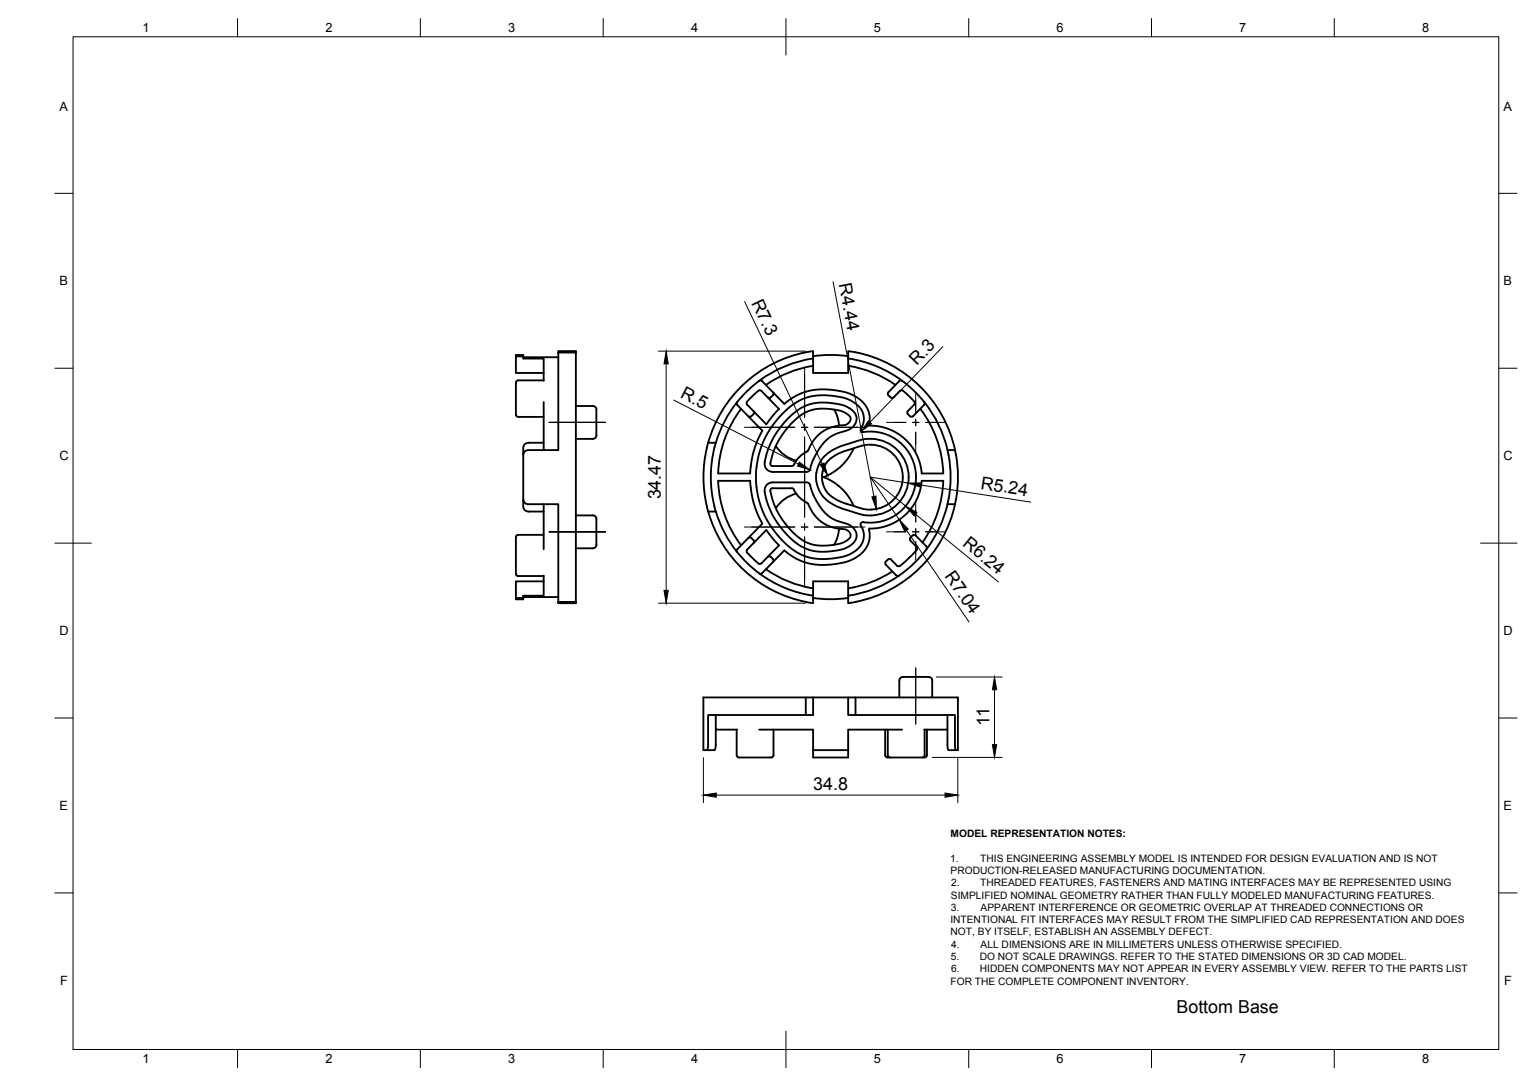
ISO-10303-21;
HEADER;
/* Generated by software containing ST-Developer
 * from STEP Tools, Inc. (www.steptools.com) 
 */

FILE_DESCRIPTION(
/* description */ ('STEP AP214'),
/* implementation_level */ '2;1');

FILE_NAME(
/* name */ 'Bottom Base.step',
/* time_stamp */ '2026-10-06T00:19:40-07:00',
/* author */ (''),
/* organization */ (''),
/* preprocessor_version */ 'ST-DEVELOPER v20.2',
/* originating_system */ 'Autodesk Translation Framework v15.15.0.0',
/* authorisation */ '');

FILE_SCHEMA (('AUTOMOTIVE_DESIGN { 1 0 10303 214 3 1 1 }'));
ENDSEC;

DATA;
#10=MECHANICAL_DESIGN_GEOMETRIC_PRESENTATION_REPRESENTATION('',(#2067),#98302);
#63=ORIENTED_CLOSED_SHELL('',*,#34171,.F.);
#64=ORIENTED_CLOSED_SHELL('',*,#34172,.F.);
#65=BREP_WITH_VOIDS('Body1',#34173,(#63,#64));
#120=TOROIDAL_SURFACE('',#35179,1.75,0.5);
#121=TOROIDAL_SURFACE('',#35197,1.75,0.5);
#122=TOROIDAL_SURFACE('',#35509,16.1,0.3);
#123=TOROIDAL_SURFACE('',#35537,0.6,0.3);
#124=TOROIDAL_SURFACE('',#35540,15.7,0.3);
#125=TOROIDAL_SURFACE('',#35542,0.6,0.3);
#126=TOROIDAL_SURFACE('',#35565,16.1,0.3);
#127=TOROIDAL_SURFACE('',#35593,0.6,0.3);
#128=TOROIDAL_SURFACE('',#35596,15.7,0.3);
#129=TOROIDAL_SURFACE('',#35598,0.6,0.3);
#130=TOROIDAL_SURFACE('',#35623,16.1,0.3);
#131=TOROIDAL_SURFACE('',#35651,0.6,0.3);
#132=TOROIDAL_SURFACE('',#35654,15.7,0.3);
#133=TOROIDAL_SURFACE('',#35656,0.6,0.3);
#134=TOROIDAL_SURFACE('',#35689,16.1,0.3);
#135=TOROIDAL_SURFACE('',#35706,0.6,0.3);
#136=TOROIDAL_SURFACE('',#35709,15.7,0.3);
#137=TOROIDAL_SURFACE('',#35711,0.6,0.3);
#587=ELLIPSE('',#35016,13.361638124116,11.5578357668316);
#588=ELLIPSE('',#35018,0.952789221356583,0.825051280209737);
#589=ELLIPSE('',#35164,8.5034308409691,7.3551645679647);
#590=ELLIPSE('',#35170,0.95278921998829,0.825051277838727);
#591=ELLIPSE('',#35172,13.3616381240247,11.5578357666725);
#592=ELLIPSE('',#35175,13.3641581201969,11.5586227277888);
#593=ELLIPSE('',#35177,13.3735436793885,11.5615411739172);
#594=ELLIPSE('',#35193,13.3735436794947,11.5615411741025);
#595=ELLIPSE('',#35195,13.3641581202021,11.5586227277978);
#596=ELLIPSE('',#35373,5.47251735374185,5.45746583056251);
#597=ELLIPSE('',#35374,5.47484463449433,5.45859738058976);
#598=ELLIPSE('',#35383,1586.78234781094,77.5099567232996);
#599=ELLIPSE('',#35385,1.14101622851481,0.979516364167449);
#600=ELLIPSE('',#35388,3.21318791213204,0.733552647206039);
#601=ELLIPSE('',#35393,9.5906032530047,5.82945480771065);
#602=ELLIPSE('',#35396,9.59060325044611,5.82945480684165);
#603=ELLIPSE('',#35401,1586.78234781094,77.5099567232996);
#604=ELLIPSE('',#35402,1.14101622838842,0.979516363971379);
#605=ELLIPSE('',#35405,3.21319255571472,0.733554698090194);
#712=SPHERICAL_SURFACE('',#35503,0.3);
#713=SPHERICAL_SURFACE('',#35507,0.3);
#714=SPHERICAL_SURFACE('',#35514,0.3);
#715=SPHERICAL_SURFACE('',#35522,0.3);
#716=SPHERICAL_SURFACE('',#35527,0.3);
#717=SPHERICAL_SURFACE('',#35532,0.3);
#718=SPHERICAL_SURFACE('',#35559,0.3);
#719=SPHERICAL_SURFACE('',#35563,0.3);
#720=SPHERICAL_SURFACE('',#35570,0.3);
#721=SPHERICAL_SURFACE('',#35578,0.3);
#722=SPHERICAL_SURFACE('',#35583,0.3);
#723=SPHERICAL_SURFACE('',#35588,0.3);
#724=SPHERICAL_SURFACE('',#35617,0.3);
#725=SPHERICAL_SURFACE('',#35621,0.3);
#726=SPHERICAL_SURFACE('',#35628,0.3);
#727=SPHERICAL_SURFACE('',#35636,0.3);
#728=SPHERICAL_SURFACE('',#35641,0.3);
#729=SPHERICAL_SURFACE('',#35646,0.3);
#730=SPHERICAL_SURFACE('',#35673,0.3);
#731=SPHERICAL_SURFACE('',#35677,0.3);
#732=SPHERICAL_SURFACE('',#35686,0.3);
#733=SPHERICAL_SURFACE('',#35691,0.3);
#734=SPHERICAL_SURFACE('',#35697,0.3);
#735=SPHERICAL_SURFACE('',#35700,0.3);
#1106=B_SPLINE_SURFACE_WITH_KNOTS('',3,1,((#74322,#74323),(#74324,#74325),
(#74326,#74327),(#74328,#74329)),.UNSPECIFIED.,.F.,.F.,.F.,(4,4),(2,2),
(1.93787056397,2.72108189072),(0.,0.18),.UNSPECIFIED.);
#1107=B_SPLINE_SURFACE_WITH_KNOTS('',3,1,((#74355,#74356),(#74357,#74358),
(#74359,#74360),(#74361,#74362)),.UNSPECIFIED.,.F.,.F.,.F.,(4,4),(2,2),
(1.93787056397,2.72108189072),(0.,0.18),.UNSPECIFIED.);
#1108=B_SPLINE_SURFACE_WITH_KNOTS('',4,1,((#74601,#74602),(#74603,#74604),
(#74605,#74606),(#74607,#74608),(#74609,#74610)),.UNSPECIFIED.,.F.,.F.,
 .F.,(5,5),(2,2),(13.4220086236,14.3963748612),(0.,0.288),.UNSPECIFIED.);
#1109=B_SPLINE_SURFACE_WITH_KNOTS('',4,1,((#74660,#74661),(#74662,#74663),
(#74664,#74665),(#74666,#74667),(#74668,#74669)),.UNSPECIFIED.,.F.,.F.,
 .F.,(5,5),(2,2),(13.4220086236,14.3963748612),(0.,0.288),.UNSPECIFIED.);
#1110=B_SPLINE_SURFACE_WITH_KNOTS('',4,1,((#74721,#74722),(#74723,#74724),
(#74725,#74726),(#74727,#74728),(#74729,#74730)),.UNSPECIFIED.,.F.,.F.,
 .F.,(5,5),(2,2),(7.90893025972,8.88329649724),(0.,0.288),.UNSPECIFIED.);
#1111=B_SPLINE_SURFACE_WITH_KNOTS('',4,1,((#74780,#74781),(#74782,#74783),
(#74784,#74785),(#74786,#74787),(#74788,#74789)),.UNSPECIFIED.,.F.,.F.,
 .F.,(5,5),(2,2),(7.90893025972,8.88329649724),(0.,0.288),.UNSPECIFIED.);
#1112=B_SPLINE_SURFACE_WITH_KNOTS('',5,1,((#75672,#75673),(#75674,#75675),
(#75676,#75677),(#75678,#75679),(#75680,#75681),(#75682,#75683),(#75684,
#75685),(#75686,#75687),(#75688,#75689),(#75690,#75691),(#75692,#75693),
(#75694,#75695)),.UNSPECIFIED.,.F.,.F.,.F.,(6,3,3,6),(2,2),(0.,3.06410506181,
5.01303018899,6.53082821197),(0.,0.180000000000001),.UNSPECIFIED.);
#1113=B_SPLINE_SURFACE_WITH_KNOTS('',5,1,((#75710,#75711),(#75712,#75713),
(#75714,#75715),(#75716,#75717),(#75718,#75719),(#75720,#75721),(#75722,
#75723),(#75724,#75725),(#75726,#75727),(#75728,#75729),(#75730,#75731),
(#75732,#75733)),.UNSPECIFIED.,.F.,.F.,.F.,(6,3,3,6),(2,2),(0.,1.23981126536,
4.14117682427,4.7101423031),(0.,0.180000000000001),.UNSPECIFIED.);
#1114=B_SPLINE_SURFACE_WITH_KNOTS('',5,1,((#75748,#75749),(#75750,#75751),
(#75752,#75753),(#75754,#75755),(#75756,#75757),(#75758,#75759),(#75760,
#75761),(#75762,#75763),(#75764,#75765),(#75766,#75767),(#75768,#75769),
(#75770,#75771)),.UNSPECIFIED.,.F.,.F.,.F.,(6,3,3,6),(2,2),(17.5092154859,
21.7374875265,29.3008927769,31.9433833551),(0.,0.180000000000001),
 .UNSPECIFIED.);
#1115=B_SPLINE_SURFACE_WITH_KNOTS('',5,1,((#75786,#75787),(#75788,#75789),
(#75790,#75791),(#75792,#75793),(#75794,#75795),(#75796,#75797),(#75798,
#75799),(#75800,#75801),(#75802,#75803)),.UNSPECIFIED.,.F.,.F.,.F.,(6,3,
6),(2,2),(10.4583103224,10.8525207074,15.6953714763),(0.,0.180000000000001),
 .UNSPECIFIED.);
#1116=B_SPLINE_SURFACE_WITH_KNOTS('',5,1,((#75836,#75837),(#75838,#75839),
(#75840,#75841),(#75842,#75843),(#75844,#75845),(#75846,#75847),(#75848,
#75849),(#75850,#75851),(#75852,#75853)),.UNSPECIFIED.,.F.,.F.,.F.,(6,3,
6),(2,2),(-1.52206773895,0.,8.40229743882),(0.,0.180000000000003),
 .UNSPECIFIED.);
#1117=B_SPLINE_SURFACE_WITH_KNOTS('',5,1,((#75877,#75878),(#75879,#75880),
(#75881,#75882),(#75883,#75884),(#75885,#75886),(#75887,#75888),(#75889,
#75890),(#75891,#75892),(#75893,#75894)),.UNSPECIFIED.,.F.,.F.,.F.,(6,3,
6),(2,2),(-1.52206773895,0.,8.40229791516),(0.,0.180000000000001),
 .UNSPECIFIED.);
#1118=B_SPLINE_SURFACE_WITH_KNOTS('',5,1,((#75906,#75907),(#75908,#75909),
(#75910,#75911),(#75912,#75913),(#75914,#75915),(#75916,#75917),(#75918,
#75919),(#75920,#75921),(#75922,#75923)),.UNSPECIFIED.,.F.,.F.,.F.,(6,3,
6),(2,2),(10.4583103224,10.8525207074,15.6953714763),(0.,0.180000000000001),
 .UNSPECIFIED.);
#1119=B_SPLINE_SURFACE_WITH_KNOTS('',5,1,((#75956,#75957),(#75958,#75959),
(#75960,#75961),(#75962,#75963),(#75964,#75965),(#75966,#75967),(#75968,
#75969),(#75970,#75971),(#75972,#75973),(#75974,#75975),(#75976,#75977),
(#75978,#75979)),.UNSPECIFIED.,.F.,.F.,.F.,(6,3,3,6),(2,2),(17.5092154859,
21.7374875265,29.3008927769,31.9433833551),(0.,0.180000000000001),
 .UNSPECIFIED.);
#1120=B_SPLINE_SURFACE_WITH_KNOTS('',5,1,((#75996,#75997),(#75998,#75999),
(#76000,#76001),(#76002,#76003),(#76004,#76005),(#76006,#76007),(#76008,
#76009),(#76010,#76011),(#76012,#76013),(#76014,#76015),(#76016,#76017),
(#76018,#76019)),.UNSPECIFIED.,.F.,.F.,.F.,(6,3,3,6),(2,2),(0.,1.23981126536,
4.14117682427,4.7101423031),(0.,0.180000000000001),.UNSPECIFIED.);
#1121=B_SPLINE_SURFACE_WITH_KNOTS('',5,1,((#76034,#76035),(#76036,#76037),
(#76038,#76039),(#76040,#76041),(#76042,#76043),(#76044,#76045),(#76046,
#76047),(#76048,#76049),(#76050,#76051),(#76052,#76053),(#76054,#76055),
(#76056,#76057)),.UNSPECIFIED.,.F.,.F.,.F.,(6,3,3,6),(2,2),(0.,3.06410506181,
5.01303018899,6.53082821197),(0.,0.180000000000001),.UNSPECIFIED.);
#1122=B_SPLINE_SURFACE_WITH_KNOTS('',5,1,((#76190,#76191),(#76192,#76193),
(#76194,#76195),(#76196,#76197),(#76198,#76199),(#76200,#76201),(#76202,
#76203),(#76204,#76205),(#76206,#76207),(#76208,#76209),(#76210,#76211),
(#76212,#76213),(#76214,#76215),(#76216,#76217),(#76218,#76219)),
 .UNSPECIFIED.,.F.,.F.,.F.,(6,3,3,3,6),(2,2),(0.,2.13949651284,3.65547289001,
4.94562974894,5.62440522293),(0.,0.120000000000001),.UNSPECIFIED.);
#1123=B_SPLINE_SURFACE_WITH_KNOTS('',5,1,((#76253,#76254),(#76255,#76256),
(#76257,#76258),(#76259,#76260),(#76261,#76262),(#76263,#76264),(#76265,
#76266),(#76267,#76268),(#76269,#76270)),.UNSPECIFIED.,.F.,.F.,.F.,(6,3,
6),(2,2),(0.,1.07297825382,3.85154891337),(0.,0.120000000000002),
 .UNSPECIFIED.);
#1124=B_SPLINE_SURFACE_WITH_KNOTS('',5,1,((#76292,#76293),(#76294,#76295),
(#76296,#76297),(#76298,#76299),(#76300,#76301),(#76302,#76303),(#76304,
#76305),(#76306,#76307),(#76308,#76309),(#76310,#76311),(#76312,#76313),
(#76314,#76315),(#76316,#76317),(#76318,#76319),(#76320,#76321),(#76322,
#76323),(#76324,#76325),(#76326,#76327)),.UNSPECIFIED.,.F.,.F.,.F.,(6,3,
3,3,3,6),(2,2),(-1.28529178055,0.,8.34825709363,17.7305069581,25.102843518,
27.4630296434),(0.,0.120000000000001),.UNSPECIFIED.);
#1125=B_SPLINE_SURFACE_WITH_KNOTS('',5,1,((#76373,#76374),(#76375,#76376),
(#76377,#76378),(#76379,#76380),(#76381,#76382),(#76383,#76384),(#76385,
#76386),(#76387,#76388),(#76389,#76390),(#76391,#76392),(#76393,#76394),
(#76395,#76396),(#76397,#76398),(#76399,#76400),(#76401,#76402),(#76403,
#76404),(#76405,#76406),(#76407,#76408)),.UNSPECIFIED.,.F.,.F.,.F.,(6,3,
3,3,3,6),(2,2),(-1.28529178055,0.,8.34825709363,17.7305069581,25.102843518,
27.4630296434),(0.,0.120000000000001),.UNSPECIFIED.);
#1126=B_SPLINE_SURFACE_WITH_KNOTS('',5,1,((#76448,#76449),(#76450,#76451),
(#76452,#76453),(#76454,#76455),(#76456,#76457),(#76458,#76459),(#76460,
#76461),(#76462,#76463),(#76464,#76465)),.UNSPECIFIED.,.F.,.F.,.F.,(6,3,
6),(2,2),(0.,1.07297825382,3.85154891337),(0.,0.120000000000001),
 .UNSPECIFIED.);
#1127=B_SPLINE_SURFACE_WITH_KNOTS('',5,1,((#76487,#76488),(#76489,#76490),
(#76491,#76492),(#76493,#76494),(#76495,#76496),(#76497,#76498),(#76499,
#76500),(#76501,#76502),(#76503,#76504),(#76505,#76506),(#76507,#76508),
(#76509,#76510),(#76511,#76512),(#76513,#76514),(#76515,#76516)),
 .UNSPECIFIED.,.F.,.F.,.F.,(6,3,3,3,6),(2,2),(0.,2.13949651284,3.65547289001,
4.94562974894,5.62440522293),(0.,0.120000000000001),.UNSPECIFIED.);
#1128=B_SPLINE_SURFACE_WITH_KNOTS('',5,1,((#76588,#76589),(#76590,#76591),
(#76592,#76593),(#76594,#76595),(#76596,#76597),(#76598,#76599)),
 .UNSPECIFIED.,.F.,.F.,.F.,(6,6),(2,2),(0.,3.5713550833),(0.,0.300000000000001),
 .UNSPECIFIED.);
#1129=B_SPLINE_SURFACE_WITH_KNOTS('',5,1,((#76666,#76667),(#76668,#76669),
(#76670,#76671),(#76672,#76673),(#76674,#76675),(#76676,#76677)),
 .UNSPECIFIED.,.F.,.F.,.F.,(6,6),(2,2),(0.,3.5713550833),(0.,0.300000000000001),
 .UNSPECIFIED.);
#1130=B_SPLINE_SURFACE_WITH_KNOTS('',5,1,((#77077,#77078),(#77079,#77080),
(#77081,#77082),(#77083,#77084),(#77085,#77086),(#77087,#77088),(#77089,
#77090),(#77091,#77092),(#77093,#77094),(#77095,#77096),(#77097,#77098),
(#77099,#77100),(#77101,#77102),(#77103,#77104),(#77105,#77106),(#77107,
#77108),(#77109,#77110),(#77111,#77112)),.UNSPECIFIED.,.F.,.F.,.F.,(6,3,
3,3,3,6),(2,2),(2.04066423734,2.62011481805,3.50908168923,4.52495007124,
5.25002578886,6.51367347233),(0.,0.300000000000002),.UNSPECIFIED.);
#1131=B_SPLINE_SURFACE_WITH_KNOTS('',5,1,((#77218,#77219),(#77220,#77221),
(#77222,#77223),(#77224,#77225),(#77226,#77227),(#77228,#77229),(#77230,
#77231),(#77232,#77233),(#77234,#77235),(#77236,#77237),(#77238,#77239),
(#77240,#77241),(#77242,#77243),(#77244,#77245),(#77246,#77247),(#77248,
#77249),(#77250,#77251),(#77252,#77253)),.UNSPECIFIED.,.F.,.F.,.F.,(6,3,
3,3,3,6),(2,2),(2.04066423734,2.62011481805,3.50908168923,4.52495007124,
5.25002578886,6.51367347233),(0.,0.300000000000002),.UNSPECIFIED.);
#1132=B_SPLINE_SURFACE_WITH_KNOTS('',5,1,((#77254,#77255),(#77256,#77257),
(#77258,#77259),(#77260,#77261),(#77262,#77263),(#77264,#77265),(#77266,
#77267),(#77268,#77269),(#77270,#77271),(#77272,#77273),(#77274,#77275),
(#77276,#77277)),.UNSPECIFIED.,.F.,.F.,.F.,(6,3,3,6),(2,2),(0.,3.39713474113,
6.68643994484,8.37826425912),(0.,0.300000000000001),.UNSPECIFIED.);
#1133=B_SPLINE_SURFACE_WITH_KNOTS('',5,1,((#77298,#77299),(#77300,#77301),
(#77302,#77303),(#77304,#77305),(#77306,#77307),(#77308,#77309),(#77310,
#77311),(#77312,#77313),(#77314,#77315)),.UNSPECIFIED.,.F.,.F.,.F.,(6,3,
6),(2,2),(0.,2.6134611976,3.73613338933),(0.,0.300000000000001),
 .UNSPECIFIED.);
#1134=B_SPLINE_SURFACE_WITH_KNOTS('',5,1,((#77327,#77328),(#77329,#77330),
(#77331,#77332),(#77333,#77334),(#77335,#77336),(#77337,#77338)),
 .UNSPECIFIED.,.F.,.F.,.F.,(6,6),(2,2),(0.,1.1155886229),(0.,0.300000000000001),
 .UNSPECIFIED.);
#1135=B_SPLINE_SURFACE_WITH_KNOTS('',5,1,((#77347,#77348),(#77349,#77350),
(#77351,#77352),(#77353,#77354),(#77355,#77356),(#77357,#77358),(#77359,
#77360),(#77361,#77362),(#77363,#77364),(#77365,#77366),(#77367,#77368),
(#77369,#77370),(#77371,#77372),(#77373,#77374),(#77375,#77376)),
 .UNSPECIFIED.,.F.,.F.,.F.,(6,3,3,3,6),(2,2),(0.,1.14196741734,1.69664449439,
2.26600465298,2.82383165251),(0.,0.300000000000001),.UNSPECIFIED.);
#1136=B_SPLINE_SURFACE_WITH_KNOTS('',5,1,((#77394,#77395),(#77396,#77397),
(#77398,#77399),(#77400,#77401),(#77402,#77403),(#77404,#77405)),
 .UNSPECIFIED.,.F.,.F.,.F.,(6,6),(2,2),(0.,2.29845936737),(0.,0.300000000000001),
 .UNSPECIFIED.);
#1137=B_SPLINE_SURFACE_WITH_KNOTS('',5,1,((#77414,#77415),(#77416,#77417),
(#77418,#77419),(#77420,#77421),(#77422,#77423),(#77424,#77425),(#77426,
#77427),(#77428,#77429),(#77430,#77431),(#77432,#77433),(#77434,#77435),
(#77436,#77437),(#77438,#77439),(#77440,#77441),(#77442,#77443)),
 .UNSPECIFIED.,.F.,.F.,.F.,(6,3,3,3,6),(2,2),(0.,6.696077534,12.6191089245,
16.7682744334,17.9215041098),(0.,0.300000000000001),.UNSPECIFIED.);
#1138=B_SPLINE_SURFACE_WITH_KNOTS('',5,1,((#77471,#77472),(#77473,#77474),
(#77475,#77476),(#77477,#77478),(#77479,#77480),(#77481,#77482),(#77483,
#77484),(#77485,#77486),(#77487,#77488),(#77489,#77490),(#77491,#77492),
(#77493,#77494),(#77495,#77496),(#77497,#77498),(#77499,#77500)),
 .UNSPECIFIED.,.F.,.F.,.F.,(6,3,3,3,6),(2,2),(0.,6.696077534,12.6191089245,
16.7682744334,17.9215041098),(0.,0.300000000000001),.UNSPECIFIED.);
#1139=B_SPLINE_SURFACE_WITH_KNOTS('',5,1,((#77520,#77521),(#77522,#77523),
(#77524,#77525),(#77526,#77527),(#77528,#77529),(#77530,#77531),(#77532,
#77533),(#77534,#77535),(#77536,#77537)),.UNSPECIFIED.,.F.,.F.,.F.,(6,3,
6),(2,2),(0.,2.6134611976,3.73613338933),(0.,0.300000000000001),
 .UNSPECIFIED.);
#1140=B_SPLINE_SURFACE_WITH_KNOTS('',5,1,((#77565,#77566),(#77567,#77568),
(#77569,#77570),(#77571,#77572),(#77573,#77574),(#77575,#77576),(#77577,
#77578),(#77579,#77580),(#77581,#77582),(#77583,#77584),(#77585,#77586),
(#77587,#77588)),.UNSPECIFIED.,.F.,.F.,.F.,(6,3,3,6),(2,2),(0.,3.39713474113,
6.68643994484,8.37826425912),(0.,0.300000000000001),.UNSPECIFIED.);
#1141=B_SPLINE_SURFACE_WITH_KNOTS('',5,1,((#77603,#77604),(#77605,#77606),
(#77607,#77608),(#77609,#77610),(#77611,#77612),(#77613,#77614)),
 .UNSPECIFIED.,.F.,.F.,.F.,(6,6),(2,2),(0.,2.29845936737),(0.,0.300000000000001),
 .UNSPECIFIED.);
#1142=B_SPLINE_SURFACE_WITH_KNOTS('',5,1,((#77623,#77624),(#77625,#77626),
(#77627,#77628),(#77629,#77630),(#77631,#77632),(#77633,#77634),(#77635,
#77636),(#77637,#77638),(#77639,#77640),(#77641,#77642),(#77643,#77644),
(#77645,#77646),(#77647,#77648),(#77649,#77650),(#77651,#77652)),
 .UNSPECIFIED.,.F.,.F.,.F.,(6,3,3,3,6),(2,2),(0.,1.14196741734,1.69664449439,
2.26600465298,2.82383165251),(0.,0.300000000000001),.UNSPECIFIED.);
#1143=B_SPLINE_SURFACE_WITH_KNOTS('',5,1,((#77670,#77671),(#77672,#77673),
(#77674,#77675),(#77676,#77677),(#77678,#77679),(#77680,#77681)),
 .UNSPECIFIED.,.F.,.F.,.F.,(6,6),(2,2),(0.,1.1155886229),(0.,0.300000000000001),
 .UNSPECIFIED.);
#1144=B_SPLINE_SURFACE_WITH_KNOTS('',5,1,((#77688,#77689),(#77690,#77691),
(#77692,#77693),(#77694,#77695),(#77696,#77697),(#77698,#77699),(#77700,
#77701),(#77702,#77703),(#77704,#77705),(#77706,#77707),(#77708,#77709),
(#77710,#77711),(#77712,#77713),(#77714,#77715),(#77716,#77717)),
 .UNSPECIFIED.,.F.,.F.,.F.,(6,3,3,3,6),(2,2),(0.,1.06902836413,2.19771269917,
3.2241260379,4.7004853448),(0.,0.120000000000001),.UNSPECIFIED.);
#1145=B_SPLINE_SURFACE_WITH_KNOTS('',5,1,((#77737,#77738),(#77739,#77740),
(#77741,#77742),(#77743,#77744),(#77745,#77746),(#77747,#77748)),
 .UNSPECIFIED.,.F.,.F.,.F.,(6,6),(2,2),(0.,6.43612007405),(0.,0.120000000000001),
 .UNSPECIFIED.);
#1146=B_SPLINE_SURFACE_WITH_KNOTS('',5,1,((#77777,#77778),(#77779,#77780),
(#77781,#77782),(#77783,#77784),(#77785,#77786),(#77787,#77788),(#77789,
#77790),(#77791,#77792),(#77793,#77794),(#77795,#77796),(#77797,#77798),
(#77799,#77800),(#77801,#77802),(#77803,#77804),(#77805,#77806)),
 .UNSPECIFIED.,.F.,.F.,.F.,(6,3,3,3,6),(2,2),(0.039515807079,7.53253625942,
14.2747183071,18.8083875826,22.71906151),(0.,0.120000000000001),
 .UNSPECIFIED.);
#1147=B_SPLINE_SURFACE_WITH_KNOTS('',5,1,((#77824,#77825),(#77826,#77827),
(#77828,#77829),(#77830,#77831),(#77832,#77833),(#77834,#77835),(#77836,
#77837),(#77838,#77839),(#77840,#77841)),.UNSPECIFIED.,.F.,.F.,.F.,(6,3,
6),(2,2),(1.18944404077E-12,1.10170421198,3.01229896543),(0.,0.120000000000001),
 .UNSPECIFIED.);
#1148=B_SPLINE_SURFACE_WITH_KNOTS('',5,1,((#77851,#77852),(#77853,#77854),
(#77855,#77856),(#77857,#77858),(#77859,#77860),(#77861,#77862),(#77863,
#77864),(#77865,#77866),(#77867,#77868)),.UNSPECIFIED.,.F.,.F.,.F.,(6,3,
6),(2,2),(0.,2.92723336323,3.88093368919),(0.,0.120000000000002),
 .UNSPECIFIED.);
#1149=B_SPLINE_SURFACE_WITH_KNOTS('',5,1,((#77871,#77872),(#77873,#77874),
(#77875,#77876),(#77877,#77878),(#77879,#77880),(#77881,#77882),(#77883,
#77884),(#77885,#77886),(#77887,#77888),(#77889,#77890),(#77891,#77892),
(#77893,#77894),(#77895,#77896),(#77897,#77898),(#77899,#77900),(#77901,
#77902),(#77903,#77904)),.UNSPECIFIED.,.F.,.F.,.F.,(6,3,3,5,6),(2,2),(3.11522256756,
4.13897763214,6.99130562041,9.89933117719,9.89969814681689),(0.,0.120000000000001),
 .UNSPECIFIED.);
#1150=B_SPLINE_SURFACE_WITH_KNOTS('',5,1,((#77908,#77909),(#77910,#77911),
(#77912,#77913),(#77914,#77915),(#77916,#77917),(#77918,#77919),(#77920,
#77921),(#77922,#77923),(#77924,#77925),(#77926,#77927),(#77928,#77929),
(#77930,#77931)),.UNSPECIFIED.,.F.,.F.,.F.,(6,3,3,6),(2,2),(3.11522256756,
4.13897763214,6.99130562041,9.89912618426),(0.,0.120000000000001),
 .UNSPECIFIED.);
#1151=B_SPLINE_SURFACE_WITH_KNOTS('',5,1,((#77933,#77934),(#77935,#77936),
(#77937,#77938),(#77939,#77940),(#77941,#77942),(#77943,#77944),(#77945,
#77946),(#77947,#77948),(#77949,#77950),(#77951,#77952),(#77953,#77954),
(#77955,#77956),(#77957,#77958),(#77959,#77960)),.UNSPECIFIED.,.F.,.F.,
 .F.,(6,3,5,6),(2,2),(0.,2.92723336323,3.88093368919,3.88140412218319),
(0.,0.120000000000005),.UNSPECIFIED.);
#1152=B_SPLINE_SURFACE_WITH_KNOTS('',5,1,((#77987,#77988),(#77989,#77990),
(#77991,#77992),(#77993,#77994),(#77995,#77996),(#77997,#77998)),
 .UNSPECIFIED.,.F.,.F.,.F.,(6,6),(2,2),(0.,6.43612007405),(0.,0.120000000000003),
 .UNSPECIFIED.);
#1153=B_SPLINE_SURFACE_WITH_KNOTS('',5,1,((#78007,#78008),(#78009,#78010),
(#78011,#78012),(#78013,#78014),(#78015,#78016),(#78017,#78018),(#78019,
#78020),(#78021,#78022),(#78023,#78024),(#78025,#78026),(#78027,#78028),
(#78029,#78030),(#78031,#78032),(#78033,#78034),(#78035,#78036)),
 .UNSPECIFIED.,.F.,.F.,.F.,(6,3,3,3,6),(2,2),(0.,1.06902836413,2.19771269917,
3.2241260379,4.7004853448),(0.,0.120000000000001),.UNSPECIFIED.);
#1154=B_SPLINE_SURFACE_WITH_KNOTS('',5,1,((#78054,#78055),(#78056,#78057),
(#78058,#78059),(#78060,#78061),(#78062,#78063),(#78064,#78065),(#78066,
#78067),(#78068,#78069),(#78070,#78071)),.UNSPECIFIED.,.F.,.F.,.F.,(6,3,
6),(2,2),(1.18944404077E-12,1.10170421198,3.01229896543),(0.,0.120000000000001),
 .UNSPECIFIED.);
#1155=B_SPLINE_SURFACE_WITH_KNOTS('',5,1,((#78083,#78084),(#78085,#78086),
(#78087,#78088),(#78089,#78090),(#78091,#78092),(#78093,#78094),(#78095,
#78096),(#78097,#78098),(#78099,#78100),(#78101,#78102),(#78103,#78104),
(#78105,#78106),(#78107,#78108),(#78109,#78110),(#78111,#78112)),
 .UNSPECIFIED.,.F.,.F.,.F.,(6,3,3,3,6),(2,2),(0.0395158070789,7.53253625942,
14.2747183071,18.8083875826,22.71906151),(0.,0.120000000000001),
 .UNSPECIFIED.);
#1274=FACE_BOUND('',#5903,.T.);
#1275=FACE_BOUND('',#5904,.T.);
#1276=FACE_BOUND('',#5905,.T.);
#1277=FACE_BOUND('',#5906,.T.);
#1278=FACE_BOUND('',#5907,.T.);
#1279=FACE_BOUND('',#5908,.T.);
#1280=FACE_BOUND('',#6001,.T.);
#1281=FACE_BOUND('',#6002,.T.);
#1282=FACE_BOUND('',#6003,.T.);
#1283=FACE_BOUND('',#6038,.T.);
#1284=FACE_BOUND('',#6051,.T.);
#1285=FACE_BOUND('',#6070,.T.);
#1286=FACE_BOUND('',#6072,.T.);
#1287=FACE_BOUND('',#6074,.T.);
#1288=FACE_BOUND('',#6114,.T.);
#1289=FACE_BOUND('',#6115,.T.);
#1290=FACE_BOUND('',#6116,.T.);
#1291=FACE_BOUND('',#6121,.T.);
#1292=FACE_BOUND('',#6170,.T.);
#1293=FACE_BOUND('',#6172,.T.);
#1294=FACE_BOUND('',#6188,.T.);
#1636=B_SPLINE_CURVE_WITH_KNOTS('',3,(#74305,#74306,#74307,#74308),
 .UNSPECIFIED.,.F.,.F.,(4,4),(1.93787056397,2.72108189072),
 .UNSPECIFIED.);
#1637=B_SPLINE_CURVE_WITH_KNOTS('',3,(#74330,#74331,#74332,#74333),
 .UNSPECIFIED.,.F.,.F.,(4,4),(1.93787056397,2.72108189072),
 .UNSPECIFIED.);
#1638=B_SPLINE_CURVE_WITH_KNOTS('',3,(#74338,#74339,#74340,#74341),
 .UNSPECIFIED.,.F.,.F.,(4,4),(1.93787056397,2.72108189072),
 .UNSPECIFIED.);
#1639=B_SPLINE_CURVE_WITH_KNOTS('',3,(#74363,#74364,#74365,#74366),
 .UNSPECIFIED.,.F.,.F.,(4,4),(1.93787056397,2.72108189072),
 .UNSPECIFIED.);
#1640=B_SPLINE_CURVE_WITH_KNOTS('',4,(#74404,#74405,#74406,#74407,#74408),
 .UNSPECIFIED.,.F.,.F.,(5,5),(0.,1.),.UNSPECIFIED.);
#1641=B_SPLINE_CURVE_WITH_KNOTS('',4,(#74416,#74417,#74418,#74419,#74420),
 .UNSPECIFIED.,.F.,.F.,(5,5),(7.90893025972,8.88329649724),
 .UNSPECIFIED.);
#1642=B_SPLINE_CURVE_WITH_KNOTS('',4,(#74428,#74429,#74430,#74431,#74432),
 .UNSPECIFIED.,.F.,.F.,(5,5),(13.4220086236,14.3963748612),
 .UNSPECIFIED.);
#1643=B_SPLINE_CURVE_WITH_KNOTS('',4,(#74440,#74441,#74442,#74443,#74444),
 .UNSPECIFIED.,.F.,.F.,(5,5),(13.4220086236,14.3963748612),
 .UNSPECIFIED.);
#1644=B_SPLINE_CURVE_WITH_KNOTS('',5,(#74544,#74545,#74546,#74547,#74548,
#74549),.UNSPECIFIED.,.F.,.F.,(6,6),(1.465995819,7.32028714189),
 .UNSPECIFIED.);
#1645=B_SPLINE_CURVE_WITH_KNOTS('',4,(#74613,#74614,#74615,#74616,#74617),
 .UNSPECIFIED.,.F.,.F.,(5,5),(13.4220086236,14.3963748612),
 .UNSPECIFIED.);
#1646=B_SPLINE_CURVE_WITH_KNOTS('',3,(#74630,#74631,#74632,#74633,#74634,
#74635,#74636,#74637,#74638,#74639),.UNSPECIFIED.,.F.,.F.,(4,2,2,2,4),(-0.319033797120111,
-0.292165211589356,-0.265296626058601,-0.238938061557758,-0.212579497056914),
 .UNSPECIFIED.);
#1647=B_SPLINE_CURVE_WITH_KNOTS('',3,(#74643,#74644,#74645,#74646,#74647,
#74648,#74649,#74650,#74651,#74652),.UNSPECIFIED.,.F.,.F.,(4,2,2,2,4),(-0.425158994113829,
-0.398800429612985,-0.372441865112142,-0.345573279581387,-0.318704694050632),
 .UNSPECIFIED.);
#1648=B_SPLINE_CURVE_WITH_KNOTS('',4,(#74672,#74673,#74674,#74675,#74676),
 .UNSPECIFIED.,.F.,.F.,(5,5),(13.4220086236,14.3963748612),
 .UNSPECIFIED.);
#1649=B_SPLINE_CURVE_WITH_KNOTS('',4,(#74733,#74734,#74735,#74736,#74737),
 .UNSPECIFIED.,.F.,.F.,(5,5),(7.90893025972,8.88329649724),
 .UNSPECIFIED.);
#1650=B_SPLINE_CURVE_WITH_KNOTS('',3,(#74750,#74751,#74752,#74753,#74754,
#74755,#74756,#74757,#74758,#74759),.UNSPECIFIED.,.F.,.F.,(4,2,2,2,4),(-0.107173137775093,
-0.0799325798318727,-0.0526920218886528,-0.0263460109443264,0.),
 .UNSPECIFIED.);
#1651=B_SPLINE_CURVE_WITH_KNOTS('',3,(#74763,#74764,#74765,#74766,#74767,
#74768,#74769,#74770,#74771,#74772),.UNSPECIFIED.,.F.,.F.,(4,2,2,2,4),(-0.213889101174212,
-0.187543090229885,-0.161197079285559,-0.133956521342339,-0.106715963399119),
 .UNSPECIFIED.);
#1652=B_SPLINE_CURVE_WITH_KNOTS('',4,(#74791,#74792,#74793,#74794,#74795),
 .UNSPECIFIED.,.F.,.F.,(5,5),(7.90893025972,8.88329649724),
 .UNSPECIFIED.);
#1653=B_SPLINE_CURVE_WITH_KNOTS('',3,(#75099,#75100,#75101,#75102,#75103,
#75104,#75105,#75106,#75107,#75108),.UNSPECIFIED.,.F.,.F.,(4,2,2,2,4),(-0.321679119149099,
-0.294322680562913,-0.266966241976726,-0.24062267379048,-0.214279105604234),
 .UNSPECIFIED.);
#1654=B_SPLINE_CURVE_WITH_KNOTS('',3,(#75110,#75111,#75112,#75113,#75114,
#75115,#75116,#75117,#75118,#75119),.UNSPECIFIED.,.F.,.F.,(4,2,2,2,4),(0.321158197663602,
0.348514636249788,0.375871074835975,0.402214643022221,0.428558211208467),
 .UNSPECIFIED.);
#1655=B_SPLINE_CURVE_WITH_KNOTS('',5,(#75123,#75124,#75125,#75126,#75127,
#75128),.UNSPECIFIED.,.F.,.F.,(6,6),(148.878135266,165.903598687),
 .UNSPECIFIED.);
#1656=B_SPLINE_CURVE_WITH_KNOTS('',5,(#75131,#75132,#75133,#75134,#75135,
#75136),.UNSPECIFIED.,.F.,.F.,(6,6),(0.,2.27905325485),.UNSPECIFIED.);
#1657=B_SPLINE_CURVE_WITH_KNOTS('',5,(#75139,#75140,#75141,#75142,#75143,
#75144),.UNSPECIFIED.,.F.,.F.,(6,6),(0.,2.27905325485),.UNSPECIFIED.);
#1658=B_SPLINE_CURVE_WITH_KNOTS('',5,(#75147,#75148,#75149,#75150,#75151,
#75152),.UNSPECIFIED.,.F.,.F.,(6,6),(124.379562504,141.405025925),
 .UNSPECIFIED.);
#1659=B_SPLINE_CURVE_WITH_KNOTS('',4,(#75156,#75157,#75158,#75159,#75160),
 .UNSPECIFIED.,.F.,.F.,(5,5),(4.11843680488,6.1261056745),.UNSPECIFIED.);
#1660=B_SPLINE_CURVE_WITH_KNOTS('',4,(#75164,#75165,#75166,#75167,#75168),
 .UNSPECIFIED.,.F.,.F.,(5,5),(2.04203522484,4.04970409445),
 .UNSPECIFIED.);
#1661=B_SPLINE_CURVE_WITH_KNOTS('',5,(#75173,#75174,#75175,#75176,#75177,
#75178),.UNSPECIFIED.,.F.,.F.,(6,6),(1.465995819,7.32028714189),
 .UNSPECIFIED.);
#1662=B_SPLINE_CURVE_WITH_KNOTS('',3,(#75231,#75232,#75233,#75234,#75235,
#75236,#75237,#75238,#75239,#75240),.UNSPECIFIED.,.F.,.F.,(4,2,2,2,4),(-0.106582101769708,
-0.0796485655513957,-0.0527150293330838,-0.0263575146665419,0.),
 .UNSPECIFIED.);
#1663=B_SPLINE_CURVE_WITH_KNOTS('',3,(#75244,#75245,#75246,#75247,#75248,
#75249,#75250,#75251,#75252,#75253),.UNSPECIFIED.,.F.,.F.,(4,2,2,2,4),(0.212791235802262,
0.239148750468804,0.265506265135346,0.292439801353658,0.31937333757197),
 .UNSPECIFIED.);
#1664=B_SPLINE_CURVE_WITH_KNOTS('',5,(#75314,#75315,#75316,#75317,#75318,
#75319,#75320,#75321,#75322),.UNSPECIFIED.,.F.,.F.,(6,3,6),(-1.52206773895,
0.,8.40229708781167),.UNSPECIFIED.);
#1665=B_SPLINE_CURVE_WITH_KNOTS('',3,(#75337,#75338,#75339,#75340,#75341,
#75342,#75343,#75344,#75345,#75346,#75347,#75348,#75349,#75350,#75351,#75352,
#75353,#75354,#75355,#75356,#75357,#75358,#75359,#75360,#75361,#75362,#75363,
#75364),.UNSPECIFIED.,.F.,.F.,(4,3,3,3,3,3,3,3,3,4),(-0.271480002345994,
-0.251044878779879,-0.221887843336835,-0.191803254069106,-0.161041040318657,
-0.129499206095465,-0.096441307247811,-0.0623399505509545,-0.0260590387577341,
-3.17944058136899E-7),.UNSPECIFIED.);
#1666=B_SPLINE_CURVE_WITH_KNOTS('',5,(#75402,#75403,#75404,#75405,#75406,
#75407,#75408,#75409,#75410,#75411,#75412,#75413),.UNSPECIFIED.,.F.,.F.,
(6,3,3,6),(0.,0.469175571973241,0.767594863359273,1.),.UNSPECIFIED.);
#1667=B_SPLINE_CURVE_WITH_KNOTS('',5,(#75415,#75416,#75417,#75418,#75419,
#75420,#75421,#75422,#75423,#75424,#75425,#75426),.UNSPECIFIED.,.F.,.F.,
(6,3,3,6),(0.,1.23981126536,4.14117682427,4.7101423031),.UNSPECIFIED.);
#1668=B_SPLINE_CURVE_WITH_KNOTS('',5,(#75427,#75428,#75429,#75430,#75431,
#75432,#75433,#75434,#75435,#75436,#75437,#75438),.UNSPECIFIED.,.F.,.F.,
(6,3,3,6),(0.,0.292934935973857,0.816928097127191,1.),.UNSPECIFIED.);
#1669=B_SPLINE_CURVE_WITH_KNOTS('',5,(#75496,#75497,#75498,#75499,#75500,
#75501,#75502,#75503,#75504),.UNSPECIFIED.,.F.,.F.,(6,3,6),(-1.52206773895,
0.,8.40229708780905),.UNSPECIFIED.);
#1670=B_SPLINE_CURVE_WITH_KNOTS('',3,(#75515,#75516,#75517,#75518,#75519,
#75520,#75521,#75522,#75523,#75524,#75525,#75526,#75527,#75528,#75529,#75530,
#75531,#75532,#75533,#75534,#75535,#75536,#75537,#75538,#75539,#75540,#75541,
#75542),.UNSPECIFIED.,.F.,.F.,(4,3,3,3,3,3,3,3,3,4),(-0.271480014742483,
-0.251044890243242,-0.221887853468803,-0.191803262827329,-0.161041047672182,
-0.129499212008716,-0.0964413116515472,-0.0623399533975151,-0.0260590399476091,
-3.17944058081387E-7),.UNSPECIFIED.);
#1671=B_SPLINE_CURVE_WITH_KNOTS('',5,(#75558,#75559,#75560,#75561,#75562,
#75563,#75564,#75565,#75566,#75567,#75568,#75569),.UNSPECIFIED.,.F.,.F.,
(6,3,3,6),(17.5092154859,21.7374875265,29.3008927769,31.9433833551),
 .UNSPECIFIED.);
#1672=B_SPLINE_CURVE_WITH_KNOTS('',5,(#75571,#75572,#75573,#75574,#75575,
#75576,#75577,#75578,#75579,#75580,#75581,#75582),.UNSPECIFIED.,.F.,.F.,
(6,3,3,6),(0.,0.263221615309587,0.879204184880883,1.),.UNSPECIFIED.);
#1673=B_SPLINE_CURVE_WITH_KNOTS('',5,(#75584,#75585,#75586,#75587,#75588,
#75589,#75590,#75591,#75592,#75593,#75594,#75595),.UNSPECIFIED.,.F.,.F.,
(6,3,3,6),(0.,3.06410506181,5.01303018899,6.53082821197),.UNSPECIFIED.);
#1674=B_SPLINE_CURVE_WITH_KNOTS('',5,(#75698,#75699,#75700,#75701,#75702,
#75703,#75704,#75705,#75706,#75707,#75708,#75709),.UNSPECIFIED.,.F.,.F.,
(6,3,3,6),(0.,3.06410506181,5.01303018899,6.53082821197),.UNSPECIFIED.);
#1675=B_SPLINE_CURVE_WITH_KNOTS('',5,(#75735,#75736,#75737,#75738,#75739,
#75740,#75741,#75742,#75743,#75744,#75745,#75746),.UNSPECIFIED.,.F.,.F.,
(6,3,3,6),(0.,0.263221615309587,0.879204184880883,1.),.UNSPECIFIED.);
#1676=B_SPLINE_CURVE_WITH_KNOTS('',5,(#75773,#75774,#75775,#75776,#75777,
#75778,#75779,#75780,#75781,#75782,#75783,#75784),.UNSPECIFIED.,.F.,.F.,
(6,3,3,6),(17.5092154859,21.7374875265,29.3008927769,31.9433833551),
 .UNSPECIFIED.);
#1677=B_SPLINE_CURVE_WITH_KNOTS('',3,(#75807,#75808,#75809,#75810,#75811,
#75812,#75813,#75814,#75815,#75816,#75817,#75818,#75819,#75820,#75821,#75822,
#75823,#75824,#75825,#75826,#75827,#75828,#75829,#75830,#75831,#75832,#75833,
#75834),.UNSPECIFIED.,.F.,.F.,(4,3,3,3,3,3,3,3,3,4),(-0.271480015020472,
-0.251044890500306,-0.221887853696004,-0.191803263023729,-0.161041047837091,
-0.129499212141309,-0.0964413117502902,-0.0623399534613448,-0.0260590399743052,
-3.17944058358943E-7),.UNSPECIFIED.);
#1678=B_SPLINE_CURVE_WITH_KNOTS('',5,(#75856,#75857,#75858,#75859,#75860,
#75861,#75862,#75863,#75864),.UNSPECIFIED.,.F.,.F.,(6,3,6),(-1.52206773895,
0.,8.40229708781167),.UNSPECIFIED.);
#1679=B_SPLINE_CURVE_WITH_KNOTS('',5,(#75897,#75898,#75899,#75900,#75901,
#75902,#75903,#75904,#75905),.UNSPECIFIED.,.F.,.F.,(6,3,6),(-1.52206773895,
0.,8.40229708780905),.UNSPECIFIED.);
#1680=B_SPLINE_CURVE_WITH_KNOTS('',3,(#75928,#75929,#75930,#75931,#75932,
#75933,#75934,#75935,#75936,#75937,#75938,#75939,#75940,#75941,#75942,#75943,
#75944,#75945,#75946,#75947,#75948,#75949,#75950,#75951,#75952,#75953,#75954,
#75955),.UNSPECIFIED.,.F.,.F.,(4,3,3,3,3,3,3,3,3,4),(-0.271480002344046,
-0.251044878778074,-0.221887843335248,-0.191803254067733,-0.161041040317497,
-0.129499206094535,-0.0964413072471161,-0.0623399505504905,-0.0260590387575272,
-3.17944058136899E-7),.UNSPECIFIED.);
#1681=B_SPLINE_CURVE_WITH_KNOTS('',5,(#75983,#75984,#75985,#75986,#75987,
#75988,#75989,#75990,#75991,#75992,#75993,#75994),.UNSPECIFIED.,.F.,.F.,
(6,3,3,6),(0.,0.292934935973857,0.816928097127191,1.),.UNSPECIFIED.);
#1682=B_SPLINE_CURVE_WITH_KNOTS('',5,(#76022,#76023,#76024,#76025,#76026,
#76027,#76028,#76029,#76030,#76031,#76032,#76033),.UNSPECIFIED.,.F.,.F.,
(6,3,3,6),(0.,1.23981126536,4.14117682427,4.7101423031),.UNSPECIFIED.);
#1683=B_SPLINE_CURVE_WITH_KNOTS('',5,(#76059,#76060,#76061,#76062,#76063,
#76064,#76065,#76066,#76067,#76068,#76069,#76070),.UNSPECIFIED.,.F.,.F.,
(6,3,3,6),(0.,3.06410506181,5.01303018899,6.53082821197),.UNSPECIFIED.);
#1684=B_SPLINE_CURVE_WITH_KNOTS('',5,(#76115,#76116,#76117,#76118,#76119,
#76120),.UNSPECIFIED.,.F.,.F.,(6,6),(0.,1.),.UNSPECIFIED.);
#1685=B_SPLINE_CURVE_WITH_KNOTS('',5,(#76221,#76222,#76223,#76224,#76225,
#76226,#76227,#76228,#76229,#76230,#76231,#76232,#76233,#76234,#76235),
 .UNSPECIFIED.,.F.,.F.,(6,3,3,3,6),(0.,2.13949651284,3.65547289001,4.94562974894,
5.62440522293),.UNSPECIFIED.);
#1686=B_SPLINE_CURVE_WITH_KNOTS('',5,(#76238,#76239,#76240,#76241,#76242,
#76243,#76244,#76245,#76246,#76247,#76248,#76249,#76250,#76251,#76252),
 .UNSPECIFIED.,.F.,.F.,(6,3,3,3,6),(0.,2.13949651284,3.65547289001,4.94562974894,
5.62440522293),.UNSPECIFIED.);
#1687=B_SPLINE_CURVE_WITH_KNOTS('',5,(#76274,#76275,#76276,#76277,#76278,
#76279,#76280,#76281,#76282),.UNSPECIFIED.,.F.,.F.,(6,3,6),(0.,1.07297825382,
3.85154891337),.UNSPECIFIED.);
#1688=B_SPLINE_CURVE_WITH_KNOTS('',5,(#76283,#76284,#76285,#76286,#76287,
#76288,#76289,#76290,#76291),.UNSPECIFIED.,.F.,.F.,(6,3,6),(0.,0.278583571948246,
1.),.UNSPECIFIED.);
#1689=B_SPLINE_CURVE_WITH_KNOTS('',5,(#76329,#76330,#76331,#76332,#76333,
#76334,#76335,#76336,#76337,#76338,#76339,#76340,#76341,#76342,#76343,#76344,
#76345,#76346),.UNSPECIFIED.,.F.,.F.,(6,3,3,3,3,6),(-1.28529177837993,0.,
8.34825709363,17.7305069581,25.102843518,27.4630296434),.UNSPECIFIED.);
#1690=B_SPLINE_CURVE_WITH_KNOTS('',5,(#76348,#76349,#76350,#76351,#76352,
#76353,#76354,#76355,#76356,#76357,#76358,#76359,#76360,#76361,#76362,#76363,
#76364,#76365),.UNSPECIFIED.,.F.,.F.,(6,3,3,3,3,6),(-1.28529178055,0.,8.34825709363,
17.7305069581,25.102843518,27.4630296434),.UNSPECIFIED.);
#1691=B_SPLINE_CURVE_WITH_KNOTS('',5,(#76412,#76413,#76414,#76415,#76416,
#76417,#76418,#76419,#76420,#76421,#76422,#76423,#76424,#76425,#76426,#76427,
#76428,#76429),.UNSPECIFIED.,.F.,.F.,(6,3,3,3,3,6),(-1.28529177837993,0.,
8.34825709363,17.7305069581,25.102843518,27.4630296434),.UNSPECIFIED.);
#1692=B_SPLINE_CURVE_WITH_KNOTS('',5,(#76430,#76431,#76432,#76433,#76434,
#76435,#76436,#76437,#76438,#76439,#76440,#76441,#76442,#76443,#76444,#76445,
#76446,#76447),.UNSPECIFIED.,.F.,.F.,(6,3,3,3,3,6),(0.,0.0447084113745589,
0.335099525711938,0.661457705937853,0.917901776225663,1.),.UNSPECIFIED.);
#1693=B_SPLINE_CURVE_WITH_KNOTS('',5,(#76467,#76468,#76469,#76470,#76471,
#76472,#76473,#76474,#76475),.UNSPECIFIED.,.F.,.F.,(6,3,6),(0.,0.278583571948246,
1.),.UNSPECIFIED.);
#1694=B_SPLINE_CURVE_WITH_KNOTS('',5,(#76477,#76478,#76479,#76480,#76481,
#76482,#76483,#76484,#76485),.UNSPECIFIED.,.F.,.F.,(6,3,6),(0.,1.07297825382,
3.85154891337),.UNSPECIFIED.);
#1695=B_SPLINE_CURVE_WITH_KNOTS('',5,(#76520,#76521,#76522,#76523,#76524,
#76525,#76526,#76527,#76528,#76529,#76530,#76531,#76532,#76533,#76534),
 .UNSPECIFIED.,.F.,.F.,(6,3,3,3,6),(0.,2.13949651284,3.65547289001,4.94562974894,
5.62440522293),.UNSPECIFIED.);
#1696=B_SPLINE_CURVE_WITH_KNOTS('',5,(#76535,#76536,#76537,#76538,#76539,
#76540,#76541,#76542,#76543,#76544,#76545,#76546,#76547,#76548,#76549),
 .UNSPECIFIED.,.F.,.F.,(6,3,3,3,6),(0.,0.380395157894659,0.649930569566199,
0.879316043726239,1.),.UNSPECIFIED.);
#1697=B_SPLINE_CURVE_WITH_KNOTS('',5,(#76565,#76566,#76567,#76568,#76569,
#76570),.UNSPECIFIED.,.F.,.F.,(6,6),(0.,0.144177579366703),
 .UNSPECIFIED.);
#1698=B_SPLINE_CURVE_WITH_KNOTS('',5,(#76575,#76576,#76577,#76578,#76579,
#76580),.UNSPECIFIED.,.F.,.F.,(6,6),(0.,0.144177579366703),
 .UNSPECIFIED.);
#1699=B_SPLINE_CURVE_WITH_KNOTS('',5,(#76582,#76583,#76584,#76585,#76586,
#76587),.UNSPECIFIED.,.F.,.F.,(6,6),(0.266540302038896,2.4758008952433),
 .UNSPECIFIED.);
#1700=B_SPLINE_CURVE_WITH_KNOTS('',5,(#76602,#76603,#76604,#76605,#76606,
#76607),.UNSPECIFIED.,.F.,.F.,(6,6),(0.,3.5713550833),.UNSPECIFIED.);
#1701=B_SPLINE_CURVE_WITH_KNOTS('',5,(#76610,#76611,#76612,#76613,#76614,
#76615),.UNSPECIFIED.,.F.,.F.,(6,6),(2.4758008952433,3.5713550833),
 .UNSPECIFIED.);
#1702=B_SPLINE_CURVE_WITH_KNOTS('',5,(#76619,#76620,#76621,#76622,#76623,
#76624,#76625,#76626,#76627,#76628,#76629,#76630,#76631),.UNSPECIFIED.,
 .F.,.F.,(6,2,2,1,2,6),(0.,0.129543792616671,0.328284019716155,0.555394747336254,
0.717494953154769,1.),.UNSPECIFIED.);
#1703=B_SPLINE_CURVE_WITH_KNOTS('',5,(#76635,#76636,#76637,#76638,#76639,
#76640,#76641,#76642,#76643,#76644,#76645,#76646,#76647,#76648,#76649,#76650,
#76651,#76652),.UNSPECIFIED.,.F.,.F.,(6,3,3,3,3,6),(2.04066423734,2.62011481805,
3.50908168923,4.52495007124,5.25002578886,6.51367347233),.UNSPECIFIED.);
#1704=B_SPLINE_CURVE_WITH_KNOTS('',5,(#76653,#76654,#76655,#76656,#76657,
#76658),.UNSPECIFIED.,.F.,.F.,(6,6),(2.47580089524329,3.5713550833),
 .UNSPECIFIED.);
#1705=B_SPLINE_CURVE_WITH_KNOTS('',5,(#76660,#76661,#76662,#76663,#76664,
#76665),.UNSPECIFIED.,.F.,.F.,(6,6),(0.266540302038896,2.47580089524329),
 .UNSPECIFIED.);
#1706=B_SPLINE_CURVE_WITH_KNOTS('',5,(#76682,#76683,#76684,#76685,#76686,
#76687),.UNSPECIFIED.,.F.,.F.,(6,6),(0.,3.5713550833),.UNSPECIFIED.);
#1707=B_SPLINE_CURVE_WITH_KNOTS('',5,(#76693,#76694,#76695,#76696,#76697,
#76698,#76699,#76700,#76701,#76702,#76703,#76704),.UNSPECIFIED.,.F.,.F.,
(6,3,3,6),(0.380642553355298,3.39713474113,6.68643994484,8.37826425912),
 .UNSPECIFIED.);
#1708=B_SPLINE_CURVE_WITH_KNOTS('',5,(#76706,#76707,#76708,#76709,#76710,
#76711),.UNSPECIFIED.,.F.,.F.,(6,6),(0.836079546685,9.68451754643),
 .UNSPECIFIED.);
#1709=B_SPLINE_CURVE_WITH_KNOTS('',3,(#76714,#76715,#76716,#76717),
 .UNSPECIFIED.,.F.,.F.,(4,4),(0.,1.89584162936),.UNSPECIFIED.);
#1710=B_SPLINE_CURVE_WITH_KNOTS('',3,(#76721,#76722,#76723,#76724,#76725,
#76726),.UNSPECIFIED.,.F.,.F.,(4,2,4),(-0.0280207886793255,-0.0140109256855064,
-1.00277206334723E-6),.UNSPECIFIED.);
#1711=B_SPLINE_CURVE_WITH_KNOTS('',5,(#76728,#76729,#76730,#76731,#76732,
#76733),.UNSPECIFIED.,.F.,.F.,(6,6),(0.,1.1155886229),.UNSPECIFIED.);
#1712=B_SPLINE_CURVE_WITH_KNOTS('',5,(#76735,#76736,#76737,#76738,#76739,
#76740,#76741,#76742,#76743,#76744,#76745,#76746,#76747,#76748,#76749),
 .UNSPECIFIED.,.F.,.F.,(6,3,3,3,6),(0.,0.404403504835335,0.600830610026598,
0.80245741666853,1.),.UNSPECIFIED.);
#1713=B_SPLINE_CURVE_WITH_KNOTS('',5,(#76751,#76752,#76753,#76754,#76755,
#76756),.UNSPECIFIED.,.F.,.F.,(6,6),(0.,2.29845936737),.UNSPECIFIED.);
#1714=B_SPLINE_CURVE_WITH_KNOTS('',5,(#76759,#76760,#76761,#76762,#76763,
#76764,#76765,#76766,#76767,#76768,#76769,#76770,#76771,#76772,#76773),
 .UNSPECIFIED.,.F.,.F.,(6,3,3,3,6),(3.5609211009699,6.696077534,12.6191089245,
16.7682744334,17.8619151354404),.UNSPECIFIED.);
#1715=B_SPLINE_CURVE_WITH_KNOTS('',5,(#76776,#76777,#76778,#76779,#76780,
#76781),.UNSPECIFIED.,.F.,.F.,(6,6),(1.73726460462955E-9,3.5609211009699),
 .UNSPECIFIED.);
#1716=B_SPLINE_CURVE_WITH_KNOTS('',5,(#76790,#76791,#76792,#76793,#76794,
#76795,#76796,#76797,#76798,#76799,#76800,#76801,#76802,#76803,#76804),
 .UNSPECIFIED.,.F.,.F.,(6,3,3,3,6),(3.56092110096989,6.696077534,12.6191089245,
16.7682744334,17.8619151354404),.UNSPECIFIED.);
#1717=B_SPLINE_CURVE_WITH_KNOTS('',5,(#76814,#76815,#76816,#76817,#76818,
#76819),.UNSPECIFIED.,.F.,.F.,(6,6),(1.73726460462955E-9,3.56092110096989),
 .UNSPECIFIED.);
#1718=B_SPLINE_CURVE_WITH_KNOTS('',5,(#76822,#76823,#76824,#76825,#76826,
#76827,#76828,#76829,#76830,#76831,#76832,#76833),.UNSPECIFIED.,.F.,.F.,
(6,3,3,6),(0.380642553355298,3.39713474113,6.68643994484,8.37826425912),
 .UNSPECIFIED.);
#1719=B_SPLINE_CURVE_WITH_KNOTS('',3,(#76838,#76839,#76840,#76841),
 .UNSPECIFIED.,.F.,.F.,(4,4),(0.,1.89584162936),.UNSPECIFIED.);
#1720=B_SPLINE_CURVE_WITH_KNOTS('',5,(#76844,#76845,#76846,#76847,#76848,
#76849),.UNSPECIFIED.,.F.,.F.,(6,6),(0.836079546685,9.68451754643),
 .UNSPECIFIED.);
#1721=B_SPLINE_CURVE_WITH_KNOTS('',5,(#76855,#76856,#76857,#76858,#76859,
#76860),.UNSPECIFIED.,.F.,.F.,(6,6),(0.,2.29845936737),.UNSPECIFIED.);
#1722=B_SPLINE_CURVE_WITH_KNOTS('',5,(#76862,#76863,#76864,#76865,#76866,
#76867,#76868,#76869,#76870,#76871,#76872,#76873,#76874,#76875,#76876),
 .UNSPECIFIED.,.F.,.F.,(6,3,3,3,6),(0.,1.14196741734,1.69664449439,2.26600465298,
2.82383165251),.UNSPECIFIED.);
#1723=B_SPLINE_CURVE_WITH_KNOTS('',5,(#76878,#76879,#76880,#76881,#76882,
#76883),.UNSPECIFIED.,.F.,.F.,(6,6),(0.,1.1155886229),.UNSPECIFIED.);
#1724=B_SPLINE_CURVE_WITH_KNOTS('',3,(#76884,#76885,#76886,#76887,#76888,
#76889),.UNSPECIFIED.,.F.,.F.,(4,2,4),(-0.0280207886793728,-0.0140109256855102,
-1.0027720631911E-6),.UNSPECIFIED.);
#1725=B_SPLINE_CURVE_WITH_KNOTS('',5,(#76893,#76894,#76895,#76896,#76897,
#76898,#76899,#76900,#76901,#76902,#76903,#76904,#76905,#76906,#76907),
 .UNSPECIFIED.,.F.,.F.,(6,3,3,3,6),(0.,1.06902836413,2.19771269917,3.2241260379,
4.7004853448),.UNSPECIFIED.);
#1726=B_SPLINE_CURVE_WITH_KNOTS('',5,(#76909,#76910,#76911,#76912,#76913,
#76914),.UNSPECIFIED.,.F.,.F.,(6,6),(0.,6.43612007405),.UNSPECIFIED.);
#1727=B_SPLINE_CURVE_WITH_KNOTS('',5,(#76926,#76927,#76928,#76929,#76930,
#76931,#76932,#76933,#76934,#76935,#76936,#76937,#76938,#76939,#76940),
 .UNSPECIFIED.,.F.,.F.,(6,3,3,3,6),(0.0395158293388482,7.53253625942,14.2747183071,
18.8083875826,22.71906151),.UNSPECIFIED.);
#1728=B_SPLINE_CURVE_WITH_KNOTS('',5,(#76941,#76942,#76943,#76944,#76945,
#76946,#76947,#76948,#76949),.UNSPECIFIED.,.F.,.F.,(6,3,6),(0.,0.365735348523741,
1.),.UNSPECIFIED.);
#1729=B_SPLINE_CURVE_WITH_KNOTS('',5,(#76952,#76953,#76954,#76955,#76956,
#76957,#76958,#76959,#76960),.UNSPECIFIED.,.F.,.F.,(6,3,6),(0.,2.92723336323,
3.88093368919),.UNSPECIFIED.);
#1730=B_SPLINE_CURVE_WITH_KNOTS('',5,(#76962,#76963,#76964,#76965,#76966,
#76967,#76968,#76969,#76970,#76971,#76972,#76973,#76974,#76975,#76976,#76977,
#76978),.UNSPECIFIED.,.F.,.F.,(6,3,3,5,6),(3.11522256756,4.13897763214,
6.99130562041,9.89933117719,9.89969814681689),.UNSPECIFIED.);
#1731=B_SPLINE_CURVE_WITH_KNOTS('',5,(#76982,#76983,#76984,#76985,#76986,
#76987,#76988,#76989,#76990,#76991,#76992,#76993),.UNSPECIFIED.,.F.,.F.,
(6,3,3,6),(3.11522256756,4.13897763214,6.99130562041,9.89912618426),
 .UNSPECIFIED.);
#1732=B_SPLINE_CURVE_WITH_KNOTS('',5,(#76995,#76996,#76997,#76998,#76999,
#77000,#77001,#77002,#77003,#77004,#77005,#77006,#77007,#77008),
 .UNSPECIFIED.,.F.,.F.,(6,3,5,6),(0.,2.92723336323,3.88093368919,3.88140412218319),
 .UNSPECIFIED.);
#1733=B_SPLINE_CURVE_WITH_KNOTS('',5,(#77024,#77025,#77026,#77027,#77028,
#77029),.UNSPECIFIED.,.F.,.F.,(6,6),(0.,1.),.UNSPECIFIED.);
#1734=B_SPLINE_CURVE_WITH_KNOTS('',5,(#77031,#77032,#77033,#77034,#77035,
#77036,#77037,#77038,#77039,#77040,#77041,#77042,#77043,#77044,#77045),
 .UNSPECIFIED.,.F.,.F.,(6,3,3,3,6),(0.,0.227429357973136,0.467550165133747,
0.685913432634515,1.),.UNSPECIFIED.);
#1735=B_SPLINE_CURVE_WITH_KNOTS('',5,(#77047,#77048,#77049,#77050,#77051,
#77052,#77053,#77054,#77055),.UNSPECIFIED.,.F.,.F.,(6,3,6),(1.18944404077E-12,
1.10170421198,3.01229896543),.UNSPECIFIED.);
#1736=B_SPLINE_CURVE_WITH_KNOTS('',5,(#77056,#77057,#77058,#77059,#77060,
#77061,#77062,#77063,#77064,#77065,#77066,#77067,#77068,#77069,#77070),
 .UNSPECIFIED.,.F.,.F.,(6,3,3,3,6),(0.0395158293387482,7.53253625942,14.2747183071,
18.8083875826,22.71906151),.UNSPECIFIED.);
#1737=B_SPLINE_CURVE_WITH_KNOTS('',5,(#77114,#77115,#77116,#77117,#77118,
#77119,#77120,#77121,#77122,#77123,#77124,#77125,#77126,#77127,#77128,#77129,
#77130,#77131),.UNSPECIFIED.,.F.,.F.,(6,3,3,3,3,6),(2.04066423734,2.62011481805,
3.50908168923,4.52495007124,5.25002578886,6.51367347233),.UNSPECIFIED.);
#1738=B_SPLINE_CURVE_WITH_KNOTS('',5,(#77136,#77137,#77138,#77139,#77140,
#77141,#77142,#77143,#77144,#77145,#77146,#77147,#77148,#77149,#77150,#77151,
#77152),.UNSPECIFIED.,.F.,.F.,(6,3,3,5,6),(3.11522256756,4.13897763214,
6.99130562041,9.89933117719,9.89969814681689),.UNSPECIFIED.);
#1739=B_SPLINE_CURVE_WITH_KNOTS('',5,(#77154,#77155,#77156,#77157,#77158,
#77159,#77160,#77161,#77162),.UNSPECIFIED.,.F.,.F.,(6,3,6),(0.,0.754260082150734,
1.),.UNSPECIFIED.);
#1740=B_SPLINE_CURVE_WITH_KNOTS('',5,(#77168,#77169,#77170,#77171,#77172,
#77173,#77174,#77175,#77176,#77177,#77178,#77179,#77180,#77181),
 .UNSPECIFIED.,.F.,.F.,(6,3,5,6),(0.,2.92723336323,3.88093368919,3.88140411694228),
 .UNSPECIFIED.);
#1741=B_SPLINE_CURVE_WITH_KNOTS('',5,(#77183,#77184,#77185,#77186,#77187,
#77188,#77189,#77190,#77191,#77192,#77193,#77194),.UNSPECIFIED.,.F.,.F.,
(6,3,3,6),(3.11522256756,4.13897763214,6.99130562041,9.89912618426),
 .UNSPECIFIED.);
#1742=B_SPLINE_CURVE_WITH_KNOTS('',5,(#77198,#77199,#77200,#77201,#77202,
#77203,#77204,#77205,#77206,#77207,#77208,#77209,#77210,#77211,#77212,#77213,
#77214,#77215),.UNSPECIFIED.,.F.,.F.,(6,3,3,3,3,6),(2.04066423734,2.62011481805,
3.50908168923,4.52495007124,5.25002578886,6.51367347233),.UNSPECIFIED.);
#1743=B_SPLINE_CURVE_WITH_KNOTS('',5,(#77281,#77282,#77283,#77284,#77285,
#77286,#77287,#77288,#77289,#77290,#77291,#77292),.UNSPECIFIED.,.F.,.F.,
(6,3,3,6),(0.,3.39713474113,6.68643994484,8.37826425912),.UNSPECIFIED.);
#1744=B_SPLINE_CURVE_WITH_KNOTS('',5,(#77318,#77319,#77320,#77321,#77322,
#77323,#77324,#77325,#77326),.UNSPECIFIED.,.F.,.F.,(6,3,6),(0.,2.6134611976,
3.73613338933),.UNSPECIFIED.);
#1745=B_SPLINE_CURVE_WITH_KNOTS('',5,(#77341,#77342,#77343,#77344,#77345,
#77346),.UNSPECIFIED.,.F.,.F.,(6,6),(0.,1.1155886229),.UNSPECIFIED.);
#1746=B_SPLINE_CURVE_WITH_KNOTS('',5,(#77379,#77380,#77381,#77382,#77383,
#77384,#77385,#77386,#77387,#77388,#77389,#77390,#77391,#77392,#77393),
 .UNSPECIFIED.,.F.,.F.,(6,3,3,3,6),(0.,1.14196741734,1.69664449439,2.26600465298,
2.82383165251),.UNSPECIFIED.);
#1747=B_SPLINE_CURVE_WITH_KNOTS('',5,(#77407,#77408,#77409,#77410,#77411,
#77412),.UNSPECIFIED.,.F.,.F.,(6,6),(0.,2.29845936737),.UNSPECIFIED.);
#1748=B_SPLINE_CURVE_WITH_KNOTS('',5,(#77445,#77446,#77447,#77448,#77449,
#77450,#77451,#77452,#77453,#77454,#77455,#77456,#77457,#77458,#77459),
 .UNSPECIFIED.,.F.,.F.,(6,3,3,3,6),(1.73726460462955E-9,6.696077534,12.6191089245,
16.7682744334,17.9215041098),.UNSPECIFIED.);
#1749=B_SPLINE_CURVE_WITH_KNOTS('',5,(#77503,#77504,#77505,#77506,#77507,
#77508,#77509,#77510,#77511,#77512,#77513,#77514,#77515,#77516,#77517),
 .UNSPECIFIED.,.F.,.F.,(6,3,3,3,6),(1.73726460462955E-9,6.696077534,12.6191089245,
16.7682744334,17.9215041098),.UNSPECIFIED.);
#1750=B_SPLINE_CURVE_WITH_KNOTS('',5,(#77540,#77541,#77542,#77543,#77544,
#77545,#77546,#77547,#77548),.UNSPECIFIED.,.F.,.F.,(6,3,6),(0.,0.699509606660128,
1.),.UNSPECIFIED.);
#1751=B_SPLINE_CURVE_WITH_KNOTS('',5,(#77590,#77591,#77592,#77593,#77594,
#77595,#77596,#77597,#77598,#77599,#77600,#77601),.UNSPECIFIED.,.F.,.F.,
(6,3,3,6),(0.,0.405469991881924,0.798069831416645,1.),.UNSPECIFIED.);
#1752=B_SPLINE_CURVE_WITH_KNOTS('',5,(#77616,#77617,#77618,#77619,#77620,
#77621),.UNSPECIFIED.,.F.,.F.,(6,6),(0.,2.29845936737),.UNSPECIFIED.);
#1753=B_SPLINE_CURVE_WITH_KNOTS('',5,(#77654,#77655,#77656,#77657,#77658,
#77659,#77660,#77661,#77662,#77663,#77664,#77665,#77666,#77667,#77668),
 .UNSPECIFIED.,.F.,.F.,(6,3,3,3,6),(0.,0.404403504835335,0.600830610026598,
0.80245741666853,1.),.UNSPECIFIED.);
#1754=B_SPLINE_CURVE_WITH_KNOTS('',5,(#77682,#77683,#77684,#77685,#77686,
#77687),.UNSPECIFIED.,.F.,.F.,(6,6),(0.,1.1155886229),.UNSPECIFIED.);
#1755=B_SPLINE_CURVE_WITH_KNOTS('',5,(#77721,#77722,#77723,#77724,#77725,
#77726,#77727,#77728,#77729,#77730,#77731,#77732,#77733,#77734,#77735),
 .UNSPECIFIED.,.F.,.F.,(6,3,3,3,6),(0.,0.227429357973136,0.467550165133747,
0.685913432634515,1.),.UNSPECIFIED.);
#1756=B_SPLINE_CURVE_WITH_KNOTS('',5,(#77750,#77751,#77752,#77753,#77754,
#77755),.UNSPECIFIED.,.F.,.F.,(6,6),(0.,1.),.UNSPECIFIED.);
#1757=B_SPLINE_CURVE_WITH_KNOTS('',5,(#77808,#77809,#77810,#77811,#77812,
#77813,#77814,#77815,#77816,#77817,#77818,#77819,#77820,#77821,#77822),
 .UNSPECIFIED.,.F.,.F.,(6,3,3,3,6),(0.0395158293388482,7.53253625942,14.2747183071,
18.8083875826,22.71906151),.UNSPECIFIED.);
#1758=B_SPLINE_CURVE_WITH_KNOTS('',5,(#77842,#77843,#77844,#77845,#77846,
#77847,#77848,#77849,#77850),.UNSPECIFIED.,.F.,.F.,(6,3,6),(1.18944404077E-12,
1.10170421198,3.01229896543),.UNSPECIFIED.);
#1759=B_SPLINE_CURVE_WITH_KNOTS('',5,(#78000,#78001,#78002,#78003,#78004,
#78005),.UNSPECIFIED.,.F.,.F.,(6,6),(0.,6.43612007405),.UNSPECIFIED.);
#1760=B_SPLINE_CURVE_WITH_KNOTS('',5,(#78038,#78039,#78040,#78041,#78042,
#78043,#78044,#78045,#78046,#78047,#78048,#78049,#78050,#78051,#78052),
 .UNSPECIFIED.,.F.,.F.,(6,3,3,3,6),(0.,1.06902836413,2.19771269917,3.2241260379,
4.7004853448),.UNSPECIFIED.);
#1761=B_SPLINE_CURVE_WITH_KNOTS('',5,(#78073,#78074,#78075,#78076,#78077,
#78078,#78079,#78080,#78081),.UNSPECIFIED.,.F.,.F.,(6,3,6),(0.,0.365735348523741,
1.),.UNSPECIFIED.);
#1762=B_SPLINE_CURVE_WITH_KNOTS('',5,(#78113,#78114,#78115,#78116,#78117,
#78118,#78119,#78120,#78121,#78122,#78123,#78124,#78125,#78126,#78127),
 .UNSPECIFIED.,.F.,.F.,(6,3,3,3,6),(0.0395158293387482,7.53253625942,14.2747183071,
18.8083875826,22.71906151),.UNSPECIFIED.);
#2047=SHAPE_REPRESENTATION_RELATIONSHIP('SRR','None',#98344,#2057);
#2057=ADVANCED_BREP_SHAPE_REPRESENTATION('',(#65),#98296);
#2067=STYLED_ITEM('',(#98399),#65);
#2131=PLANE('',#34963);
#2132=PLANE('',#34967);
#2133=PLANE('',#34968);
#2134=PLANE('',#34969);
#2135=PLANE('',#34971);
#2136=PLANE('',#34974);
#2137=PLANE('',#34982);
#2138=PLANE('',#34983);
#2139=PLANE('',#35015);
#2140=PLANE('',#35017);
#2141=PLANE('',#35020);
#2142=PLANE('',#35031);
#2143=PLANE('',#35032);
#2144=PLANE('',#35037);
#2145=PLANE('',#35038);
#2146=PLANE('',#35049);
#2147=PLANE('',#35050);
#2148=PLANE('',#35055);
#2149=PLANE('',#35056);
#2150=PLANE('',#35061);
#2151=PLANE('',#35074);
#2152=PLANE('',#35075);
#2153=PLANE('',#35076);
#2154=PLANE('',#35079);
#2155=PLANE('',#35080);
#2156=PLANE('',#35090);
#2157=PLANE('',#35091);
#2158=PLANE('',#35094);
#2159=PLANE('',#35098);
#2160=PLANE('',#35099);
#2161=PLANE('',#35110);
#2162=PLANE('',#35123);
#2163=PLANE('',#35126);
#2164=PLANE('',#35127);
#2165=PLANE('',#35131);
#2166=PLANE('',#35141);
#2167=PLANE('',#35142);
#2168=PLANE('',#35143);
#2169=PLANE('',#35144);
#2170=PLANE('',#35145);
#2171=PLANE('',#35147);
#2172=PLANE('',#35148);
#2173=PLANE('',#35149);
#2174=PLANE('',#35150);
#2175=PLANE('',#35151);
#2176=PLANE('',#35152);
#2177=PLANE('',#35153);
#2178=PLANE('',#35154);
#2179=PLANE('',#35155);
#2180=PLANE('',#35157);
#2181=PLANE('',#35158);
#2182=PLANE('',#35162);
#2183=PLANE('',#35163);
#2184=PLANE('',#35165);
#2185=PLANE('',#35166);
#2186=PLANE('',#35167);
#2187=PLANE('',#35168);
#2188=PLANE('',#35169);
#2189=PLANE('',#35171);
#2190=PLANE('',#35173);
#2191=PLANE('',#35174);
#2192=PLANE('',#35176);
#2193=PLANE('',#35178);
#2194=PLANE('',#35182);
#2195=PLANE('',#35192);
#2196=PLANE('',#35194);
#2197=PLANE('',#35196);
#2198=PLANE('',#35222);
#2199=PLANE('',#35223);
#2200=PLANE('',#35226);
#2201=PLANE('',#35229);
#2202=PLANE('',#35233);
#2203=PLANE('',#35260);
#2204=PLANE('',#35264);
#2205=PLANE('',#35265);
#2206=PLANE('',#35266);
#2207=PLANE('',#35268);
#2208=PLANE('',#35271);
#2209=PLANE('',#35280);
#2210=PLANE('',#35292);
#2211=PLANE('',#35297);
#2212=PLANE('',#35302);
#2213=PLANE('',#35318);
#2214=PLANE('',#35322);
#2215=PLANE('',#35324);
#2216=PLANE('',#35328);
#2217=PLANE('',#35332);
#2218=PLANE('',#35339);
#2219=PLANE('',#35356);
#2220=PLANE('',#35372);
#2221=PLANE('',#35375);
#2222=PLANE('',#35378);
#2223=PLANE('',#35379);
#2224=PLANE('',#35381);
#2225=PLANE('',#35382);
#2226=PLANE('',#35386);
#2227=PLANE('',#35387);
#2228=PLANE('',#35389);
#2229=PLANE('',#35390);
#2230=PLANE('',#35394);
#2231=PLANE('',#35395);
#2232=PLANE('',#35399);
#2233=PLANE('',#35403);
#2234=PLANE('',#35404);
#2235=PLANE('',#35406);
#2236=PLANE('',#35422);
#2237=PLANE('',#35432);
#2238=PLANE('',#35437);
#2239=PLANE('',#35446);
#2240=PLANE('',#35458);
#2241=PLANE('',#35463);
#2242=PLANE('',#35464);
#2243=PLANE('',#35465);
#2244=PLANE('',#35466);
#2245=PLANE('',#35467);
#2246=PLANE('',#35468);
#2247=PLANE('',#35469);
#2248=PLANE('',#35470);
#2249=PLANE('',#35471);
#2250=PLANE('',#35472);
#2251=PLANE('',#35473);
#2252=PLANE('',#35474);
#2253=PLANE('',#35475);
#2254=PLANE('',#35476);
#2255=PLANE('',#35477);
#2256=PLANE('',#35479);
#2257=PLANE('',#35481);
#2258=PLANE('',#35494);
#2259=PLANE('',#35496);
#2260=PLANE('',#35516);
#2261=PLANE('',#35546);
#2262=PLANE('',#35549);
#2263=PLANE('',#35553);
#2264=PLANE('',#35572);
#2265=PLANE('',#35602);
#2266=PLANE('',#35604);
#2267=PLANE('',#35606);
#2268=PLANE('',#35608);
#2269=PLANE('',#35611);
#2270=PLANE('',#35630);
#2271=PLANE('',#35660);
#2272=PLANE('',#35663);
#2273=PLANE('',#35667);
#2274=PLANE('',#35679);
#2275=PLANE('',#35715);
#2276=PLANE('',#35718);
#2277=PLANE('',#35721);
#2278=PLANE('',#35722);
#2279=PLANE('',#35725);
#2620=CYLINDRICAL_SURFACE('',#34965,6.69050581799);
#2621=CYLINDRICAL_SURFACE('',#34972,6.69050581799);
#2622=CYLINDRICAL_SURFACE('',#34975,4.44342636361);
#2623=CYLINDRICAL_SURFACE('',#34979,6.24342636361);
#2624=CYLINDRICAL_SURFACE('',#35013,16.1);
#2625=CYLINDRICAL_SURFACE('',#35021,16.4);
#2626=CYLINDRICAL_SURFACE('',#35033,17.4);
#2627=CYLINDRICAL_SURFACE('',#35039,16.4);
#2628=CYLINDRICAL_SURFACE('',#35051,17.4);
#2629=CYLINDRICAL_SURFACE('',#35057,16.1);
#2630=CYLINDRICAL_SURFACE('',#35062,7.6);
#2631=CYLINDRICAL_SURFACE('',#35067,0.2);
#2632=CYLINDRICAL_SURFACE('',#35069,7.6);
#2633=CYLINDRICAL_SURFACE('',#35077,16.1);
#2634=CYLINDRICAL_SURFACE('',#35081,7.6);
#2635=CYLINDRICAL_SURFACE('',#35084,0.2);
#2636=CYLINDRICAL_SURFACE('',#35086,0.2);
#2637=CYLINDRICAL_SURFACE('',#35088,7.6);
#2638=CYLINDRICAL_SURFACE('',#35092,7.34342636361001);
#2639=CYLINDRICAL_SURFACE('',#35095,16.1);
#2640=CYLINDRICAL_SURFACE('',#35100,7.34342636361001);
#2641=CYLINDRICAL_SURFACE('',#35102,2.25);
#2642=CYLINDRICAL_SURFACE('',#35108,6.24342636361);
#2643=CYLINDRICAL_SURFACE('',#35111,0.5);
#2644=CYLINDRICAL_SURFACE('',#35113,6.5);
#2645=CYLINDRICAL_SURFACE('',#35115,0.5);
#2646=CYLINDRICAL_SURFACE('',#35117,0.5);
#2647=CYLINDRICAL_SURFACE('',#35119,6.5);
#2648=CYLINDRICAL_SURFACE('',#35121,0.5);
#2649=CYLINDRICAL_SURFACE('',#35124,7.34342636361001);
#2650=CYLINDRICAL_SURFACE('',#35128,16.1);
#2651=CYLINDRICAL_SURFACE('',#35132,7.34342636361001);
#2652=CYLINDRICAL_SURFACE('',#35134,2.25);
#2653=CYLINDRICAL_SURFACE('',#35160,0.700000000000002);
#2654=CYLINDRICAL_SURFACE('',#35161,0.700000000000002);
#2655=CYLINDRICAL_SURFACE('',#35200,0.700000000000002);
#2656=CYLINDRICAL_SURFACE('',#35201,16.4);
#2657=CYLINDRICAL_SURFACE('',#35204,15.4);
#2658=CYLINDRICAL_SURFACE('',#35207,15.4);
#2659=CYLINDRICAL_SURFACE('',#35210,15.4);
#2660=CYLINDRICAL_SURFACE('',#35213,15.4);
#2661=CYLINDRICAL_SURFACE('',#35216,15.4);
#2662=CYLINDRICAL_SURFACE('',#35219,15.4);
#2663=CYLINDRICAL_SURFACE('',#35225,16.7);
#2664=CYLINDRICAL_SURFACE('',#35243,15.4);
#2665=CYLINDRICAL_SURFACE('',#35245,15.4);
#2666=CYLINDRICAL_SURFACE('',#35247,15.4);
#2667=CYLINDRICAL_SURFACE('',#35249,15.4);
#2668=CYLINDRICAL_SURFACE('',#35252,15.4);
#2669=CYLINDRICAL_SURFACE('',#35255,15.4);
#2670=CYLINDRICAL_SURFACE('',#35258,16.4);
#2671=CYLINDRICAL_SURFACE('',#35261,0.700000000000002);
#2672=CYLINDRICAL_SURFACE('',#35262,16.7);
#2673=CYLINDRICAL_SURFACE('',#35282,0.5);
#2674=CYLINDRICAL_SURFACE('',#35284,6.5);
#2675=CYLINDRICAL_SURFACE('',#35286,0.5);
#2676=CYLINDRICAL_SURFACE('',#35288,6.5);
#2677=CYLINDRICAL_SURFACE('',#35290,0.5);
#2678=CYLINDRICAL_SURFACE('',#35293,5.24342636361);
#2679=CYLINDRICAL_SURFACE('',#35295,5.24342636361);
#2680=CYLINDRICAL_SURFACE('',#35298,5.5);
#2681=CYLINDRICAL_SURFACE('',#35300,5.5);
#2682=CYLINDRICAL_SURFACE('',#35304,7.04342636361);
#2683=CYLINDRICAL_SURFACE('',#35306,0.1);
#2684=CYLINDRICAL_SURFACE('',#35308,10.8);
#2685=CYLINDRICAL_SURFACE('',#35310,10.8);
#2686=CYLINDRICAL_SURFACE('',#35312,0.1);
#2687=CYLINDRICAL_SURFACE('',#35314,7.04342636361);
#2688=CYLINDRICAL_SURFACE('',#35316,1.25);
#2689=CYLINDRICAL_SURFACE('',#35326,1.25);
#2690=CYLINDRICAL_SURFACE('',#35329,4.44342636361);
#2691=CYLINDRICAL_SURFACE('',#35333,7.3);
#2692=CYLINDRICAL_SURFACE('',#35336,7.3);
#2693=CYLINDRICAL_SURFACE('',#35340,4.7);
#2694=CYLINDRICAL_SURFACE('',#35348,4.7);
#2695=CYLINDRICAL_SURFACE('',#35357,6.24342636361);
#2696=CYLINDRICAL_SURFACE('',#35360,0.3);
#2697=CYLINDRICAL_SURFACE('',#35363,10.);
#2698=CYLINDRICAL_SURFACE('',#35366,0.3);
#2699=CYLINDRICAL_SURFACE('',#35369,6.24342636361);
#2700=CYLINDRICAL_SURFACE('',#35418,4.44342636361);
#2701=CYLINDRICAL_SURFACE('',#35420,4.44342636361);
#2702=CYLINDRICAL_SURFACE('',#35427,3.);
#2703=CYLINDRICAL_SURFACE('',#35428,0.3);
#2704=CYLINDRICAL_SURFACE('',#35430,0.3);
#2705=CYLINDRICAL_SURFACE('',#35433,0.3);
#2706=CYLINDRICAL_SURFACE('',#35435,0.3);
#2707=CYLINDRICAL_SURFACE('',#35438,0.3);
#2708=CYLINDRICAL_SURFACE('',#35440,0.3);
#2709=CYLINDRICAL_SURFACE('',#35442,5.69050581799);
#2710=CYLINDRICAL_SURFACE('',#35444,0.5);
#2711=CYLINDRICAL_SURFACE('',#35447,1.1);
#2712=CYLINDRICAL_SURFACE('',#35449,3.);
#2713=CYLINDRICAL_SURFACE('',#35451,3.);
#2714=CYLINDRICAL_SURFACE('',#35452,5.24342636361);
#2715=CYLINDRICAL_SURFACE('',#35453,5.24342636361);
#2716=CYLINDRICAL_SURFACE('',#35454,3.);
#2717=CYLINDRICAL_SURFACE('',#35456,1.1);
#2718=CYLINDRICAL_SURFACE('',#35459,0.5);
#2719=CYLINDRICAL_SURFACE('',#35461,5.69050581799);
#2720=CYLINDRICAL_SURFACE('',#35498,0.300000000000002);
#2721=CYLINDRICAL_SURFACE('',#35501,0.299999999999999);
#2722=CYLINDRICAL_SURFACE('',#35505,0.3);
#2723=CYLINDRICAL_SURFACE('',#35512,0.3);
#2724=CYLINDRICAL_SURFACE('',#35520,0.300000000000001);
#2725=CYLINDRICAL_SURFACE('',#35525,0.300000000000001);
#2726=CYLINDRICAL_SURFACE('',#35530,0.300000000000001);
#2727=CYLINDRICAL_SURFACE('',#35535,0.300000000000002);
#2728=CYLINDRICAL_SURFACE('',#35545,0.3);
#2729=CYLINDRICAL_SURFACE('',#35547,0.3);
#2730=CYLINDRICAL_SURFACE('',#35548,0.3);
#2731=CYLINDRICAL_SURFACE('',#35550,0.300000000000001);
#2732=CYLINDRICAL_SURFACE('',#35551,0.300000000000001);
#2733=CYLINDRICAL_SURFACE('',#35552,0.300000000000001);
#2734=CYLINDRICAL_SURFACE('',#35554,0.300000000000002);
#2735=CYLINDRICAL_SURFACE('',#35557,0.3);
#2736=CYLINDRICAL_SURFACE('',#35561,0.3);
#2737=CYLINDRICAL_SURFACE('',#35568,0.299999999999999);
#2738=CYLINDRICAL_SURFACE('',#35576,0.300000000000002);
#2739=CYLINDRICAL_SURFACE('',#35581,0.3);
#2740=CYLINDRICAL_SURFACE('',#35586,0.300000000000002);
#2741=CYLINDRICAL_SURFACE('',#35591,0.300000000000002);
#2742=CYLINDRICAL_SURFACE('',#35601,0.300000000000001);
#2743=CYLINDRICAL_SURFACE('',#35603,0.3);
#2744=CYLINDRICAL_SURFACE('',#35605,0.3);
#2745=CYLINDRICAL_SURFACE('',#35607,0.300000000000001);
#2746=CYLINDRICAL_SURFACE('',#35609,0.300000000000001);
#2747=CYLINDRICAL_SURFACE('',#35610,0.300000000000001);
#2748=CYLINDRICAL_SURFACE('',#35612,0.3);
#2749=CYLINDRICAL_SURFACE('',#35615,0.299999999999999);
#2750=CYLINDRICAL_SURFACE('',#35619,0.3);
#2751=CYLINDRICAL_SURFACE('',#35626,0.3);
#2752=CYLINDRICAL_SURFACE('',#35634,0.300000000000002);
#2753=CYLINDRICAL_SURFACE('',#35639,0.300000000000002);
#2754=CYLINDRICAL_SURFACE('',#35644,0.300000000000002);
#2755=CYLINDRICAL_SURFACE('',#35649,0.300000000000001);
#2756=CYLINDRICAL_SURFACE('',#35659,0.300000000000002);
#2757=CYLINDRICAL_SURFACE('',#35661,0.300000000000001);
#2758=CYLINDRICAL_SURFACE('',#35662,0.3);
#2759=CYLINDRICAL_SURFACE('',#35664,0.3);
#2760=CYLINDRICAL_SURFACE('',#35665,0.300000000000001);
#2761=CYLINDRICAL_SURFACE('',#35666,0.300000000000001);
#2762=CYLINDRICAL_SURFACE('',#35668,0.3);
#2763=CYLINDRICAL_SURFACE('',#35671,0.300000000000001);
#2764=CYLINDRICAL_SURFACE('',#35675,0.3);
#2765=CYLINDRICAL_SURFACE('',#35684,0.3);
#2766=CYLINDRICAL_SURFACE('',#35694,0.3);
#2767=CYLINDRICAL_SURFACE('',#35703,0.300000000000002);
#2768=CYLINDRICAL_SURFACE('',#35704,0.300000000000001);
#2769=CYLINDRICAL_SURFACE('',#35714,0.300000000000002);
#2770=CYLINDRICAL_SURFACE('',#35716,0.300000000000001);
#2771=CYLINDRICAL_SURFACE('',#35717,0.3);
#2772=CYLINDRICAL_SURFACE('',#35719,0.299999999999999);
#2773=CYLINDRICAL_SURFACE('',#35720,0.3);
#2774=CYLINDRICAL_SURFACE('',#35723,0.300000000000001);
#2775=CYLINDRICAL_SURFACE('',#35724,0.3);
#3729=FACE_OUTER_BOUND('',#5889,.T.);
#3730=FACE_OUTER_BOUND('',#5890,.T.);
#3731=FACE_OUTER_BOUND('',#5891,.T.);
#3732=FACE_OUTER_BOUND('',#5892,.T.);
#3733=FACE_OUTER_BOUND('',#5893,.T.);
#3734=FACE_OUTER_BOUND('',#5894,.T.);
#3735=FACE_OUTER_BOUND('',#5895,.T.);
#3736=FACE_OUTER_BOUND('',#5896,.T.);
#3737=FACE_OUTER_BOUND('',#5897,.T.);
#3738=FACE_OUTER_BOUND('',#5898,.T.);
#3739=FACE_OUTER_BOUND('',#5899,.T.);
#3740=FACE_OUTER_BOUND('',#5900,.T.);
#3741=FACE_OUTER_BOUND('',#5901,.T.);
#3742=FACE_OUTER_BOUND('',#5902,.T.);
#3743=FACE_OUTER_BOUND('',#5909,.T.);
#3744=FACE_OUTER_BOUND('',#5910,.T.);
#3745=FACE_OUTER_BOUND('',#5911,.T.);
#3746=FACE_OUTER_BOUND('',#5912,.T.);
#3747=FACE_OUTER_BOUND('',#5913,.T.);
#3748=FACE_OUTER_BOUND('',#5914,.T.);
#3749=FACE_OUTER_BOUND('',#5915,.T.);
#3750=FACE_OUTER_BOUND('',#5916,.T.);
#3751=FACE_OUTER_BOUND('',#5917,.T.);
#3752=FACE_OUTER_BOUND('',#5918,.T.);
#3753=FACE_OUTER_BOUND('',#5919,.T.);
#3754=FACE_OUTER_BOUND('',#5920,.T.);
#3755=FACE_OUTER_BOUND('',#5921,.T.);
#3756=FACE_OUTER_BOUND('',#5922,.T.);
#3757=FACE_OUTER_BOUND('',#5923,.T.);
#3758=FACE_OUTER_BOUND('',#5924,.T.);
#3759=FACE_OUTER_BOUND('',#5925,.T.);
#3760=FACE_OUTER_BOUND('',#5926,.T.);
#3761=FACE_OUTER_BOUND('',#5927,.T.);
#3762=FACE_OUTER_BOUND('',#5928,.T.);
#3763=FACE_OUTER_BOUND('',#5929,.T.);
#3764=FACE_OUTER_BOUND('',#5930,.T.);
#3765=FACE_OUTER_BOUND('',#5931,.T.);
#3766=FACE_OUTER_BOUND('',#5932,.T.);
#3767=FACE_OUTER_BOUND('',#5933,.T.);
#3768=FACE_OUTER_BOUND('',#5934,.T.);
#3769=FACE_OUTER_BOUND('',#5935,.T.);
#3770=FACE_OUTER_BOUND('',#5936,.T.);
#3771=FACE_OUTER_BOUND('',#5937,.T.);
#3772=FACE_OUTER_BOUND('',#5938,.T.);
#3773=FACE_OUTER_BOUND('',#5939,.T.);
#3774=FACE_OUTER_BOUND('',#5940,.T.);
#3775=FACE_OUTER_BOUND('',#5941,.T.);
#3776=FACE_OUTER_BOUND('',#5942,.T.);
#3777=FACE_OUTER_BOUND('',#5943,.T.);
#3778=FACE_OUTER_BOUND('',#5944,.T.);
#3779=FACE_OUTER_BOUND('',#5945,.T.);
#3780=FACE_OUTER_BOUND('',#5946,.T.);
#3781=FACE_OUTER_BOUND('',#5947,.T.);
#3782=FACE_OUTER_BOUND('',#5948,.T.);
#3783=FACE_OUTER_BOUND('',#5949,.T.);
#3784=FACE_OUTER_BOUND('',#5950,.T.);
#3785=FACE_OUTER_BOUND('',#5951,.T.);
#3786=FACE_OUTER_BOUND('',#5952,.T.);
#3787=FACE_OUTER_BOUND('',#5953,.T.);
#3788=FACE_OUTER_BOUND('',#5954,.T.);
#3789=FACE_OUTER_BOUND('',#5955,.T.);
#3790=FACE_OUTER_BOUND('',#5956,.T.);
#3791=FACE_OUTER_BOUND('',#5957,.T.);
#3792=FACE_OUTER_BOUND('',#5958,.T.);
#3793=FACE_OUTER_BOUND('',#5959,.T.);
#3794=FACE_OUTER_BOUND('',#5960,.T.);
#3795=FACE_OUTER_BOUND('',#5961,.T.);
#3796=FACE_OUTER_BOUND('',#5962,.T.);
#3797=FACE_OUTER_BOUND('',#5963,.T.);
#3798=FACE_OUTER_BOUND('',#5964,.T.);
#3799=FACE_OUTER_BOUND('',#5965,.T.);
#3800=FACE_OUTER_BOUND('',#5966,.T.);
#3801=FACE_OUTER_BOUND('',#5967,.T.);
#3802=FACE_OUTER_BOUND('',#5968,.T.);
#3803=FACE_OUTER_BOUND('',#5969,.T.);
#3804=FACE_OUTER_BOUND('',#5970,.T.);
#3805=FACE_OUTER_BOUND('',#5971,.T.);
#3806=FACE_OUTER_BOUND('',#5972,.T.);
#3807=FACE_OUTER_BOUND('',#5973,.T.);
#3808=FACE_OUTER_BOUND('',#5974,.T.);
#3809=FACE_OUTER_BOUND('',#5975,.T.);
#3810=FACE_OUTER_BOUND('',#5976,.T.);
#3811=FACE_OUTER_BOUND('',#5977,.T.);
#3812=FACE_OUTER_BOUND('',#5978,.T.);
#3813=FACE_OUTER_BOUND('',#5979,.T.);
#3814=FACE_OUTER_BOUND('',#5980,.T.);
#3815=FACE_OUTER_BOUND('',#5981,.T.);
#3816=FACE_OUTER_BOUND('',#5982,.T.);
#3817=FACE_OUTER_BOUND('',#5983,.T.);
#3818=FACE_OUTER_BOUND('',#5984,.T.);
#3819=FACE_OUTER_BOUND('',#5985,.T.);
#3820=FACE_OUTER_BOUND('',#5986,.T.);
#3821=FACE_OUTER_BOUND('',#5987,.T.);
#3822=FACE_OUTER_BOUND('',#5988,.T.);
#3823=FACE_OUTER_BOUND('',#5989,.T.);
#3824=FACE_OUTER_BOUND('',#5990,.T.);
#3825=FACE_OUTER_BOUND('',#5991,.T.);
#3826=FACE_OUTER_BOUND('',#5992,.T.);
#3827=FACE_OUTER_BOUND('',#5993,.T.);
#3828=FACE_OUTER_BOUND('',#5994,.T.);
#3829=FACE_OUTER_BOUND('',#5995,.T.);
#3830=FACE_OUTER_BOUND('',#5996,.T.);
#3831=FACE_OUTER_BOUND('',#5997,.T.);
#3832=FACE_OUTER_BOUND('',#5998,.T.);
#3833=FACE_OUTER_BOUND('',#5999,.T.);
#3834=FACE_OUTER_BOUND('',#6000,.T.);
#3835=FACE_OUTER_BOUND('',#6004,.T.);
#3836=FACE_OUTER_BOUND('',#6005,.T.);
#3837=FACE_OUTER_BOUND('',#6006,.T.);
#3838=FACE_OUTER_BOUND('',#6007,.T.);
#3839=FACE_OUTER_BOUND('',#6008,.T.);
#3840=FACE_OUTER_BOUND('',#6009,.T.);
#3841=FACE_OUTER_BOUND('',#6010,.T.);
#3842=FACE_OUTER_BOUND('',#6011,.T.);
#3843=FACE_OUTER_BOUND('',#6012,.T.);
#3844=FACE_OUTER_BOUND('',#6013,.T.);
#3845=FACE_OUTER_BOUND('',#6014,.T.);
#3846=FACE_OUTER_BOUND('',#6015,.T.);
#3847=FACE_OUTER_BOUND('',#6016,.T.);
#3848=FACE_OUTER_BOUND('',#6017,.T.);
#3849=FACE_OUTER_BOUND('',#6018,.T.);
#3850=FACE_OUTER_BOUND('',#6019,.T.);
#3851=FACE_OUTER_BOUND('',#6020,.T.);
#3852=FACE_OUTER_BOUND('',#6021,.T.);
#3853=FACE_OUTER_BOUND('',#6022,.T.);
#3854=FACE_OUTER_BOUND('',#6023,.T.);
#3855=FACE_OUTER_BOUND('',#6024,.T.);
#3856=FACE_OUTER_BOUND('',#6025,.T.);
#3857=FACE_OUTER_BOUND('',#6026,.T.);
#3858=FACE_OUTER_BOUND('',#6027,.T.);
#3859=FACE_OUTER_BOUND('',#6028,.T.);
#3860=FACE_OUTER_BOUND('',#6029,.T.);
#3861=FACE_OUTER_BOUND('',#6030,.T.);
#3862=FACE_OUTER_BOUND('',#6031,.T.);
#3863=FACE_OUTER_BOUND('',#6032,.T.);
#3864=FACE_OUTER_BOUND('',#6033,.T.);
#3865=FACE_OUTER_BOUND('',#6034,.T.);
#3866=FACE_OUTER_BOUND('',#6035,.T.);
#3867=FACE_OUTER_BOUND('',#6036,.T.);
#3868=FACE_OUTER_BOUND('',#6037,.T.);
#3869=FACE_OUTER_BOUND('',#6039,.T.);
#3870=FACE_OUTER_BOUND('',#6040,.T.);
#3871=FACE_OUTER_BOUND('',#6041,.T.);
#3872=FACE_OUTER_BOUND('',#6042,.T.);
#3873=FACE_OUTER_BOUND('',#6043,.T.);
#3874=FACE_OUTER_BOUND('',#6044,.T.);
#3875=FACE_OUTER_BOUND('',#6045,.T.);
#3876=FACE_OUTER_BOUND('',#6046,.T.);
#3877=FACE_OUTER_BOUND('',#6047,.T.);
#3878=FACE_OUTER_BOUND('',#6048,.T.);
#3879=FACE_OUTER_BOUND('',#6049,.T.);
#3880=FACE_OUTER_BOUND('',#6050,.T.);
#3881=FACE_OUTER_BOUND('',#6052,.T.);
#3882=FACE_OUTER_BOUND('',#6053,.T.);
#3883=FACE_OUTER_BOUND('',#6054,.T.);
#3884=FACE_OUTER_BOUND('',#6055,.T.);
#3885=FACE_OUTER_BOUND('',#6056,.T.);
#3886=FACE_OUTER_BOUND('',#6057,.T.);
#3887=FACE_OUTER_BOUND('',#6058,.T.);
#3888=FACE_OUTER_BOUND('',#6059,.T.);
#3889=FACE_OUTER_BOUND('',#6060,.T.);
#3890=FACE_OUTER_BOUND('',#6061,.T.);
#3891=FACE_OUTER_BOUND('',#6062,.T.);
#3892=FACE_OUTER_BOUND('',#6063,.T.);
#3893=FACE_OUTER_BOUND('',#6064,.T.);
#3894=FACE_OUTER_BOUND('',#6065,.T.);
#3895=FACE_OUTER_BOUND('',#6066,.T.);
#3896=FACE_OUTER_BOUND('',#6067,.T.);
#3897=FACE_OUTER_BOUND('',#6068,.T.);
#3898=FACE_OUTER_BOUND('',#6069,.T.);
#3899=FACE_OUTER_BOUND('',#6071,.T.);
#3900=FACE_OUTER_BOUND('',#6073,.T.);
#3901=FACE_OUTER_BOUND('',#6075,.T.);
#3902=FACE_OUTER_BOUND('',#6076,.T.);
#3903=FACE_OUTER_BOUND('',#6077,.T.);
#3904=FACE_OUTER_BOUND('',#6078,.T.);
#3905=FACE_OUTER_BOUND('',#6079,.T.);
#3906=FACE_OUTER_BOUND('',#6080,.T.);
#3907=FACE_OUTER_BOUND('',#6081,.T.);
#3908=FACE_OUTER_BOUND('',#6082,.T.);
#3909=FACE_OUTER_BOUND('',#6083,.T.);
#3910=FACE_OUTER_BOUND('',#6084,.T.);
#3911=FACE_OUTER_BOUND('',#6085,.T.);
#3912=FACE_OUTER_BOUND('',#6086,.T.);
#3913=FACE_OUTER_BOUND('',#6087,.T.);
#3914=FACE_OUTER_BOUND('',#6088,.T.);
#3915=FACE_OUTER_BOUND('',#6089,.T.);
#3916=FACE_OUTER_BOUND('',#6090,.T.);
#3917=FACE_OUTER_BOUND('',#6091,.T.);
#3918=FACE_OUTER_BOUND('',#6092,.T.);
#3919=FACE_OUTER_BOUND('',#6093,.T.);
#3920=FACE_OUTER_BOUND('',#6094,.T.);
#3921=FACE_OUTER_BOUND('',#6095,.T.);
#3922=FACE_OUTER_BOUND('',#6096,.T.);
#3923=FACE_OUTER_BOUND('',#6097,.T.);
#3924=FACE_OUTER_BOUND('',#6098,.T.);
#3925=FACE_OUTER_BOUND('',#6099,.T.);
#3926=FACE_OUTER_BOUND('',#6100,.T.);
#3927=FACE_OUTER_BOUND('',#6101,.T.);
#3928=FACE_OUTER_BOUND('',#6102,.T.);
#3929=FACE_OUTER_BOUND('',#6103,.T.);
#3930=FACE_OUTER_BOUND('',#6104,.T.);
#3931=FACE_OUTER_BOUND('',#6105,.T.);
#3932=FACE_OUTER_BOUND('',#6106,.T.);
#3933=FACE_OUTER_BOUND('',#6107,.T.);
#3934=FACE_OUTER_BOUND('',#6108,.T.);
#3935=FACE_OUTER_BOUND('',#6109,.T.);
#3936=FACE_OUTER_BOUND('',#6110,.T.);
#3937=FACE_OUTER_BOUND('',#6111,.T.);
#3938=FACE_OUTER_BOUND('',#6112,.T.);
#3939=FACE_OUTER_BOUND('',#6113,.T.);
#3940=FACE_OUTER_BOUND('',#6117,.T.);
#3941=FACE_OUTER_BOUND('',#6118,.T.);
#3942=FACE_OUTER_BOUND('',#6119,.T.);
#3943=FACE_OUTER_BOUND('',#6120,.T.);
#3944=FACE_OUTER_BOUND('',#6122,.T.);
#3945=FACE_OUTER_BOUND('',#6123,.T.);
#3946=FACE_OUTER_BOUND('',#6124,.T.);
#3947=FACE_OUTER_BOUND('',#6125,.T.);
#3948=FACE_OUTER_BOUND('',#6126,.T.);
#3949=FACE_OUTER_BOUND('',#6127,.T.);
#3950=FACE_OUTER_BOUND('',#6128,.T.);
#3951=FACE_OUTER_BOUND('',#6129,.T.);
#3952=FACE_OUTER_BOUND('',#6130,.T.);
#3953=FACE_OUTER_BOUND('',#6131,.T.);
#3954=FACE_OUTER_BOUND('',#6132,.T.);
#3955=FACE_OUTER_BOUND('',#6133,.T.);
#3956=FACE_OUTER_BOUND('',#6134,.T.);
#3957=FACE_OUTER_BOUND('',#6135,.T.);
#3958=FACE_OUTER_BOUND('',#6136,.T.);
#3959=FACE_OUTER_BOUND('',#6137,.T.);
#3960=FACE_OUTER_BOUND('',#6138,.T.);
#3961=FACE_OUTER_BOUND('',#6139,.T.);
#3962=FACE_OUTER_BOUND('',#6140,.T.);
#3963=FACE_OUTER_BOUND('',#6141,.T.);
#3964=FACE_OUTER_BOUND('',#6142,.T.);
#3965=FACE_OUTER_BOUND('',#6143,.T.);
#3966=FACE_OUTER_BOUND('',#6144,.T.);
#3967=FACE_OUTER_BOUND('',#6145,.T.);
#3968=FACE_OUTER_BOUND('',#6146,.T.);
#3969=FACE_OUTER_BOUND('',#6147,.T.);
#3970=FACE_OUTER_BOUND('',#6148,.T.);
#3971=FACE_OUTER_BOUND('',#6149,.T.);
#3972=FACE_OUTER_BOUND('',#6150,.T.);
#3973=FACE_OUTER_BOUND('',#6151,.T.);
#3974=FACE_OUTER_BOUND('',#6152,.T.);
#3975=FACE_OUTER_BOUND('',#6153,.T.);
#3976=FACE_OUTER_BOUND('',#6154,.T.);
#3977=FACE_OUTER_BOUND('',#6155,.T.);
#3978=FACE_OUTER_BOUND('',#6156,.T.);
#3979=FACE_OUTER_BOUND('',#6157,.T.);
#3980=FACE_OUTER_BOUND('',#6158,.T.);
#3981=FACE_OUTER_BOUND('',#6159,.T.);
#3982=FACE_OUTER_BOUND('',#6160,.T.);
#3983=FACE_OUTER_BOUND('',#6161,.T.);
#3984=FACE_OUTER_BOUND('',#6162,.T.);
#3985=FACE_OUTER_BOUND('',#6163,.T.);
#3986=FACE_OUTER_BOUND('',#6164,.T.);
#3987=FACE_OUTER_BOUND('',#6165,.T.);
#3988=FACE_OUTER_BOUND('',#6166,.T.);
#3989=FACE_OUTER_BOUND('',#6167,.T.);
#3990=FACE_OUTER_BOUND('',#6168,.T.);
#3991=FACE_OUTER_BOUND('',#6169,.T.);
#3992=FACE_OUTER_BOUND('',#6171,.T.);
#3993=FACE_OUTER_BOUND('',#6173,.T.);
#3994=FACE_OUTER_BOUND('',#6174,.T.);
#3995=FACE_OUTER_BOUND('',#6175,.T.);
#3996=FACE_OUTER_BOUND('',#6176,.T.);
#3997=FACE_OUTER_BOUND('',#6177,.T.);
#3998=FACE_OUTER_BOUND('',#6178,.T.);
#3999=FACE_OUTER_BOUND('',#6179,.T.);
#4000=FACE_OUTER_BOUND('',#6180,.T.);
#4001=FACE_OUTER_BOUND('',#6181,.T.);
#4002=FACE_OUTER_BOUND('',#6182,.T.);
#4003=FACE_OUTER_BOUND('',#6183,.T.);
#4004=FACE_OUTER_BOUND('',#6184,.T.);
#4005=FACE_OUTER_BOUND('',#6185,.T.);
#4006=FACE_OUTER_BOUND('',#6186,.T.);
#4007=FACE_OUTER_BOUND('',#6187,.T.);
#4008=FACE_OUTER_BOUND('',#6189,.T.);
#4009=FACE_OUTER_BOUND('',#6190,.T.);
#4010=FACE_OUTER_BOUND('',#6191,.T.);
#4011=FACE_OUTER_BOUND('',#6192,.T.);
#4012=FACE_OUTER_BOUND('',#6193,.T.);
#4013=FACE_OUTER_BOUND('',#6194,.T.);
#4014=FACE_OUTER_BOUND('',#6195,.T.);
#4015=FACE_OUTER_BOUND('',#6196,.T.);
#4016=FACE_OUTER_BOUND('',#6197,.T.);
#4017=FACE_OUTER_BOUND('',#6198,.T.);
#4018=FACE_OUTER_BOUND('',#6199,.T.);
#4019=FACE_OUTER_BOUND('',#6200,.T.);
#4020=FACE_OUTER_BOUND('',#6201,.T.);
#4021=FACE_OUTER_BOUND('',#6202,.T.);
#4022=FACE_OUTER_BOUND('',#6203,.T.);
#4023=FACE_OUTER_BOUND('',#6204,.T.);
#4024=FACE_OUTER_BOUND('',#6205,.T.);
#4025=FACE_OUTER_BOUND('',#6206,.T.);
#4026=FACE_OUTER_BOUND('',#6207,.T.);
#4027=FACE_OUTER_BOUND('',#6208,.T.);
#4028=FACE_OUTER_BOUND('',#6209,.T.);
#4029=FACE_OUTER_BOUND('',#6210,.T.);
#4030=FACE_OUTER_BOUND('',#6211,.T.);
#4031=FACE_OUTER_BOUND('',#6212,.T.);
#4032=FACE_OUTER_BOUND('',#6213,.T.);
#4033=FACE_OUTER_BOUND('',#6214,.T.);
#4034=FACE_OUTER_BOUND('',#6215,.T.);
#4035=FACE_OUTER_BOUND('',#6216,.T.);
#4036=FACE_OUTER_BOUND('',#6217,.T.);
#4037=FACE_OUTER_BOUND('',#6218,.T.);
#4038=FACE_OUTER_BOUND('',#6219,.T.);
#4039=FACE_OUTER_BOUND('',#6220,.T.);
#4040=FACE_OUTER_BOUND('',#6221,.T.);
#4041=FACE_OUTER_BOUND('',#6222,.T.);
#4042=FACE_OUTER_BOUND('',#6223,.T.);
#4043=FACE_OUTER_BOUND('',#6224,.T.);
#4044=FACE_OUTER_BOUND('',#6225,.T.);
#4045=FACE_OUTER_BOUND('',#6226,.T.);
#4046=FACE_OUTER_BOUND('',#6227,.T.);
#4047=FACE_OUTER_BOUND('',#6228,.T.);
#4048=FACE_OUTER_BOUND('',#6229,.T.);
#4049=FACE_OUTER_BOUND('',#6230,.T.);
#4050=FACE_OUTER_BOUND('',#6231,.T.);
#4051=FACE_OUTER_BOUND('',#6232,.T.);
#4052=FACE_OUTER_BOUND('',#6233,.T.);
#4053=FACE_OUTER_BOUND('',#6234,.T.);
#4054=FACE_OUTER_BOUND('',#6235,.T.);
#4055=FACE_OUTER_BOUND('',#6236,.T.);
#4056=FACE_OUTER_BOUND('',#6237,.T.);
#4057=FACE_OUTER_BOUND('',#6238,.T.);
#4058=FACE_OUTER_BOUND('',#6239,.T.);
#4059=FACE_OUTER_BOUND('',#6240,.T.);
#4060=FACE_OUTER_BOUND('',#6241,.T.);
#4061=FACE_OUTER_BOUND('',#6242,.T.);
#4062=FACE_OUTER_BOUND('',#6243,.T.);
#4063=FACE_OUTER_BOUND('',#6244,.T.);
#4064=FACE_OUTER_BOUND('',#6245,.T.);
#4065=FACE_OUTER_BOUND('',#6246,.T.);
#4066=FACE_OUTER_BOUND('',#6247,.T.);
#4067=FACE_OUTER_BOUND('',#6248,.T.);
#4068=FACE_OUTER_BOUND('',#6249,.T.);
#4069=FACE_OUTER_BOUND('',#6250,.T.);
#4070=FACE_OUTER_BOUND('',#6251,.T.);
#4071=FACE_OUTER_BOUND('',#6252,.T.);
#4072=FACE_OUTER_BOUND('',#6253,.T.);
#4073=FACE_OUTER_BOUND('',#6254,.T.);
#4074=FACE_OUTER_BOUND('',#6255,.T.);
#4075=FACE_OUTER_BOUND('',#6256,.T.);
#4076=FACE_OUTER_BOUND('',#6257,.T.);
#4077=FACE_OUTER_BOUND('',#6258,.T.);
#4078=FACE_OUTER_BOUND('',#6259,.T.);
#4079=FACE_OUTER_BOUND('',#6260,.T.);
#4080=FACE_OUTER_BOUND('',#6261,.T.);
#4081=FACE_OUTER_BOUND('',#6262,.T.);
#4082=FACE_OUTER_BOUND('',#6263,.T.);
#4083=FACE_OUTER_BOUND('',#6264,.T.);
#4084=FACE_OUTER_BOUND('',#6265,.T.);
#4085=FACE_OUTER_BOUND('',#6266,.T.);
#4086=FACE_OUTER_BOUND('',#6267,.T.);
#4087=FACE_OUTER_BOUND('',#6268,.T.);
#4088=FACE_OUTER_BOUND('',#6269,.T.);
#4089=FACE_OUTER_BOUND('',#6270,.T.);
#4090=FACE_OUTER_BOUND('',#6271,.T.);
#4091=FACE_OUTER_BOUND('',#6272,.T.);
#4092=FACE_OUTER_BOUND('',#6273,.T.);
#4093=FACE_OUTER_BOUND('',#6274,.T.);
#4094=FACE_OUTER_BOUND('',#6275,.T.);
#4095=FACE_OUTER_BOUND('',#6276,.T.);
#4096=FACE_OUTER_BOUND('',#6277,.T.);
#4097=FACE_OUTER_BOUND('',#6278,.T.);
#4098=FACE_OUTER_BOUND('',#6279,.T.);
#4099=FACE_OUTER_BOUND('',#6280,.T.);
#4100=FACE_OUTER_BOUND('',#6281,.T.);
#4101=FACE_OUTER_BOUND('',#6282,.T.);
#4102=FACE_OUTER_BOUND('',#6283,.T.);
#4103=FACE_OUTER_BOUND('',#6284,.T.);
#4104=FACE_OUTER_BOUND('',#6285,.T.);
#4105=FACE_OUTER_BOUND('',#6286,.T.);
#4106=FACE_OUTER_BOUND('',#6287,.T.);
#4107=FACE_OUTER_BOUND('',#6288,.T.);
#4108=FACE_OUTER_BOUND('',#6289,.T.);
#4109=FACE_OUTER_BOUND('',#6290,.T.);
#4110=FACE_OUTER_BOUND('',#6291,.T.);
#4111=FACE_OUTER_BOUND('',#6292,.T.);
#4112=FACE_OUTER_BOUND('',#6293,.T.);
#4113=FACE_OUTER_BOUND('',#6294,.T.);
#4114=FACE_OUTER_BOUND('',#6295,.T.);
#4115=FACE_OUTER_BOUND('',#6296,.T.);
#4116=FACE_OUTER_BOUND('',#6297,.T.);
#4117=FACE_OUTER_BOUND('',#6298,.T.);
#4118=FACE_OUTER_BOUND('',#6299,.T.);
#4119=FACE_OUTER_BOUND('',#6300,.T.);
#4120=FACE_OUTER_BOUND('',#6301,.T.);
#4121=FACE_OUTER_BOUND('',#6302,.T.);
#4122=FACE_OUTER_BOUND('',#6303,.T.);
#4123=FACE_OUTER_BOUND('',#6304,.T.);
#4124=FACE_OUTER_BOUND('',#6305,.T.);
#4125=FACE_OUTER_BOUND('',#6306,.T.);
#5889=EDGE_LOOP('',(#23937,#23938,#23939));
#5890=EDGE_LOOP('',(#23940,#23941,#23942,#23943));
#5891=EDGE_LOOP('',(#23944,#23945,#23946,#23947));
#5892=EDGE_LOOP('',(#23948,#23949,#23950,#23951));
#5893=EDGE_LOOP('',(#23952,#23953,#23954));
#5894=EDGE_LOOP('',(#23955,#23956,#23957));
#5895=EDGE_LOOP('',(#23958,#23959,#23960,#23961));
#5896=EDGE_LOOP('',(#23962,#23963,#23964,#23965));
#5897=EDGE_LOOP('',(#23966,#23967,#23968,#23969));
#5898=EDGE_LOOP('',(#23970,#23971,#23972));
#5899=EDGE_LOOP('',(#23973,#23974,#23975,#23976,#23977));
#5900=EDGE_LOOP('',(#23978,#23979,#23980,#23981));
#5901=EDGE_LOOP('',(#23982,#23983,#23984,#23985,#23986));
#5902=EDGE_LOOP('',(#23987,#23988,#23989,#23990,#23991,#23992,#23993,#23994,
#23995,#23996,#23997,#23998,#23999,#24000,#24001,#24002));
#5903=EDGE_LOOP('',(#24003,#24004,#24005,#24006,#24007,#24008));
#5904=EDGE_LOOP('',(#24009,#24010,#24011,#24012,#24013,#24014,#24015));
#5905=EDGE_LOOP('',(#24016,#24017,#24018,#24019,#24020,#24021,#24022));
#5906=EDGE_LOOP('',(#24023,#24024,#24025,#24026,#24027,#24028,#24029));
#5907=EDGE_LOOP('',(#24030,#24031,#24032,#24033,#24034,#24035,#24036,#24037,
#24038,#24039));
#5908=EDGE_LOOP('',(#24040,#24041,#24042,#24043,#24044,#24045,#24046));
#5909=EDGE_LOOP('',(#24047,#24048,#24049,#24050));
#5910=EDGE_LOOP('',(#24051,#24052,#24053,#24054));
#5911=EDGE_LOOP('',(#24055,#24056,#24057,#24058,#24059,#24060,#24061,#24062));
#5912=EDGE_LOOP('',(#24063,#24064,#24065,#24066,#24067));
#5913=EDGE_LOOP('',(#24068,#24069,#24070,#24071,#24072,#24073,#24074,#24075,
#24076,#24077,#24078,#24079,#24080,#24081,#24082,#24083,#24084,#24085,#24086,
#24087));
#5914=EDGE_LOOP('',(#24088,#24089,#24090,#24091));
#5915=EDGE_LOOP('',(#24092,#24093,#24094,#24095));
#5916=EDGE_LOOP('',(#24096,#24097,#24098,#24099));
#5917=EDGE_LOOP('',(#24100,#24101,#24102,#24103,#24104,#24105,#24106,#24107,
#24108,#24109));
#5918=EDGE_LOOP('',(#24110,#24111,#24112,#24113));
#5919=EDGE_LOOP('',(#24114,#24115,#24116,#24117));
#5920=EDGE_LOOP('',(#24118,#24119,#24120,#24121));
#5921=EDGE_LOOP('',(#24122,#24123,#24124,#24125,#24126,#24127,#24128,#24129,
#24130,#24131,#24132,#24133,#24134,#24135,#24136,#24137,#24138,#24139,#24140,
#24141));
#5922=EDGE_LOOP('',(#24142,#24143,#24144,#24145));
#5923=EDGE_LOOP('',(#24146,#24147,#24148,#24149));
#5924=EDGE_LOOP('',(#24150,#24151,#24152,#24153));
#5925=EDGE_LOOP('',(#24154,#24155,#24156,#24157,#24158,#24159,#24160,#24161,
#24162,#24163));
#5926=EDGE_LOOP('',(#24164,#24165,#24166,#24167));
#5927=EDGE_LOOP('',(#24168,#24169,#24170,#24171));
#5928=EDGE_LOOP('',(#24172,#24173,#24174,#24175));
#5929=EDGE_LOOP('',(#24176,#24177,#24178,#24179,#24180,#24181));
#5930=EDGE_LOOP('',(#24182,#24183,#24184,#24185,#24186));
#5931=EDGE_LOOP('',(#24187,#24188,#24189,#24190,#24191,#24192,#24193));
#5932=EDGE_LOOP('',(#24194,#24195,#24196,#24197));
#5933=EDGE_LOOP('',(#24198,#24199,#24200,#24201,#24202,#24203,#24204));
#5934=EDGE_LOOP('',(#24205,#24206,#24207,#24208,#24209));
#5935=EDGE_LOOP('',(#24210,#24211,#24212,#24213,#24214));
#5936=EDGE_LOOP('',(#24215,#24216,#24217,#24218,#24219));
#5937=EDGE_LOOP('',(#24220,#24221,#24222,#24223));
#5938=EDGE_LOOP('',(#24224,#24225,#24226,#24227,#24228));
#5939=EDGE_LOOP('',(#24229,#24230,#24231,#24232));
#5940=EDGE_LOOP('',(#24233,#24234,#24235,#24236,#24237));
#5941=EDGE_LOOP('',(#24238,#24239,#24240,#24241));
#5942=EDGE_LOOP('',(#24242,#24243,#24244,#24245));
#5943=EDGE_LOOP('',(#24246,#24247,#24248,#24249,#24250));
#5944=EDGE_LOOP('',(#24251,#24252,#24253,#24254));
#5945=EDGE_LOOP('',(#24255,#24256,#24257,#24258,#24259));
#5946=EDGE_LOOP('',(#24260,#24261,#24262,#24263));
#5947=EDGE_LOOP('',(#24264,#24265,#24266,#24267));
#5948=EDGE_LOOP('',(#24268,#24269,#24270,#24271,#24272));
#5949=EDGE_LOOP('',(#24273,#24274,#24275,#24276,#24277));
#5950=EDGE_LOOP('',(#24278,#24279,#24280,#24281));
#5951=EDGE_LOOP('',(#24282,#24283,#24284,#24285));
#5952=EDGE_LOOP('',(#24286,#24287,#24288,#24289,#24290,#24291,#24292,#24293,
#24294,#24295));
#5953=EDGE_LOOP('',(#24296,#24297,#24298,#24299));
#5954=EDGE_LOOP('',(#24300,#24301,#24302,#24303));
#5955=EDGE_LOOP('',(#24304,#24305,#24306,#24307));
#5956=EDGE_LOOP('',(#24308,#24309,#24310,#24311));
#5957=EDGE_LOOP('',(#24312,#24313,#24314,#24315));
#5958=EDGE_LOOP('',(#24316,#24317,#24318,#24319));
#5959=EDGE_LOOP('',(#24320,#24321,#24322,#24323));
#5960=EDGE_LOOP('',(#24324,#24325,#24326,#24327));
#5961=EDGE_LOOP('',(#24328,#24329,#24330,#24331));
#5962=EDGE_LOOP('',(#24332,#24333,#24334,#24335));
#5963=EDGE_LOOP('',(#24336,#24337,#24338,#24339));
#5964=EDGE_LOOP('',(#24340,#24341,#24342,#24343,#24344));
#5965=EDGE_LOOP('',(#24345,#24346,#24347,#24348,#24349));
#5966=EDGE_LOOP('',(#24350,#24351,#24352,#24353));
#5967=EDGE_LOOP('',(#24354,#24355,#24356,#24357));
#5968=EDGE_LOOP('',(#24358,#24359,#24360,#24361,#24362,#24363,#24364,#24365,
#24366,#24367,#24368));
#5969=EDGE_LOOP('',(#24369,#24370,#24371,#24372,#24373));
#5970=EDGE_LOOP('',(#24374,#24375,#24376,#24377,#24378,#24379));
#5971=EDGE_LOOP('',(#24380,#24381,#24382,#24383,#24384));
#5972=EDGE_LOOP('',(#24385,#24386,#24387,#24388,#24389,#24390,#24391,#24392));
#5973=EDGE_LOOP('',(#24393,#24394,#24395,#24396));
#5974=EDGE_LOOP('',(#24397,#24398,#24399,#24400,#24401,#24402,#24403,#24404));
#5975=EDGE_LOOP('',(#24405,#24406,#24407,#24408,#24409));
#5976=EDGE_LOOP('',(#24410,#24411,#24412,#24413,#24414,#24415));
#5977=EDGE_LOOP('',(#24416,#24417,#24418,#24419,#24420,#24421));
#5978=EDGE_LOOP('',(#24422,#24423,#24424,#24425,#24426));
#5979=EDGE_LOOP('',(#24427,#24428,#24429,#24430,#24431,#24432));
#5980=EDGE_LOOP('',(#24433,#24434,#24435,#24436,#24437));
#5981=EDGE_LOOP('',(#24438,#24439,#24440,#24441,#24442,#24443,#24444,#24445));
#5982=EDGE_LOOP('',(#24446,#24447,#24448,#24449));
#5983=EDGE_LOOP('',(#24450,#24451,#24452,#24453,#24454,#24455,#24456,#24457));
#5984=EDGE_LOOP('',(#24458,#24459,#24460,#24461));
#5985=EDGE_LOOP('',(#24462,#24463,#24464,#24465));
#5986=EDGE_LOOP('',(#24466,#24467,#24468,#24469));
#5987=EDGE_LOOP('',(#24470,#24471,#24472,#24473));
#5988=EDGE_LOOP('',(#24474,#24475,#24476,#24477,#24478,#24479,#24480,#24481,
#24482,#24483,#24484,#24485));
#5989=EDGE_LOOP('',(#24486,#24487,#24488,#24489));
#5990=EDGE_LOOP('',(#24490,#24491,#24492,#24493,#24494,#24495,#24496,#24497,
#24498,#24499,#24500,#24501));
#5991=EDGE_LOOP('',(#24502,#24503,#24504));
#5992=EDGE_LOOP('',(#24505,#24506,#24507));
#5993=EDGE_LOOP('',(#24508,#24509,#24510,#24511,#24512));
#5994=EDGE_LOOP('',(#24513,#24514,#24515,#24516,#24517,#24518,#24519,#24520));
#5995=EDGE_LOOP('',(#24521,#24522,#24523,#24524));
#5996=EDGE_LOOP('',(#24525,#24526,#24527,#24528,#24529,#24530));
#5997=EDGE_LOOP('',(#24531,#24532,#24533,#24534,#24535,#24536));
#5998=EDGE_LOOP('',(#24537,#24538,#24539,#24540,#24541,#24542));
#5999=EDGE_LOOP('',(#24543,#24544,#24545,#24546));
#6000=EDGE_LOOP('',(#24547,#24548,#24549,#24550,#24551,#24552,#24553,#24554,
#24555,#24556));
#6001=EDGE_LOOP('',(#24557,#24558,#24559,#24560,#24561,#24562,#24563,#24564,
#24565));
#6002=EDGE_LOOP('',(#24566));
#6003=EDGE_LOOP('',(#24567));
#6004=EDGE_LOOP('',(#24568,#24569,#24570,#24571,#24572,#24573));
#6005=EDGE_LOOP('',(#24574,#24575,#24576,#24577,#24578,#24579));
#6006=EDGE_LOOP('',(#24580,#24581,#24582,#24583,#24584,#24585));
#6007=EDGE_LOOP('',(#24586,#24587,#24588,#24589,#24590));
#6008=EDGE_LOOP('',(#24591,#24592,#24593,#24594));
#6009=EDGE_LOOP('',(#24595,#24596,#24597,#24598,#24599,#24600));
#6010=EDGE_LOOP('',(#24601,#24602,#24603,#24604));
#6011=EDGE_LOOP('',(#24605,#24606,#24607,#24608));
#6012=EDGE_LOOP('',(#24609,#24610,#24611,#24612));
#6013=EDGE_LOOP('',(#24613,#24614,#24615,#24616));
#6014=EDGE_LOOP('',(#24617,#24618,#24619,#24620));
#6015=EDGE_LOOP('',(#24621,#24622,#24623,#24624));
#6016=EDGE_LOOP('',(#24625,#24626,#24627,#24628));
#6017=EDGE_LOOP('',(#24629,#24630,#24631,#24632));
#6018=EDGE_LOOP('',(#24633,#24634,#24635,#24636));
#6019=EDGE_LOOP('',(#24637,#24638,#24639,#24640,#24641));
#6020=EDGE_LOOP('',(#24642,#24643,#24644,#24645,#24646,#24647));
#6021=EDGE_LOOP('',(#24648,#24649,#24650,#24651,#24652,#24653,#24654,#24655,
#24656,#24657,#24658,#24659,#24660,#24661,#24662,#24663,#24664,#24665,#24666,
#24667,#24668,#24669,#24670,#24671,#24672,#24673));
#6022=EDGE_LOOP('',(#24674,#24675,#24676,#24677));
#6023=EDGE_LOOP('',(#24678,#24679,#24680,#24681));
#6024=EDGE_LOOP('',(#24682,#24683,#24684,#24685));
#6025=EDGE_LOOP('',(#24686,#24687,#24688,#24689));
#6026=EDGE_LOOP('',(#24690,#24691,#24692,#24693));
#6027=EDGE_LOOP('',(#24694,#24695,#24696,#24697));
#6028=EDGE_LOOP('',(#24698,#24699,#24700,#24701,#24702,#24703));
#6029=EDGE_LOOP('',(#24704,#24705,#24706,#24707));
#6030=EDGE_LOOP('',(#24708,#24709,#24710,#24711));
#6031=EDGE_LOOP('',(#24712,#24713,#24714,#24715));
#6032=EDGE_LOOP('',(#24716,#24717,#24718,#24719));
#6033=EDGE_LOOP('',(#24720,#24721,#24722,#24723));
#6034=EDGE_LOOP('',(#24724,#24725,#24726,#24727,#24728));
#6035=EDGE_LOOP('',(#24729,#24730,#24731,#24732,#24733,#24734));
#6036=EDGE_LOOP('',(#24735,#24736,#24737,#24738,#24739,#24740,#24741,#24742,
#24743,#24744,#24745,#24746,#24747,#24748,#24749,#24750,#24751,#24752,#24753,
#24754,#24755,#24756,#24757,#24758,#24759,#24760));
#6037=EDGE_LOOP('',(#24761));
#6038=EDGE_LOOP('',(#24762));
#6039=EDGE_LOOP('',(#24763,#24764,#24765,#24766));
#6040=EDGE_LOOP('',(#24767,#24768,#24769,#24770));
#6041=EDGE_LOOP('',(#24771,#24772,#24773,#24774));
#6042=EDGE_LOOP('',(#24775,#24776,#24777,#24778));
#6043=EDGE_LOOP('',(#24779,#24780,#24781,#24782));
#6044=EDGE_LOOP('',(#24783,#24784,#24785,#24786));
#6045=EDGE_LOOP('',(#24787,#24788,#24789,#24790));
#6046=EDGE_LOOP('',(#24791,#24792,#24793,#24794));
#6047=EDGE_LOOP('',(#24795,#24796,#24797,#24798));
#6048=EDGE_LOOP('',(#24799,#24800,#24801,#24802));
#6049=EDGE_LOOP('',(#24803,#24804,#24805,#24806));
#6050=EDGE_LOOP('',(#24807));
#6051=EDGE_LOOP('',(#24808));
#6052=EDGE_LOOP('',(#24809,#24810,#24811,#24812));
#6053=EDGE_LOOP('',(#24813,#24814,#24815,#24816));
#6054=EDGE_LOOP('',(#24817,#24818,#24819,#24820));
#6055=EDGE_LOOP('',(#24821,#24822,#24823,#24824));
#6056=EDGE_LOOP('',(#24825,#24826,#24827,#24828));
#6057=EDGE_LOOP('',(#24829,#24830,#24831,#24832));
#6058=EDGE_LOOP('',(#24833,#24834,#24835,#24836));
#6059=EDGE_LOOP('',(#24837,#24838,#24839,#24840));
#6060=EDGE_LOOP('',(#24841,#24842,#24843,#24844));
#6061=EDGE_LOOP('',(#24845,#24846,#24847,#24848));
#6062=EDGE_LOOP('',(#24849,#24850,#24851,#24852));
#6063=EDGE_LOOP('',(#24853,#24854,#24855,#24856));
#6064=EDGE_LOOP('',(#24857,#24858,#24859,#24860));
#6065=EDGE_LOOP('',(#24861,#24862,#24863,#24864));
#6066=EDGE_LOOP('',(#24865,#24866,#24867,#24868));
#6067=EDGE_LOOP('',(#24869,#24870,#24871,#24872));
#6068=EDGE_LOOP('',(#24873,#24874,#24875,#24876));
#6069=EDGE_LOOP('',(#24877,#24878,#24879,#24880,#24881,#24882,#24883,#24884,
#24885));
#6070=EDGE_LOOP('',(#24886,#24887,#24888,#24889,#24890,#24891));
#6071=EDGE_LOOP('',(#24892));
#6072=EDGE_LOOP('',(#24893));
#6073=EDGE_LOOP('',(#24894));
#6074=EDGE_LOOP('',(#24895));
#6075=EDGE_LOOP('',(#24896,#24897,#24898,#24899));
#6076=EDGE_LOOP('',(#24900));
#6077=EDGE_LOOP('',(#24901,#24902,#24903,#24904,#24905));
#6078=EDGE_LOOP('',(#24906,#24907,#24908,#24909,#24910,#24911));
#6079=EDGE_LOOP('',(#24912,#24913,#24914,#24915,#24916));
#6080=EDGE_LOOP('',(#24917,#24918,#24919,#24920,#24921));
#6081=EDGE_LOOP('',(#24922,#24923,#24924,#24925,#24926,#24927));
#6082=EDGE_LOOP('',(#24928,#24929,#24930,#24931,#24932,#24933,#24934,#24935,
#24936,#24937));
#6083=EDGE_LOOP('',(#24938,#24939,#24940,#24941,#24942,#24943,#24944,#24945,
#24946,#24947));
#6084=EDGE_LOOP('',(#24948));
#6085=EDGE_LOOP('',(#24949,#24950,#24951,#24952));
#6086=EDGE_LOOP('',(#24953,#24954,#24955,#24956));
#6087=EDGE_LOOP('',(#24957,#24958,#24959,#24960));
#6088=EDGE_LOOP('',(#24961,#24962,#24963,#24964));
#6089=EDGE_LOOP('',(#24965,#24966,#24967,#24968));
#6090=EDGE_LOOP('',(#24969,#24970,#24971,#24972));
#6091=EDGE_LOOP('',(#24973,#24974,#24975,#24976));
#6092=EDGE_LOOP('',(#24977,#24978,#24979,#24980));
#6093=EDGE_LOOP('',(#24981,#24982,#24983,#24984));
#6094=EDGE_LOOP('',(#24985,#24986,#24987,#24988));
#6095=EDGE_LOOP('',(#24989,#24990,#24991,#24992));
#6096=EDGE_LOOP('',(#24993,#24994,#24995,#24996));
#6097=EDGE_LOOP('',(#24997,#24998,#24999,#25000,#25001,#25002,#25003,#25004,
#25005,#25006));
#6098=EDGE_LOOP('',(#25007,#25008,#25009));
#6099=EDGE_LOOP('',(#25010,#25011,#25012,#25013,#25014,#25015,#25016));
#6100=EDGE_LOOP('',(#25017,#25018,#25019,#25020,#25021,#25022,#25023));
#6101=EDGE_LOOP('',(#25024,#25025,#25026));
#6102=EDGE_LOOP('',(#25027,#25028,#25029,#25030,#25031,#25032,#25033));
#6103=EDGE_LOOP('',(#25034,#25035,#25036,#25037,#25038,#25039,#25040,#25041));
#6104=EDGE_LOOP('',(#25042,#25043,#25044,#25045));
#6105=EDGE_LOOP('',(#25046,#25047,#25048,#25049,#25050,#25051));
#6106=EDGE_LOOP('',(#25052,#25053,#25054));
#6107=EDGE_LOOP('',(#25055,#25056,#25057,#25058,#25059,#25060));
#6108=EDGE_LOOP('',(#25061,#25062,#25063));
#6109=EDGE_LOOP('',(#25064,#25065,#25066,#25067,#25068,#25069));
#6110=EDGE_LOOP('',(#25070,#25071,#25072,#25073,#25074,#25075,#25076,#25077));
#6111=EDGE_LOOP('',(#25078,#25079,#25080,#25081));
#6112=EDGE_LOOP('',(#25082,#25083,#25084,#25085,#25086,#25087));
#6113=EDGE_LOOP('',(#25088,#25089,#25090,#25091,#25092,#25093,#25094,#25095,
#25096,#25097,#25098));
#6114=EDGE_LOOP('',(#25099,#25100,#25101,#25102,#25103,#25104,#25105,#25106,
#25107));
#6115=EDGE_LOOP('',(#25108,#25109,#25110,#25111,#25112,#25113,#25114));
#6116=EDGE_LOOP('',(#25115,#25116,#25117,#25118,#25119,#25120,#25121,#25122,
#25123));
#6117=EDGE_LOOP('',(#25124,#25125,#25126,#25127));
#6118=EDGE_LOOP('',(#25128,#25129,#25130,#25131));
#6119=EDGE_LOOP('',(#25132,#25133,#25134,#25135));
#6120=EDGE_LOOP('',(#25136,#25137,#25138,#25139,#25140,#25141,#25142));
#6121=EDGE_LOOP('',(#25143,#25144,#25145,#25146,#25147,#25148,#25149));
#6122=EDGE_LOOP('',(#25150,#25151,#25152,#25153));
#6123=EDGE_LOOP('',(#25154,#25155,#25156,#25157));
#6124=EDGE_LOOP('',(#25158,#25159,#25160,#25161,#25162));
#6125=EDGE_LOOP('',(#25163,#25164,#25165,#25166));
#6126=EDGE_LOOP('',(#25167,#25168,#25169,#25170,#25171));
#6127=EDGE_LOOP('',(#25172,#25173,#25174,#25175));
#6128=EDGE_LOOP('',(#25176,#25177,#25178,#25179));
#6129=EDGE_LOOP('',(#25180,#25181,#25182,#25183));
#6130=EDGE_LOOP('',(#25184,#25185,#25186,#25187,#25188,#25189));
#6131=EDGE_LOOP('',(#25190,#25191,#25192,#25193));
#6132=EDGE_LOOP('',(#25194,#25195,#25196,#25197));
#6133=EDGE_LOOP('',(#25198,#25199,#25200,#25201));
#6134=EDGE_LOOP('',(#25202,#25203,#25204,#25205,#25206,#25207));
#6135=EDGE_LOOP('',(#25208,#25209,#25210,#25211,#25212));
#6136=EDGE_LOOP('',(#25213,#25214,#25215,#25216));
#6137=EDGE_LOOP('',(#25217,#25218,#25219,#25220));
#6138=EDGE_LOOP('',(#25221,#25222,#25223,#25224));
#6139=EDGE_LOOP('',(#25225,#25226,#25227,#25228));
#6140=EDGE_LOOP('',(#25229,#25230,#25231,#25232,#25233));
#6141=EDGE_LOOP('',(#25234,#25235,#25236,#25237));
#6142=EDGE_LOOP('',(#25238,#25239,#25240,#25241));
#6143=EDGE_LOOP('',(#25242,#25243,#25244,#25245));
#6144=EDGE_LOOP('',(#25246,#25247,#25248,#25249));
#6145=EDGE_LOOP('',(#25250,#25251,#25252,#25253));
#6146=EDGE_LOOP('',(#25254,#25255,#25256,#25257));
#6147=EDGE_LOOP('',(#25258,#25259,#25260,#25261));
#6148=EDGE_LOOP('',(#25262,#25263,#25264,#25265));
#6149=EDGE_LOOP('',(#25266,#25267,#25268,#25269));
#6150=EDGE_LOOP('',(#25270,#25271,#25272,#25273));
#6151=EDGE_LOOP('',(#25274,#25275,#25276,#25277));
#6152=EDGE_LOOP('',(#25278,#25279,#25280,#25281));
#6153=EDGE_LOOP('',(#25282,#25283,#25284,#25285));
#6154=EDGE_LOOP('',(#25286,#25287,#25288,#25289));
#6155=EDGE_LOOP('',(#25290,#25291,#25292,#25293));
#6156=EDGE_LOOP('',(#25294,#25295,#25296,#25297));
#6157=EDGE_LOOP('',(#25298,#25299,#25300,#25301));
#6158=EDGE_LOOP('',(#25302,#25303,#25304,#25305));
#6159=EDGE_LOOP('',(#25306,#25307,#25308,#25309));
#6160=EDGE_LOOP('',(#25310,#25311,#25312,#25313));
#6161=EDGE_LOOP('',(#25314,#25315,#25316,#25317));
#6162=EDGE_LOOP('',(#25318,#25319,#25320,#25321));
#6163=EDGE_LOOP('',(#25322,#25323,#25324,#25325));
#6164=EDGE_LOOP('',(#25326,#25327,#25328,#25329));
#6165=EDGE_LOOP('',(#25330,#25331,#25332,#25333));
#6166=EDGE_LOOP('',(#25334,#25335,#25336,#25337));
#6167=EDGE_LOOP('',(#25338,#25339,#25340,#25341));
#6168=EDGE_LOOP('',(#25342,#25343,#25344,#25345));
#6169=EDGE_LOOP('',(#25346,#25347,#25348,#25349,#25350,#25351,#25352,#25353,
#25354));
#6170=EDGE_LOOP('',(#25355,#25356,#25357,#25358,#25359,#25360,#25361,#25362,
#25363,#25364));
#6171=EDGE_LOOP('',(#25365,#25366,#25367,#25368,#25369,#25370,#25371,#25372,
#25373));
#6172=EDGE_LOOP('',(#25374,#25375,#25376,#25377,#25378,#25379,#25380,#25381,
#25382,#25383));
#6173=EDGE_LOOP('',(#25384,#25385,#25386,#25387));
#6174=EDGE_LOOP('',(#25388,#25389,#25390,#25391));
#6175=EDGE_LOOP('',(#25392,#25393,#25394,#25395));
#6176=EDGE_LOOP('',(#25396,#25397,#25398,#25399));
#6177=EDGE_LOOP('',(#25400,#25401,#25402,#25403,#25404,#25405));
#6178=EDGE_LOOP('',(#25406,#25407,#25408,#25409,#25410,#25411,#25412,#25413));
#6179=EDGE_LOOP('',(#25414,#25415,#25416,#25417,#25418,#25419,#25420,#25421));
#6180=EDGE_LOOP('',(#25422,#25423,#25424,#25425,#25426,#25427));
#6181=EDGE_LOOP('',(#25428,#25429,#25430,#25431,#25432,#25433));
#6182=EDGE_LOOP('',(#25434,#25435,#25436,#25437,#25438,#25439,#25440,#25441));
#6183=EDGE_LOOP('',(#25442,#25443,#25444,#25445,#25446,#25447,#25448,#25449));
#6184=EDGE_LOOP('',(#25450,#25451,#25452,#25453,#25454,#25455));
#6185=EDGE_LOOP('',(#25456,#25457,#25458,#25459,#25460));
#6186=EDGE_LOOP('',(#25461,#25462,#25463,#25464,#25465));
#6187=EDGE_LOOP('',(#25466,#25467,#25468,#25469,#25470,#25471,#25472,#25473,
#25474,#25475,#25476,#25477,#25478,#25479,#25480,#25481,#25482,#25483,#25484,
#25485,#25486,#25487,#25488,#25489,#25490,#25491,#25492,#25493,#25494,#25495,
#25496,#25497,#25498,#25499,#25500,#25501,#25502,#25503,#25504,#25505,#25506,
#25507,#25508,#25509,#25510,#25511,#25512,#25513,#25514,#25515,#25516,#25517,
#25518,#25519,#25520,#25521,#25522,#25523));
#6188=EDGE_LOOP('',(#25524,#25525,#25526,#25527,#25528,#25529,#25530,#25531,
#25532,#25533,#25534));
#6189=EDGE_LOOP('',(#25535,#25536,#25537,#25538,#25539));
#6190=EDGE_LOOP('',(#25540,#25541,#25542,#25543,#25544));
#6191=EDGE_LOOP('',(#25545,#25546,#25547,#25548));
#6192=EDGE_LOOP('',(#25549,#25550,#25551,#25552));
#6193=EDGE_LOOP('',(#25553,#25554,#25555));
#6194=EDGE_LOOP('',(#25556,#25557,#25558,#25559));
#6195=EDGE_LOOP('',(#25560,#25561,#25562));
#6196=EDGE_LOOP('',(#25563,#25564,#25565,#25566));
#6197=EDGE_LOOP('',(#25567,#25568,#25569,#25570));
#6198=EDGE_LOOP('',(#25571,#25572,#25573));
#6199=EDGE_LOOP('',(#25574,#25575,#25576,#25577,#25578,#25579,#25580,#25581,
#25582,#25583));
#6200=EDGE_LOOP('',(#25584,#25585,#25586,#25587));
#6201=EDGE_LOOP('',(#25588,#25589,#25590));
#6202=EDGE_LOOP('',(#25591,#25592,#25593,#25594));
#6203=EDGE_LOOP('',(#25595,#25596,#25597));
#6204=EDGE_LOOP('',(#25598,#25599,#25600,#25601));
#6205=EDGE_LOOP('',(#25602,#25603,#25604));
#6206=EDGE_LOOP('',(#25605,#25606,#25607,#25608));
#6207=EDGE_LOOP('',(#25609,#25610,#25611,#25612));
#6208=EDGE_LOOP('',(#25613,#25614,#25615,#25616));
#6209=EDGE_LOOP('',(#25617,#25618,#25619,#25620));
#6210=EDGE_LOOP('',(#25621,#25622,#25623,#25624));
#6211=EDGE_LOOP('',(#25625,#25626,#25627,#25628));
#6212=EDGE_LOOP('',(#25629,#25630,#25631,#25632));
#6213=EDGE_LOOP('',(#25633,#25634,#25635,#25636));
#6214=EDGE_LOOP('',(#25637,#25638,#25639,#25640));
#6215=EDGE_LOOP('',(#25641,#25642,#25643,#25644));
#6216=EDGE_LOOP('',(#25645,#25646,#25647,#25648));
#6217=EDGE_LOOP('',(#25649,#25650,#25651,#25652));
#6218=EDGE_LOOP('',(#25653,#25654,#25655,#25656,#25657,#25658));
#6219=EDGE_LOOP('',(#25659,#25660,#25661,#25662));
#6220=EDGE_LOOP('',(#25663,#25664,#25665,#25666));
#6221=EDGE_LOOP('',(#25667,#25668,#25669));
#6222=EDGE_LOOP('',(#25670,#25671,#25672,#25673));
#6223=EDGE_LOOP('',(#25674,#25675,#25676));
#6224=EDGE_LOOP('',(#25677,#25678,#25679,#25680));
#6225=EDGE_LOOP('',(#25681,#25682,#25683,#25684));
#6226=EDGE_LOOP('',(#25685,#25686,#25687));
#6227=EDGE_LOOP('',(#25688,#25689,#25690,#25691,#25692,#25693,#25694,#25695,
#25696,#25697));
#6228=EDGE_LOOP('',(#25698,#25699,#25700,#25701));
#6229=EDGE_LOOP('',(#25702,#25703,#25704));
#6230=EDGE_LOOP('',(#25705,#25706,#25707,#25708));
#6231=EDGE_LOOP('',(#25709,#25710,#25711));
#6232=EDGE_LOOP('',(#25712,#25713,#25714,#25715));
#6233=EDGE_LOOP('',(#25716,#25717,#25718));
#6234=EDGE_LOOP('',(#25719,#25720,#25721,#25722));
#6235=EDGE_LOOP('',(#25723,#25724,#25725,#25726));
#6236=EDGE_LOOP('',(#25727,#25728,#25729,#25730));
#6237=EDGE_LOOP('',(#25731,#25732,#25733,#25734));
#6238=EDGE_LOOP('',(#25735,#25736,#25737,#25738));
#6239=EDGE_LOOP('',(#25739,#25740,#25741,#25742));
#6240=EDGE_LOOP('',(#25743,#25744,#25745,#25746));
#6241=EDGE_LOOP('',(#25747,#25748,#25749,#25750,#25751,#25752));
#6242=EDGE_LOOP('',(#25753,#25754,#25755,#25756));
#6243=EDGE_LOOP('',(#25757,#25758,#25759,#25760));
#6244=EDGE_LOOP('',(#25761,#25762,#25763,#25764));
#6245=EDGE_LOOP('',(#25765,#25766,#25767,#25768));
#6246=EDGE_LOOP('',(#25769,#25770,#25771,#25772));
#6247=EDGE_LOOP('',(#25773,#25774,#25775,#25776));
#6248=EDGE_LOOP('',(#25777,#25778,#25779,#25780));
#6249=EDGE_LOOP('',(#25781,#25782,#25783,#25784));
#6250=EDGE_LOOP('',(#25785,#25786,#25787,#25788));
#6251=EDGE_LOOP('',(#25789,#25790,#25791));
#6252=EDGE_LOOP('',(#25792,#25793,#25794,#25795));
#6253=EDGE_LOOP('',(#25796,#25797,#25798));
#6254=EDGE_LOOP('',(#25799,#25800,#25801,#25802));
#6255=EDGE_LOOP('',(#25803,#25804,#25805,#25806));
#6256=EDGE_LOOP('',(#25807,#25808,#25809));
#6257=EDGE_LOOP('',(#25810,#25811,#25812,#25813,#25814,#25815,#25816,#25817,
#25818,#25819));
#6258=EDGE_LOOP('',(#25820,#25821,#25822,#25823));
#6259=EDGE_LOOP('',(#25824,#25825,#25826));
#6260=EDGE_LOOP('',(#25827,#25828,#25829,#25830));
#6261=EDGE_LOOP('',(#25831,#25832,#25833));
#6262=EDGE_LOOP('',(#25834,#25835,#25836,#25837));
#6263=EDGE_LOOP('',(#25838,#25839,#25840));
#6264=EDGE_LOOP('',(#25841,#25842,#25843,#25844));
#6265=EDGE_LOOP('',(#25845,#25846,#25847,#25848));
#6266=EDGE_LOOP('',(#25849,#25850,#25851,#25852));
#6267=EDGE_LOOP('',(#25853,#25854,#25855,#25856));
#6268=EDGE_LOOP('',(#25857,#25858,#25859,#25860));
#6269=EDGE_LOOP('',(#25861,#25862,#25863,#25864));
#6270=EDGE_LOOP('',(#25865,#25866,#25867,#25868));
#6271=EDGE_LOOP('',(#25869,#25870,#25871,#25872));
#6272=EDGE_LOOP('',(#25873,#25874,#25875,#25876));
#6273=EDGE_LOOP('',(#25877,#25878,#25879,#25880));
#6274=EDGE_LOOP('',(#25881,#25882,#25883,#25884));
#6275=EDGE_LOOP('',(#25885,#25886,#25887,#25888));
#6276=EDGE_LOOP('',(#25889,#25890,#25891,#25892,#25893,#25894));
#6277=EDGE_LOOP('',(#25895,#25896,#25897,#25898));
#6278=EDGE_LOOP('',(#25899,#25900,#25901,#25902));
#6279=EDGE_LOOP('',(#25903,#25904,#25905));
#6280=EDGE_LOOP('',(#25906,#25907,#25908,#25909));
#6281=EDGE_LOOP('',(#25910,#25911,#25912));
#6282=EDGE_LOOP('',(#25913,#25914,#25915,#25916,#25917,#25918,#25919,#25920,
#25921,#25922));
#6283=EDGE_LOOP('',(#25923,#25924,#25925,#25926));
#6284=EDGE_LOOP('',(#25927,#25928,#25929));
#6285=EDGE_LOOP('',(#25930,#25931,#25932,#25933));
#6286=EDGE_LOOP('',(#25934,#25935,#25936));
#6287=EDGE_LOOP('',(#25937,#25938,#25939,#25940));
#6288=EDGE_LOOP('',(#25941,#25942,#25943));
#6289=EDGE_LOOP('',(#25944,#25945,#25946));
#6290=EDGE_LOOP('',(#25947,#25948,#25949,#25950));
#6291=EDGE_LOOP('',(#25951,#25952,#25953,#25954));
#6292=EDGE_LOOP('',(#25955,#25956,#25957,#25958));
#6293=EDGE_LOOP('',(#25959,#25960,#25961,#25962));
#6294=EDGE_LOOP('',(#25963,#25964,#25965,#25966));
#6295=EDGE_LOOP('',(#25967,#25968,#25969,#25970));
#6296=EDGE_LOOP('',(#25971,#25972,#25973,#25974));
#6297=EDGE_LOOP('',(#25975,#25976,#25977,#25978));
#6298=EDGE_LOOP('',(#25979,#25980,#25981,#25982));
#6299=EDGE_LOOP('',(#25983,#25984,#25985,#25986));
#6300=EDGE_LOOP('',(#25987,#25988,#25989,#25990));
#6301=EDGE_LOOP('',(#25991,#25992,#25993,#25994));
#6302=EDGE_LOOP('',(#25995,#25996,#25997,#25998,#25999,#26000));
#6303=EDGE_LOOP('',(#26001,#26002,#26003,#26004));
#6304=EDGE_LOOP('',(#26005,#26006,#26007,#26008));
#6305=EDGE_LOOP('',(#26009,#26010,#26011,#26012));
#6306=EDGE_LOOP('',(#26013,#26014,#26015,#26016));
#7949=LINE('',#74310,#9789);
#7950=LINE('',#74314,#9790);
#7951=LINE('',#74316,#9791);
#7952=LINE('',#74320,#9792);
#7953=LINE('',#74321,#9793);
#7954=LINE('',#74344,#9794);
#7955=LINE('',#74347,#9795);
#7956=LINE('',#74349,#9796);
#7957=LINE('',#74350,#9797);
#7958=LINE('',#74353,#9798);
#7959=LINE('',#74373,#9799);
#7960=LINE('',#74378,#9800);
#7961=LINE('',#74384,#9801);
#7962=LINE('',#74387,#9802);
#7963=LINE('',#74391,#9803);
#7964=LINE('',#74393,#9804);
#7965=LINE('',#74395,#9805);
#7966=LINE('',#74397,#9806);
#7967=LINE('',#74398,#9807);
#7968=LINE('',#74402,#9808);
#7969=LINE('',#74410,#9809);
#7970=LINE('',#74414,#9810);
#7971=LINE('',#74422,#9811);
#7972=LINE('',#74426,#9812);
#7973=LINE('',#74434,#9813);
#7974=LINE('',#74438,#9814);
#7975=LINE('',#74446,#9815);
#7976=LINE('',#74450,#9816);
#7977=LINE('',#74458,#9817);
#7978=LINE('',#74466,#9818);
#7979=LINE('',#74468,#9819);
#7980=LINE('',#74472,#9820);
#7981=LINE('',#74473,#9821);
#7982=LINE('',#74476,#9822);
#7983=LINE('',#74478,#9823);
#7984=LINE('',#74483,#9824);
#7985=LINE('',#74491,#9825);
#7986=LINE('',#74493,#9826);
#7987=LINE('',#74497,#9827);
#7988=LINE('',#74501,#9828);
#7989=LINE('',#74514,#9829);
#7990=LINE('',#74522,#9830);
#7991=LINE('',#74526,#9831);
#7992=LINE('',#74528,#9832);
#7993=LINE('',#74533,#9833);
#7994=LINE('',#74537,#9834);
#7995=LINE('',#74540,#9835);
#7996=LINE('',#74553,#9836);
#7997=LINE('',#74554,#9837);
#7998=LINE('',#74557,#9838);
#7999=LINE('',#74558,#9839);
#8000=LINE('',#74562,#9840);
#8001=LINE('',#74566,#9841);
#8002=LINE('',#74570,#9842);
#8003=LINE('',#74574,#9843);
#8004=LINE('',#74578,#9844);
#8005=LINE('',#74582,#9845);
#8006=LINE('',#74586,#9846);
#8007=LINE('',#74589,#9847);
#8008=LINE('',#74591,#9848);
#8009=LINE('',#74595,#9849);
#8010=LINE('',#74599,#9850);
#8011=LINE('',#74600,#9851);
#8012=LINE('',#74612,#9852);
#8013=LINE('',#74620,#9853);
#8014=LINE('',#74621,#9854);
#8015=LINE('',#74624,#9855);
#8016=LINE('',#74628,#9856);
#8017=LINE('',#74654,#9857);
#8018=LINE('',#74658,#9858);
#8019=LINE('',#74659,#9859);
#8020=LINE('',#74671,#9860);
#8021=LINE('',#74679,#9861);
#8022=LINE('',#74680,#9862);
#8023=LINE('',#74684,#9863);
#8024=LINE('',#74688,#9864);
#8025=LINE('',#74692,#9865);
#8026=LINE('',#74696,#9866);
#8027=LINE('',#74700,#9867);
#8028=LINE('',#74704,#9868);
#8029=LINE('',#74708,#9869);
#8030=LINE('',#74711,#9870);
#8031=LINE('',#74715,#9871);
#8032=LINE('',#74719,#9872);
#8033=LINE('',#74720,#9873);
#8034=LINE('',#74732,#9874);
#8035=LINE('',#74740,#9875);
#8036=LINE('',#74741,#9876);
#8037=LINE('',#74744,#9877);
#8038=LINE('',#74748,#9878);
#8039=LINE('',#74774,#9879);
#8040=LINE('',#74778,#9880);
#8041=LINE('',#74779,#9881);
#8042=LINE('',#74796,#9882);
#8043=LINE('',#74798,#9883);
#8044=LINE('',#74801,#9884);
#8045=LINE('',#74803,#9885);
#8046=LINE('',#74811,#9886);
#8047=LINE('',#74813,#9887);
#8048=LINE('',#74814,#9888);
#8049=LINE('',#74817,#9889);
#8050=LINE('',#74827,#9890);
#8051=LINE('',#74838,#9891);
#8052=LINE('',#74841,#9892);
#8053=LINE('',#74842,#9893);
#8054=LINE('',#74845,#9894);
#8055=LINE('',#74847,#9895);
#8056=LINE('',#74849,#9896);
#8057=LINE('',#74850,#9897);
#8058=LINE('',#74853,#9898);
#8059=LINE('',#74855,#9899);
#8060=LINE('',#74856,#9900);
#8061=LINE('',#74859,#9901);
#8062=LINE('',#74863,#9902);
#8063=LINE('',#74865,#9903);
#8064=LINE('',#74866,#9904);
#8065=LINE('',#74869,#9905);
#8066=LINE('',#74870,#9906);
#8067=LINE('',#74873,#9907);
#8068=LINE('',#74881,#9908);
#8069=LINE('',#74885,#9909);
#8070=LINE('',#74887,#9910);
#8071=LINE('',#74891,#9911);
#8072=LINE('',#74894,#9912);
#8073=LINE('',#74897,#9913);
#8074=LINE('',#74898,#9914);
#8075=LINE('',#74901,#9915);
#8076=LINE('',#74907,#9916);
#8077=LINE('',#74909,#9917);
#8078=LINE('',#74910,#9918);
#8079=LINE('',#74913,#9919);
#8080=LINE('',#74914,#9920);
#8081=LINE('',#74918,#9921);
#8082=LINE('',#74923,#9922);
#8083=LINE('',#74932,#9923);
#8084=LINE('',#74936,#9924);
#8085=LINE('',#74937,#9925);
#8086=LINE('',#74941,#9926);
#8087=LINE('',#74945,#9927);
#8088=LINE('',#74949,#9928);
#8089=LINE('',#74953,#9929);
#8090=LINE('',#74956,#9930);
#8091=LINE('',#74961,#9931);
#8092=LINE('',#74963,#9932);
#8093=LINE('',#74966,#9933);
#8094=LINE('',#74969,#9934);
#8095=LINE('',#74972,#9935);
#8096=LINE('',#74973,#9936);
#8097=LINE('',#74976,#9937);
#8098=LINE('',#74978,#9938);
#8099=LINE('',#74979,#9939);
#8100=LINE('',#74982,#9940);
#8101=LINE('',#74988,#9941);
#8102=LINE('',#74989,#9942);
#8103=LINE('',#74993,#9943);
#8104=LINE('',#75003,#9944);
#8105=LINE('',#75009,#9945);
#8106=LINE('',#75012,#9946);
#8107=LINE('',#75013,#9947);
#8108=LINE('',#75017,#9948);
#8109=LINE('',#75019,#9949);
#8110=LINE('',#75021,#9950);
#8111=LINE('',#75022,#9951);
#8112=LINE('',#75024,#9952);
#8113=LINE('',#75026,#9953);
#8114=LINE('',#75027,#9954);
#8115=LINE('',#75031,#9955);
#8116=LINE('',#75035,#9956);
#8117=LINE('',#75037,#9957);
#8118=LINE('',#75038,#9958);
#8119=LINE('',#75040,#9959);
#8120=LINE('',#75042,#9960);
#8121=LINE('',#75043,#9961);
#8122=LINE('',#75046,#9962);
#8123=LINE('',#75047,#9963);
#8124=LINE('',#75048,#9964);
#8125=LINE('',#75051,#9965);
#8126=LINE('',#75054,#9966);
#8127=LINE('',#75055,#9967);
#8128=LINE('',#75057,#9968);
#8129=LINE('',#75060,#9969);
#8130=LINE('',#75061,#9970);
#8131=LINE('',#75064,#9971);
#8132=LINE('',#75066,#9972);
#8133=LINE('',#75068,#9973);
#8134=LINE('',#75070,#9974);
#8135=LINE('',#75072,#9975);
#8136=LINE('',#75074,#9976);
#8137=LINE('',#75075,#9977);
#8138=LINE('',#75079,#9978);
#8139=LINE('',#75082,#9979);
#8140=LINE('',#75084,#9980);
#8141=LINE('',#75086,#9981);
#8142=LINE('',#75088,#9982);
#8143=LINE('',#75090,#9983);
#8144=LINE('',#75091,#9984);
#8145=LINE('',#75094,#9985);
#8146=LINE('',#75096,#9986);
#8147=LINE('',#75122,#9987);
#8148=LINE('',#75146,#9988);
#8149=LINE('',#75161,#9989);
#8150=LINE('',#75163,#9990);
#8151=LINE('',#75185,#9991);
#8152=LINE('',#75207,#9992);
#8153=LINE('',#75212,#9993);
#8154=LINE('',#75221,#9994);
#8155=LINE('',#75230,#9995);
#8156=LINE('',#75258,#9996);
#8157=LINE('',#75266,#9997);
#8158=LINE('',#75269,#9998);
#8159=LINE('',#75273,#9999);
#8160=LINE('',#75277,#10000);
#8161=LINE('',#75282,#10001);
#8162=LINE('',#75286,#10002);
#8163=LINE('',#75293,#10003);
#8164=LINE('',#75296,#10004);
#8165=LINE('',#75300,#10005);
#8166=LINE('',#75304,#10006);
#8167=LINE('',#75305,#10007);
#8168=LINE('',#75312,#10008);
#8169=LINE('',#75326,#10009);
#8170=LINE('',#75335,#10010);
#8171=LINE('',#75366,#10011);
#8172=LINE('',#75371,#10012);
#8173=LINE('',#75374,#10013);
#8174=LINE('',#75378,#10014);
#8175=LINE('',#75382,#10015);
#8176=LINE('',#75387,#10016);
#8177=LINE('',#75391,#10017);
#8178=LINE('',#75394,#10018);
#8179=LINE('',#75396,#10019);
#8180=LINE('',#75441,#10020);
#8181=LINE('',#75445,#10021);
#8182=LINE('',#75448,#10022);
#8183=LINE('',#75451,#10023);
#8184=LINE('',#75453,#10024);
#8185=LINE('',#75458,#10025);
#8186=LINE('',#75462,#10026);
#8187=LINE('',#75469,#10027);
#8188=LINE('',#75472,#10028);
#8189=LINE('',#75476,#10029);
#8190=LINE('',#75482,#10030);
#8191=LINE('',#75487,#10031);
#8192=LINE('',#75489,#10032);
#8193=LINE('',#75492,#10033);
#8194=LINE('',#75505,#10034);
#8195=LINE('',#75509,#10035);
#8196=LINE('',#75514,#10036);
#8197=LINE('',#75547,#10037);
#8198=LINE('',#75551,#10038);
#8199=LINE('',#75554,#10039);
#8200=LINE('',#75556,#10040);
#8201=LINE('',#75600,#10041);
#8202=LINE('',#75602,#10042);
#8203=LINE('',#75606,#10043);
#8204=LINE('',#75610,#10044);
#8205=LINE('',#75617,#10045);
#8206=LINE('',#75620,#10046);
#8207=LINE('',#75624,#10047);
#8208=LINE('',#75628,#10048);
#8209=LINE('',#75631,#10049);
#8210=LINE('',#75636,#10050);
#8211=LINE('',#75639,#10051);
#8212=LINE('',#75640,#10052);
#8213=LINE('',#75644,#10053);
#8214=LINE('',#75648,#10054);
#8215=LINE('',#75650,#10055);
#8216=LINE('',#75653,#10056);
#8217=LINE('',#75658,#10057);
#8218=LINE('',#75666,#10058);
#8219=LINE('',#75667,#10059);
#8220=LINE('',#75671,#10060);
#8221=LINE('',#75697,#10061);
#8222=LINE('',#75747,#10062);
#8223=LINE('',#75785,#10063);
#8224=LINE('',#75805,#10064);
#8225=LINE('',#75835,#10065);
#8226=LINE('',#75865,#10066);
#8227=LINE('',#75866,#10067);
#8228=LINE('',#75870,#10068);
#8229=LINE('',#75875,#10069);
#8230=LINE('',#75876,#10070);
#8231=LINE('',#75896,#10071);
#8232=LINE('',#75925,#10072);
#8233=LINE('',#75927,#10073);
#8234=LINE('',#75981,#10074);
#8235=LINE('',#75995,#10075);
#8236=LINE('',#76021,#10076);
#8237=LINE('',#76071,#10077);
#8238=LINE('',#76075,#10078);
#8239=LINE('',#76079,#10079);
#8240=LINE('',#76083,#10080);
#8241=LINE('',#76088,#10081);
#8242=LINE('',#76093,#10082);
#8243=LINE('',#76102,#10083);
#8244=LINE('',#76107,#10084);
#8245=LINE('',#76113,#10085);
#8246=LINE('',#76122,#10086);
#8247=LINE('',#76123,#10087);
#8248=LINE('',#76129,#10088);
#8249=LINE('',#76135,#10089);
#8250=LINE('',#76138,#10090);
#8251=LINE('',#76140,#10091);
#8252=LINE('',#76141,#10092);
#8253=LINE('',#76144,#10093);
#8254=LINE('',#76162,#10094);
#8255=LINE('',#76180,#10095);
#8256=LINE('',#76183,#10096);
#8257=LINE('',#76187,#10097);
#8258=LINE('',#76237,#10098);
#8259=LINE('',#76273,#10099);
#8260=LINE('',#76366,#10100);
#8261=LINE('',#76372,#10101);
#8262=LINE('',#76411,#10102);
#8263=LINE('',#76486,#10103);
#8264=LINE('',#76519,#10104);
#8265=LINE('',#76553,#10105);
#8266=LINE('',#76609,#10106);
#8267=LINE('',#76616,#10107);
#8268=LINE('',#76679,#10108);
#8269=LINE('',#76681,#10109);
#8270=LINE('',#76785,#10110);
#8271=LINE('',#76811,#10111);
#8272=LINE('',#76920,#10112);
#8273=LINE('',#77018,#10113);
#8274=LINE('',#77074,#10114);
#8275=LINE('',#77132,#10115);
#8276=LINE('',#77217,#10116);
#8277=LINE('',#77279,#10117);
#8278=LINE('',#77293,#10118);
#8279=LINE('',#77297,#10119);
#8280=LINE('',#77317,#10120);
#8281=LINE('',#77340,#10121);
#8282=LINE('',#77378,#10122);
#8283=LINE('',#77413,#10123);
#8284=LINE('',#77460,#10124);
#8285=LINE('',#77464,#10125);
#8286=LINE('',#77467,#10126);
#8287=LINE('',#77468,#10127);
#8288=LINE('',#77518,#10128);
#8289=LINE('',#77519,#10129);
#8290=LINE('',#77549,#10130);
#8291=LINE('',#77550,#10131);
#8292=LINE('',#77554,#10132);
#8293=LINE('',#77557,#10133);
#8294=LINE('',#77558,#10134);
#8295=LINE('',#77564,#10135);
#8296=LINE('',#77602,#10136);
#8297=LINE('',#77622,#10137);
#8298=LINE('',#77669,#10138);
#8299=LINE('',#77719,#10139);
#8300=LINE('',#77736,#10140);
#8301=LINE('',#77756,#10141);
#8302=LINE('',#77760,#10142);
#8303=LINE('',#77763,#10143);
#8304=LINE('',#77767,#10144);
#8305=LINE('',#77768,#10145);
#8306=LINE('',#77771,#10146);
#8307=LINE('',#77776,#10147);
#8308=LINE('',#77823,#10148);
#8309=LINE('',#77869,#10149);
#8310=LINE('',#77870,#10150);
#8311=LINE('',#77905,#10151);
#8312=LINE('',#77907,#10152);
#8313=LINE('',#77932,#10153);
#8314=LINE('',#77961,#10154);
#8315=LINE('',#77963,#10155);
#8316=LINE('',#77969,#10156);
#8317=LINE('',#77970,#10157);
#8318=LINE('',#77974,#10158);
#8319=LINE('',#77977,#10159);
#8320=LINE('',#77978,#10160);
#8321=LINE('',#77982,#10161);
#8322=LINE('',#77986,#10162);
#8323=LINE('',#78006,#10163);
#8324=LINE('',#78053,#10164);
#8325=LINE('',#78082,#10165);
#8326=LINE('',#78131,#10166);
#8327=LINE('',#78133,#10167);
#8328=LINE('',#78135,#10168);
#8329=LINE('',#78137,#10169);
#8330=LINE('',#78140,#10170);
#8331=LINE('',#78142,#10171);
#8332=LINE('',#78144,#10172);
#8333=LINE('',#78145,#10173);
#8334=LINE('',#78148,#10174);
#8335=LINE('',#78150,#10175);
#8336=LINE('',#78152,#10176);
#8337=LINE('',#78154,#10177);
#8338=LINE('',#78155,#10178);
#8339=LINE('',#78158,#10179);
#8340=LINE('',#78160,#10180);
#8341=LINE('',#78162,#10181);
#8342=LINE('',#78164,#10182);
#8343=LINE('',#78165,#10183);
#8344=LINE('',#78168,#10184);
#8345=LINE('',#78170,#10185);
#8346=LINE('',#78172,#10186);
#8347=LINE('',#78173,#10187);
#8348=LINE('',#78176,#10188);
#8349=LINE('',#78178,#10189);
#8350=LINE('',#78180,#10190);
#8351=LINE('',#78181,#10191);
#8352=LINE('',#78184,#10192);
#8353=LINE('',#78186,#10193);
#8354=LINE('',#78188,#10194);
#8355=LINE('',#78190,#10195);
#8356=LINE('',#78191,#10196);
#8357=LINE('',#78194,#10197);
#8358=LINE('',#78196,#10198);
#8359=LINE('',#78198,#10199);
#8360=LINE('',#78200,#10200);
#8361=LINE('',#78201,#10201);
#8362=LINE('',#78204,#10202);
#8363=LINE('',#78206,#10203);
#8364=LINE('',#78208,#10204);
#8365=LINE('',#78209,#10205);
#8366=LINE('',#78214,#10206);
#8367=LINE('',#78220,#10207);
#8368=LINE('',#78227,#10208);
#8369=LINE('',#78232,#10209);
#8370=LINE('',#78235,#10210);
#8371=LINE('',#78239,#10211);
#8372=LINE('',#78243,#10212);
#8373=LINE('',#78250,#10213);
#8374=LINE('',#78256,#10214);
#8375=LINE('',#78264,#10215);
#8376=LINE('',#78277,#10216);
#8377=LINE('',#78279,#10217);
#8378=LINE('',#78281,#10218);
#8379=LINE('',#78289,#10219);
#8380=LINE('',#78290,#10220);
#8381=LINE('',#78294,#10221);
#8382=LINE('',#78306,#10222);
#8383=LINE('',#78323,#10223);
#8384=LINE('',#78326,#10224);
#8385=LINE('',#78328,#10225);
#8386=LINE('',#78334,#10226);
#8387=LINE('',#78336,#10227);
#8388=LINE('',#78337,#10228);
#8389=LINE('',#78343,#10229);
#8390=LINE('',#78350,#10230);
#8391=LINE('',#78360,#10231);
#8392=LINE('',#78366,#10232);
#8393=LINE('',#78368,#10233);
#8394=LINE('',#78370,#10234);
#8395=LINE('',#78378,#10235);
#8396=LINE('',#78379,#10236);
#8397=LINE('',#78383,#10237);
#8398=LINE('',#78390,#10238);
#8399=LINE('',#78398,#10239);
#8400=LINE('',#78406,#10240);
#8401=LINE('',#78418,#10241);
#8402=LINE('',#78420,#10242);
#8403=LINE('',#78422,#10243);
#8404=LINE('',#78424,#10244);
#8405=LINE('',#78426,#10245);
#8406=LINE('',#78428,#10246);
#8407=LINE('',#78430,#10247);
#8408=LINE('',#78432,#10248);
#8409=LINE('',#78435,#10249);
#8410=LINE('',#78441,#10250);
#8411=LINE('',#78449,#10251);
#8412=LINE('',#78463,#10252);
#8413=LINE('',#78465,#10253);
#8414=LINE('',#78473,#10254);
#8415=LINE('',#78475,#10255);
#8416=LINE('',#78476,#10256);
#8417=LINE('',#78480,#10257);
#8418=LINE('',#78493,#10258);
#8419=LINE('',#78509,#10259);
#8420=LINE('',#78512,#10260);
#8421=LINE('',#78514,#10261);
#8422=LINE('',#78520,#10262);
#8423=LINE('',#78522,#10263);
#8424=LINE('',#78523,#10264);
#8425=LINE('',#78528,#10265);
#8426=LINE('',#78532,#10266);
#8427=LINE('',#78542,#10267);
#8428=LINE('',#78544,#10268);
#8429=LINE('',#78552,#10269);
#8430=LINE('',#78554,#10270);
#8431=LINE('',#78556,#10271);
#8432=LINE('',#78561,#10272);
#8433=LINE('',#78577,#10273);
#8434=LINE('',#78587,#10274);
#8435=LINE('',#78591,#10275);
#8436=LINE('',#78602,#10276);
#8437=LINE('',#78604,#10277);
#8438=LINE('',#78606,#10278);
#8439=LINE('',#78608,#10279);
#8440=LINE('',#78610,#10280);
#8441=LINE('',#78611,#10281);
#8442=LINE('',#78613,#10282);
#8443=LINE('',#78615,#10283);
#8444=LINE('',#78618,#10284);
#8445=LINE('',#78621,#10285);
#9789=VECTOR('',#40276,1000.);
#9790=VECTOR('',#40281,1000.);
#9791=VECTOR('',#40282,1000.);
#9792=VECTOR('',#40287,1000.);
#9793=VECTOR('',#40288,1000.);
#9794=VECTOR('',#40295,1000.);
#9795=VECTOR('',#40298,1000.);
#9796=VECTOR('',#40299,1000.);
#9797=VECTOR('',#40300,1000.);
#9798=VECTOR('',#40303,1000.);
#9799=VECTOR('',#40312,1000.);
#9800=VECTOR('',#40317,1000.);
#9801=VECTOR('',#40322,1000.);
#9802=VECTOR('',#40325,1000.);
#9803=VECTOR('',#40328,1000.);
#9804=VECTOR('',#40329,1000.);
#9805=VECTOR('',#40330,1000.);
#9806=VECTOR('',#40331,1000.);
#9807=VECTOR('',#40332,1000.);
#9808=VECTOR('',#40335,1000.);
#9809=VECTOR('',#40336,1000.);
#9810=VECTOR('',#40339,1000.);
#9811=VECTOR('',#40340,1000.);
#9812=VECTOR('',#40343,1000.);
#9813=VECTOR('',#40344,1000.);
#9814=VECTOR('',#40347,1000.);
#9815=VECTOR('',#40348,1000.);
#9816=VECTOR('',#40351,1000.);
#9817=VECTOR('',#40358,1000.);
#9818=VECTOR('',#40365,1000.);
#9819=VECTOR('',#40366,1000.);
#9820=VECTOR('',#40369,1000.);
#9821=VECTOR('',#40370,1000.);
#9822=VECTOR('',#40371,1000.);
#9823=VECTOR('',#40372,1000.);
#9824=VECTOR('',#40377,1000.);
#9825=VECTOR('',#40384,1000.);
#9826=VECTOR('',#40385,1000.);
#9827=VECTOR('',#40388,1000.);
#9828=VECTOR('',#40391,1000.);
#9829=VECTOR('',#40404,1000.);
#9830=VECTOR('',#40411,1000.);
#9831=VECTOR('',#40414,1000.);
#9832=VECTOR('',#40415,1000.);
#9833=VECTOR('',#40422,1000.);
#9834=VECTOR('',#40427,1000.);
#9835=VECTOR('',#40430,1000.);
#9836=VECTOR('',#40435,1000.);
#9837=VECTOR('',#40436,1000.);
#9838=VECTOR('',#40439,1000.);
#9839=VECTOR('',#40440,1000.);
#9840=VECTOR('',#40443,1000.);
#9841=VECTOR('',#40446,1000.);
#9842=VECTOR('',#40449,1000.);
#9843=VECTOR('',#40452,1000.);
#9844=VECTOR('',#40455,1000.);
#9845=VECTOR('',#40458,1000.);
#9846=VECTOR('',#40461,1000.);
#9847=VECTOR('',#40464,1000.);
#9848=VECTOR('',#40465,1000.);
#9849=VECTOR('',#40468,1000.);
#9850=VECTOR('',#40473,1000.);
#9851=VECTOR('',#40474,1000.);
#9852=VECTOR('',#40475,1000.);
#9853=VECTOR('',#40478,1000.);
#9854=VECTOR('',#40479,1000.);
#9855=VECTOR('',#40482,1000.);
#9856=VECTOR('',#40485,1000.);
#9857=VECTOR('',#40488,1000.);
#9858=VECTOR('',#40493,1000.);
#9859=VECTOR('',#40494,1000.);
#9860=VECTOR('',#40495,1000.);
#9861=VECTOR('',#40498,1000.);
#9862=VECTOR('',#40499,1000.);
#9863=VECTOR('',#40502,1000.);
#9864=VECTOR('',#40505,1000.);
#9865=VECTOR('',#40508,1000.);
#9866=VECTOR('',#40511,1000.);
#9867=VECTOR('',#40514,1000.);
#9868=VECTOR('',#40517,1000.);
#9869=VECTOR('',#40520,1000.);
#9870=VECTOR('',#40523,1000.);
#9871=VECTOR('',#40526,1000.);
#9872=VECTOR('',#40531,1000.);
#9873=VECTOR('',#40532,1000.);
#9874=VECTOR('',#40533,1000.);
#9875=VECTOR('',#40536,1000.);
#9876=VECTOR('',#40537,1000.);
#9877=VECTOR('',#40540,1000.);
#9878=VECTOR('',#40543,1000.);
#9879=VECTOR('',#40546,1000.);
#9880=VECTOR('',#40551,1000.);
#9881=VECTOR('',#40552,1000.);
#9882=VECTOR('',#40553,1000.);
#9883=VECTOR('',#40556,1000.);
#9884=VECTOR('',#40559,1000.);
#9885=VECTOR('',#40560,1000.);
#9886=VECTOR('',#40569,1000.);
#9887=VECTOR('',#40570,1000.);
#9888=VECTOR('',#40571,1000.);
#9889=VECTOR('',#40574,1000.);
#9890=VECTOR('',#40585,1000.);
#9891=VECTOR('',#40598,1000.);
#9892=VECTOR('',#40601,1000.);
#9893=VECTOR('',#40602,1000.);
#9894=VECTOR('',#40605,1000.);
#9895=VECTOR('',#40606,1000.);
#9896=VECTOR('',#40607,1000.);
#9897=VECTOR('',#40608,1000.);
#9898=VECTOR('',#40611,1000.);
#9899=VECTOR('',#40612,1000.);
#9900=VECTOR('',#40613,1000.);
#9901=VECTOR('',#40616,1000.);
#9902=VECTOR('',#40621,1000.);
#9903=VECTOR('',#40622,1000.);
#9904=VECTOR('',#40623,1000.);
#9905=VECTOR('',#40626,1000.);
#9906=VECTOR('',#40627,1000.);
#9907=VECTOR('',#40630,1000.);
#9908=VECTOR('',#40641,1000.);
#9909=VECTOR('',#40648,1000.);
#9910=VECTOR('',#40651,1000.);
#9911=VECTOR('',#40656,1000.);
#9912=VECTOR('',#40659,1000.);
#9913=VECTOR('',#40662,1000.);
#9914=VECTOR('',#40663,1000.);
#9915=VECTOR('',#40666,1000.);
#9916=VECTOR('',#40673,1000.);
#9917=VECTOR('',#40674,1000.);
#9918=VECTOR('',#40675,1000.);
#9919=VECTOR('',#40678,1000.);
#9920=VECTOR('',#40679,1000.);
#9921=VECTOR('',#40684,1000.);
#9922=VECTOR('',#40689,2.25);
#9923=VECTOR('',#40700,1000.);
#9924=VECTOR('',#40705,1000.);
#9925=VECTOR('',#40706,1000.);
#9926=VECTOR('',#40711,1000.);
#9927=VECTOR('',#40716,1000.);
#9928=VECTOR('',#40721,1000.);
#9929=VECTOR('',#40726,1000.);
#9930=VECTOR('',#40729,1000.);
#9931=VECTOR('',#40736,1000.);
#9932=VECTOR('',#40739,1000.);
#9933=VECTOR('',#40742,1000.);
#9934=VECTOR('',#40745,1000.);
#9935=VECTOR('',#40748,1000.);
#9936=VECTOR('',#40749,1000.);
#9937=VECTOR('',#40752,1000.);
#9938=VECTOR('',#40753,1000.);
#9939=VECTOR('',#40754,1000.);
#9940=VECTOR('',#40757,1000.);
#9941=VECTOR('',#40764,1000.);
#9942=VECTOR('',#40765,1000.);
#9943=VECTOR('',#40770,1000.);
#9944=VECTOR('',#40781,2.25);
#9945=VECTOR('',#40790,1000.);
#9946=VECTOR('',#40793,1000.);
#9947=VECTOR('',#40794,1000.);
#9948=VECTOR('',#40797,1000.);
#9949=VECTOR('',#40798,1000.);
#9950=VECTOR('',#40799,1000.);
#9951=VECTOR('',#40800,1000.);
#9952=VECTOR('',#40801,1000.);
#9953=VECTOR('',#40802,1000.);
#9954=VECTOR('',#40803,1000.);
#9955=VECTOR('',#40808,1000.);
#9956=VECTOR('',#40811,1000.);
#9957=VECTOR('',#40812,1000.);
#9958=VECTOR('',#40813,1000.);
#9959=VECTOR('',#40814,1000.);
#9960=VECTOR('',#40815,1000.);
#9961=VECTOR('',#40816,1000.);
#9962=VECTOR('',#40819,1000.);
#9963=VECTOR('',#40820,1000.);
#9964=VECTOR('',#40821,1000.);
#9965=VECTOR('',#40826,1000.);
#9966=VECTOR('',#40829,1000.);
#9967=VECTOR('',#40830,1000.);
#9968=VECTOR('',#40833,1000.);
#9969=VECTOR('',#40836,1000.);
#9970=VECTOR('',#40837,1000.);
#9971=VECTOR('',#40840,1000.);
#9972=VECTOR('',#40841,1000.);
#9973=VECTOR('',#40842,1000.);
#9974=VECTOR('',#40843,1000.);
#9975=VECTOR('',#40844,1000.);
#9976=VECTOR('',#40845,1000.);
#9977=VECTOR('',#40846,1000.);
#9978=VECTOR('',#40851,1000.);
#9979=VECTOR('',#40854,1000.);
#9980=VECTOR('',#40855,1000.);
#9981=VECTOR('',#40856,1000.);
#9982=VECTOR('',#40857,1000.);
#9983=VECTOR('',#40858,1000.);
#9984=VECTOR('',#40859,1000.);
#9985=VECTOR('',#40862,1000.);
#9986=VECTOR('',#40863,1000.);
#9987=VECTOR('',#40872,1000.);
#9988=VECTOR('',#40877,1000.);
#9989=VECTOR('',#40882,1000.);
#9990=VECTOR('',#40883,1000.);
#9991=VECTOR('',#40900,1000.);
#9992=VECTOR('',#40927,1000.);
#9993=VECTOR('',#40932,1000.);
#9994=VECTOR('',#40943,1000.);
#9995=VECTOR('',#40956,1000.);
#9996=VECTOR('',#40965,1000.);
#9997=VECTOR('',#40974,1000.);
#9998=VECTOR('',#40977,1000.);
#9999=VECTOR('',#40980,1000.);
#10000=VECTOR('',#40983,1000.);
#10001=VECTOR('',#40988,1000.);
#10002=VECTOR('',#40991,1000.);
#10003=VECTOR('',#40998,1000.);
#10004=VECTOR('',#41001,1000.);
#10005=VECTOR('',#41004,1000.);
#10006=VECTOR('',#41011,1000.);
#10007=VECTOR('',#41012,1000.);
#10008=VECTOR('',#41021,10.);
#10009=VECTOR('',#41024,1000.);
#10010=VECTOR('',#41033,10.);
#10011=VECTOR('',#41034,10.);
#10012=VECTOR('',#41039,10.);
#10013=VECTOR('',#41042,10.);
#10014=VECTOR('',#41045,10.);
#10015=VECTOR('',#41048,10.);
#10016=VECTOR('',#41053,10.);
#10017=VECTOR('',#41056,10.);
#10018=VECTOR('',#41059,10.);
#10019=VECTOR('',#41060,1000.);
#10020=VECTOR('',#41067,1000.);
#10021=VECTOR('',#41072,1000.);
#10022=VECTOR('',#41075,1000.);
#10023=VECTOR('',#41078,1000.);
#10024=VECTOR('',#41079,1000.);
#10025=VECTOR('',#41084,1000.);
#10026=VECTOR('',#41087,1000.);
#10027=VECTOR('',#41094,1000.);
#10028=VECTOR('',#41097,1000.);
#10029=VECTOR('',#41100,1000.);
#10030=VECTOR('',#41111,1000.);
#10031=VECTOR('',#41120,1000.);
#10032=VECTOR('',#41123,1000.);
#10033=VECTOR('',#41126,1000.);
#10034=VECTOR('',#41129,10.);
#10035=VECTOR('',#41132,10.);
#10036=VECTOR('',#41137,10.);
#10037=VECTOR('',#41142,10.);
#10038=VECTOR('',#41145,10.);
#10039=VECTOR('',#41148,10.);
#10040=VECTOR('',#41149,10.);
#10041=VECTOR('',#41154,1000.);
#10042=VECTOR('',#41155,10.);
#10043=VECTOR('',#41158,10.);
#10044=VECTOR('',#41161,10.);
#10045=VECTOR('',#41170,1000.);
#10046=VECTOR('',#41173,1000.);
#10047=VECTOR('',#41178,1000.);
#10048=VECTOR('',#41183,1000.);
#10049=VECTOR('',#41186,1000.);
#10050=VECTOR('',#41193,1000.);
#10051=VECTOR('',#41196,1000.);
#10052=VECTOR('',#41197,1000.);
#10053=VECTOR('',#41202,1000.);
#10054=VECTOR('',#41207,1000.);
#10055=VECTOR('',#41210,1000.);
#10056=VECTOR('',#41213,5.5);
#10057=VECTOR('',#41220,5.5);
#10058=VECTOR('',#41229,1000.);
#10059=VECTOR('',#41230,1000.);
#10060=VECTOR('',#41235,1000.);
#10061=VECTOR('',#41236,1000.);
#10062=VECTOR('',#41237,1000.);
#10063=VECTOR('',#41238,1000.);
#10064=VECTOR('',#41239,1000.);
#10065=VECTOR('',#41240,1000.);
#10066=VECTOR('',#41241,1000.);
#10067=VECTOR('',#41242,1000.);
#10068=VECTOR('',#41247,1000.);
#10069=VECTOR('',#41252,1000.);
#10070=VECTOR('',#41253,1000.);
#10071=VECTOR('',#41254,1000.);
#10072=VECTOR('',#41255,1000.);
#10073=VECTOR('',#41256,1000.);
#10074=VECTOR('',#41257,1000.);
#10075=VECTOR('',#41258,1000.);
#10076=VECTOR('',#41259,1000.);
#10077=VECTOR('',#41260,1000.);
#10078=VECTOR('',#41265,1000.);
#10079=VECTOR('',#41270,1000.);
#10080=VECTOR('',#41275,1.25);
#10081=VECTOR('',#41280,1000.);
#10082=VECTOR('',#41285,1000.);
#10083=VECTOR('',#41296,1.25);
#10084=VECTOR('',#41303,1000.);
#10085=VECTOR('',#41310,1000.);
#10086=VECTOR('',#41311,1000.);
#10087=VECTOR('',#41312,1000.);
#10088=VECTOR('',#41319,10.);
#10089=VECTOR('',#41326,1000.);
#10090=VECTOR('',#41329,1000.);
#10091=VECTOR('',#41330,10.);
#10092=VECTOR('',#41331,1000.);
#10093=VECTOR('',#41334,4.7);
#10094=VECTOR('',#41353,4.7);
#10095=VECTOR('',#41372,1000.);
#10096=VECTOR('',#41375,1000.);
#10097=VECTOR('',#41378,1000.);
#10098=VECTOR('',#41383,1000.);
#10099=VECTOR('',#41384,1000.);
#10100=VECTOR('',#41385,1000.);
#10101=VECTOR('',#41392,1000.);
#10102=VECTOR('',#41393,1000.);
#10103=VECTOR('',#41394,1000.);
#10104=VECTOR('',#41395,1000.);
#10105=VECTOR('',#41398,1000.);
#10106=VECTOR('',#41423,1000.);
#10107=VECTOR('',#41424,1000.);
#10108=VECTOR('',#41431,1000.);
#10109=VECTOR('',#41432,1000.);
#10110=VECTOR('',#41453,1000.);
#10111=VECTOR('',#41466,1000.);
#10112=VECTOR('',#41489,1000.);
#10113=VECTOR('',#41504,1000.);
#10114=VECTOR('',#41513,1000.);
#10115=VECTOR('',#41518,1000.);
#10116=VECTOR('',#41531,1000.);
#10117=VECTOR('',#41532,1000.);
#10118=VECTOR('',#41533,1000.);
#10119=VECTOR('',#41538,1000.);
#10120=VECTOR('',#41539,1000.);
#10121=VECTOR('',#41540,1000.);
#10122=VECTOR('',#41541,1000.);
#10123=VECTOR('',#41542,1000.);
#10124=VECTOR('',#41543,1000.);
#10125=VECTOR('',#41548,1000.);
#10126=VECTOR('',#41551,1000.);
#10127=VECTOR('',#41552,1000.);
#10128=VECTOR('',#41557,1000.);
#10129=VECTOR('',#41558,1000.);
#10130=VECTOR('',#41559,1000.);
#10131=VECTOR('',#41560,1000.);
#10132=VECTOR('',#41565,1000.);
#10133=VECTOR('',#41568,1000.);
#10134=VECTOR('',#41569,1000.);
#10135=VECTOR('',#41578,1000.);
#10136=VECTOR('',#41579,1000.);
#10137=VECTOR('',#41580,1000.);
#10138=VECTOR('',#41581,1000.);
#10139=VECTOR('',#41582,1000.);
#10140=VECTOR('',#41583,1000.);
#10141=VECTOR('',#41584,1000.);
#10142=VECTOR('',#41589,1000.);
#10143=VECTOR('',#41592,1000.);
#10144=VECTOR('',#41597,1000.);
#10145=VECTOR('',#41598,1000.);
#10146=VECTOR('',#41601,1000.);
#10147=VECTOR('',#41608,1000.);
#10148=VECTOR('',#41609,1000.);
#10149=VECTOR('',#41610,1000.);
#10150=VECTOR('',#41611,1000.);
#10151=VECTOR('',#41612,1000.);
#10152=VECTOR('',#41615,1000.);
#10153=VECTOR('',#41616,1000.);
#10154=VECTOR('',#41617,1000.);
#10155=VECTOR('',#41620,1000.);
#10156=VECTOR('',#41627,1000.);
#10157=VECTOR('',#41628,1000.);
#10158=VECTOR('',#41633,1000.);
#10159=VECTOR('',#41636,1000.);
#10160=VECTOR('',#41637,1000.);
#10161=VECTOR('',#41642,1000.);
#10162=VECTOR('',#41647,1000.);
#10163=VECTOR('',#41648,1000.);
#10164=VECTOR('',#41649,1000.);
#10165=VECTOR('',#41650,1000.);
#10166=VECTOR('',#41657,1000.);
#10167=VECTOR('',#41660,1000.);
#10168=VECTOR('',#41663,1000.);
#10169=VECTOR('',#41666,1000.);
#10170=VECTOR('',#41669,1000.);
#10171=VECTOR('',#41670,1000.);
#10172=VECTOR('',#41671,1000.);
#10173=VECTOR('',#41672,1000.);
#10174=VECTOR('',#41675,1000.);
#10175=VECTOR('',#41676,1000.);
#10176=VECTOR('',#41677,1000.);
#10177=VECTOR('',#41678,1000.);
#10178=VECTOR('',#41679,1000.);
#10179=VECTOR('',#41682,1000.);
#10180=VECTOR('',#41683,1000.);
#10181=VECTOR('',#41684,1000.);
#10182=VECTOR('',#41685,1000.);
#10183=VECTOR('',#41686,1000.);
#10184=VECTOR('',#41689,1000.);
#10185=VECTOR('',#41690,1000.);
#10186=VECTOR('',#41691,1000.);
#10187=VECTOR('',#41692,1000.);
#10188=VECTOR('',#41695,1000.);
#10189=VECTOR('',#41696,1000.);
#10190=VECTOR('',#41697,1000.);
#10191=VECTOR('',#41698,1000.);
#10192=VECTOR('',#41701,1000.);
#10193=VECTOR('',#41702,1000.);
#10194=VECTOR('',#41703,1000.);
#10195=VECTOR('',#41704,1000.);
#10196=VECTOR('',#41705,1000.);
#10197=VECTOR('',#41708,1000.);
#10198=VECTOR('',#41709,1000.);
#10199=VECTOR('',#41710,1000.);
#10200=VECTOR('',#41711,1000.);
#10201=VECTOR('',#41712,1000.);
#10202=VECTOR('',#41715,1000.);
#10203=VECTOR('',#41716,1000.);
#10204=VECTOR('',#41717,1000.);
#10205=VECTOR('',#41718,1000.);
#10206=VECTOR('',#41725,1000.);
#10207=VECTOR('',#41732,1000.);
#10208=VECTOR('',#41741,1000.);
#10209=VECTOR('',#41746,1000.);
#10210=VECTOR('',#41749,1000.);
#10211=VECTOR('',#41754,1000.);
#10212=VECTOR('',#41757,1000.);
#10213=VECTOR('',#41768,1000.);
#10214=VECTOR('',#41775,1000.);
#10215=VECTOR('',#41788,1000.);
#10216=VECTOR('',#41809,1000.);
#10217=VECTOR('',#41810,1000.);
#10218=VECTOR('',#41811,1000.);
#10219=VECTOR('',#41818,1000.);
#10220=VECTOR('',#41819,1000.);
#10221=VECTOR('',#41824,1000.);
#10222=VECTOR('',#41843,1000.);
#10223=VECTOR('',#41876,1000.);
#10224=VECTOR('',#41881,1000.);
#10225=VECTOR('',#41884,1000.);
#10226=VECTOR('',#41893,1000.);
#10227=VECTOR('',#41894,1000.);
#10228=VECTOR('',#41895,1000.);
#10229=VECTOR('',#41902,1000.);
#10230=VECTOR('',#41913,1000.);
#10231=VECTOR('',#41928,1000.);
#10232=VECTOR('',#41937,1000.);
#10233=VECTOR('',#41938,1000.);
#10234=VECTOR('',#41939,1000.);
#10235=VECTOR('',#41946,1000.);
#10236=VECTOR('',#41947,1000.);
#10237=VECTOR('',#41952,1000.);
#10238=VECTOR('',#41961,1000.);
#10239=VECTOR('',#41972,1000.);
#10240=VECTOR('',#41983,1000.);
#10241=VECTOR('',#42004,1000.);
#10242=VECTOR('',#42007,1000.);
#10243=VECTOR('',#42010,1000.);
#10244=VECTOR('',#42013,1000.);
#10245=VECTOR('',#42016,1000.);
#10246=VECTOR('',#42019,1000.);
#10247=VECTOR('',#42022,1000.);
#10248=VECTOR('',#42025,1000.);
#10249=VECTOR('',#42030,1000.);
#10250=VECTOR('',#42037,1000.);
#10251=VECTOR('',#42050,1000.);
#10252=VECTOR('',#42073,1000.);
#10253=VECTOR('',#42074,1000.);
#10254=VECTOR('',#42081,1000.);
#10255=VECTOR('',#42082,1000.);
#10256=VECTOR('',#42083,1000.);
#10257=VECTOR('',#42088,1000.);
#10258=VECTOR('',#42109,1000.);
#10259=VECTOR('',#42140,1000.);
#10260=VECTOR('',#42145,1000.);
#10261=VECTOR('',#42148,1000.);
#10262=VECTOR('',#42157,1000.);
#10263=VECTOR('',#42158,1000.);
#10264=VECTOR('',#42159,1000.);
#10265=VECTOR('',#42164,1000.);
#10266=VECTOR('',#42169,1000.);
#10267=VECTOR('',#42186,1000.);
#10268=VECTOR('',#42187,1000.);
#10269=VECTOR('',#42194,1000.);
#10270=VECTOR('',#42195,1000.);
#10271=VECTOR('',#42196,1000.);
#10272=VECTOR('',#42203,1000.);
#10273=VECTOR('',#42226,1000.);
#10274=VECTOR('',#42241,1000.);
#10275=VECTOR('',#42246,1000.);
#10276=VECTOR('',#42265,1000.);
#10277=VECTOR('',#42268,1000.);
#10278=VECTOR('',#42271,1000.);
#10279=VECTOR('',#42274,1000.);
#10280=VECTOR('',#42277,1000.);
#10281=VECTOR('',#42278,1000.);
#10282=VECTOR('',#42281,1000.);
#10283=VECTOR('',#42284,1000.);
#10284=VECTOR('',#42289,1000.);
#10285=VECTOR('',#42294,1000.);
#11640=CIRCLE('',#34964,6.6905058179921);
#11641=CIRCLE('',#34966,6.69050581799);
#11642=CIRCLE('',#34970,6.69050581798971);
#11643=CIRCLE('',#34973,6.69050581799);
#11644=CIRCLE('',#34976,4.44342636361);
#11645=CIRCLE('',#34977,4.44342636361);
#11646=CIRCLE('',#34978,4.44342636361);
#11647=CIRCLE('',#34980,6.24342636361);
#11648=CIRCLE('',#34981,6.24342636361);
#11649=CIRCLE('',#34984,17.4);
#11650=CIRCLE('',#34985,16.4);
#11651=CIRCLE('',#34986,17.4);
#11652=CIRCLE('',#34987,16.4);
#11653=CIRCLE('',#34988,7.6);
#11654=CIRCLE('',#34989,0.2);
#11655=CIRCLE('',#34990,7.6);
#11656=CIRCLE('',#34991,16.1);
#11657=CIRCLE('',#34992,0.2);
#11658=CIRCLE('',#34993,7.6);
#11659=CIRCLE('',#34994,16.1);
#11660=CIRCLE('',#34995,7.6);
#11661=CIRCLE('',#34996,0.2);
#11662=CIRCLE('',#34997,16.1);
#11663=CIRCLE('',#34998,2.25);
#11664=CIRCLE('',#34999,7.34342636361);
#11665=CIRCLE('',#35000,16.1);
#11666=CIRCLE('',#35001,7.34342636361);
#11667=CIRCLE('',#35002,0.5);
#11668=CIRCLE('',#35003,6.5);
#11669=CIRCLE('',#35004,0.5);
#11670=CIRCLE('',#35005,0.5);
#11671=CIRCLE('',#35006,6.5);
#11672=CIRCLE('',#35007,0.5);
#11673=CIRCLE('',#35008,6.24342636361);
#11674=CIRCLE('',#35009,2.25);
#11675=CIRCLE('',#35010,7.34342636361);
#11676=CIRCLE('',#35011,16.1);
#11677=CIRCLE('',#35012,7.34342636361);
#11678=CIRCLE('',#35014,16.1);
#11679=CIRCLE('',#35019,7.59999999999999);
#11680=CIRCLE('',#35022,16.4);
#11681=CIRCLE('',#35023,16.4);
#11682=CIRCLE('',#35024,16.4);
#11683=CIRCLE('',#35025,16.4);
#11684=CIRCLE('',#35026,16.4);
#11685=CIRCLE('',#35027,16.4);
#11686=CIRCLE('',#35028,16.4);
#11687=CIRCLE('',#35029,16.4);
#11688=CIRCLE('',#35030,16.4);
#11689=CIRCLE('',#35034,17.4);
#11690=CIRCLE('',#35035,17.4);
#11691=CIRCLE('',#35036,17.4);
#11692=CIRCLE('',#35040,16.4);
#11693=CIRCLE('',#35041,16.4);
#11694=CIRCLE('',#35042,16.4);
#11695=CIRCLE('',#35043,16.4);
#11696=CIRCLE('',#35044,16.4);
#11697=CIRCLE('',#35045,16.4);
#11698=CIRCLE('',#35046,16.4);
#11699=CIRCLE('',#35047,16.4);
#11700=CIRCLE('',#35048,16.4);
#11701=CIRCLE('',#35052,17.4);
#11702=CIRCLE('',#35053,17.4);
#11703=CIRCLE('',#35054,17.4);
#11704=CIRCLE('',#35058,16.1);
#11705=CIRCLE('',#35059,16.1);
#11706=CIRCLE('',#35060,16.1);
#11707=CIRCLE('',#35063,7.6);
#11708=CIRCLE('',#35064,7.6);
#11709=CIRCLE('',#35065,7.6);
#11710=CIRCLE('',#35066,7.6);
#11711=CIRCLE('',#35068,0.2);
#11712=CIRCLE('',#35070,7.6);
#11713=CIRCLE('',#35071,7.6);
#11714=CIRCLE('',#35072,7.6);
#11715=CIRCLE('',#35073,7.6);
#11716=CIRCLE('',#35078,16.1);
#11717=CIRCLE('',#35082,7.6);
#11718=CIRCLE('',#35083,7.6);
#11719=CIRCLE('',#35085,0.2);
#11720=CIRCLE('',#35087,0.2);
#11721=CIRCLE('',#35089,7.6);
#11722=CIRCLE('',#35093,7.34342636361);
#11723=CIRCLE('',#35096,16.1);
#11724=CIRCLE('',#35097,16.1);
#11725=CIRCLE('',#35101,7.34342636361);
#11726=CIRCLE('',#35103,2.25);
#11727=CIRCLE('',#35104,2.25);
#11728=CIRCLE('',#35105,2.25);
#11729=CIRCLE('',#35106,2.25);
#11730=CIRCLE('',#35107,2.25);
#11731=CIRCLE('',#35109,6.24342636361);
#11732=CIRCLE('',#35112,0.5);
#11733=CIRCLE('',#35114,6.5);
#11734=CIRCLE('',#35116,0.5);
#11735=CIRCLE('',#35118,0.5);
#11736=CIRCLE('',#35120,6.5);
#11737=CIRCLE('',#35122,0.5);
#11738=CIRCLE('',#35125,7.34342636361);
#11739=CIRCLE('',#35129,16.1);
#11740=CIRCLE('',#35130,16.1);
#11741=CIRCLE('',#35133,7.34342636361);
#11742=CIRCLE('',#35135,2.25);
#11743=CIRCLE('',#35136,2.25);
#11744=CIRCLE('',#35137,2.25);
#11745=CIRCLE('',#35138,2.25);
#11746=CIRCLE('',#35139,2.25);
#11747=CIRCLE('',#35140,2.25);
#11748=CIRCLE('',#35146,16.7);
#11749=CIRCLE('',#35156,16.7);
#11750=CIRCLE('',#35159,16.4000000000001);
#11751=CIRCLE('',#35180,0.5);
#11752=CIRCLE('',#35181,1.75);
#11753=CIRCLE('',#35183,0.5);
#11754=CIRCLE('',#35184,6.5);
#11755=CIRCLE('',#35185,0.5);
#11756=CIRCLE('',#35186,6.5);
#11757=CIRCLE('',#35187,0.5);
#11758=CIRCLE('',#35188,5.24342636361);
#11759=CIRCLE('',#35189,5.24342636361);
#11760=CIRCLE('',#35190,5.5);
#11761=CIRCLE('',#35191,5.5);
#11762=CIRCLE('',#35198,0.5);
#11763=CIRCLE('',#35199,1.75);
#11764=CIRCLE('',#35202,16.4);
#11765=CIRCLE('',#35203,16.4);
#11766=CIRCLE('',#35205,15.4);
#11767=CIRCLE('',#35206,15.4);
#11768=CIRCLE('',#35208,15.4);
#11769=CIRCLE('',#35209,15.4);
#11770=CIRCLE('',#35211,15.4);
#11771=CIRCLE('',#35212,15.4);
#11772=CIRCLE('',#35214,15.4);
#11773=CIRCLE('',#35215,15.4);
#11774=CIRCLE('',#35217,15.4);
#11775=CIRCLE('',#35218,15.4);
#11776=CIRCLE('',#35220,15.4);
#11777=CIRCLE('',#35221,15.4);
#11778=CIRCLE('',#35224,16.7);
#11779=CIRCLE('',#35227,10.8000000000012);
#11780=CIRCLE('',#35228,15.4);
#11781=CIRCLE('',#35230,15.4000000000006);
#11782=CIRCLE('',#35231,0.299999999999997);
#11783=CIRCLE('',#35232,0.300000000000003);
#11784=CIRCLE('',#35234,15.4);
#11785=CIRCLE('',#35235,0.300000000000001);
#11786=CIRCLE('',#35236,0.299999999999996);
#11787=CIRCLE('',#35237,0.3);
#11788=CIRCLE('',#35238,0.300000000000001);
#11789=CIRCLE('',#35239,0.300000000000001);
#11790=CIRCLE('',#35240,0.300000000000001);
#11791=CIRCLE('',#35241,7.04342636361);
#11792=CIRCLE('',#35242,0.0999999999999999);
#11793=CIRCLE('',#35244,15.4);
#11794=CIRCLE('',#35246,15.4);
#11795=CIRCLE('',#35248,15.4);
#11796=CIRCLE('',#35250,15.4);
#11797=CIRCLE('',#35251,15.4);
#11798=CIRCLE('',#35253,15.4);
#11799=CIRCLE('',#35254,15.4);
#11800=CIRCLE('',#35256,15.4);
#11801=CIRCLE('',#35257,15.4);
#11802=CIRCLE('',#35259,16.4);
#11803=CIRCLE('',#35263,16.7);
#11804=CIRCLE('',#35267,10.7999999999998);
#11805=CIRCLE('',#35269,0.299999999999998);
#11806=CIRCLE('',#35270,0.300000000000003);
#11807=CIRCLE('',#35272,0.299999999999997);
#11808=CIRCLE('',#35273,0.300000000000004);
#11809=CIRCLE('',#35274,0.3);
#11810=CIRCLE('',#35275,0.0999999999999991);
#11811=CIRCLE('',#35276,7.04342636361);
#11812=CIRCLE('',#35277,0.299999999999999);
#11813=CIRCLE('',#35278,0.300000000000001);
#11814=CIRCLE('',#35279,0.300000000000003);
#11815=CIRCLE('',#35281,1.25);
#11816=CIRCLE('',#35283,0.5);
#11817=CIRCLE('',#35285,6.5);
#11818=CIRCLE('',#35287,0.5);
#11819=CIRCLE('',#35289,6.5);
#11820=CIRCLE('',#35291,0.5);
#11821=CIRCLE('',#35294,5.24342636361);
#11822=CIRCLE('',#35296,5.24342636361);
#11823=CIRCLE('',#35299,5.5);
#11824=CIRCLE('',#35301,5.5);
#11825=CIRCLE('',#35303,1.25);
#11826=CIRCLE('',#35305,7.04342636361);
#11827=CIRCLE('',#35307,0.1);
#11828=CIRCLE('',#35309,10.8);
#11829=CIRCLE('',#35311,10.8);
#11830=CIRCLE('',#35313,0.1);
#11831=CIRCLE('',#35315,7.04342636361);
#11832=CIRCLE('',#35317,1.25);
#11833=CIRCLE('',#35319,4.44342636361);
#11834=CIRCLE('',#35320,7.3);
#11835=CIRCLE('',#35321,7.3);
#11836=CIRCLE('',#35323,4.7);
#11837=CIRCLE('',#35325,4.7);
#11838=CIRCLE('',#35327,1.25);
#11839=CIRCLE('',#35330,4.44342636361);
#11840=CIRCLE('',#35331,4.44342636361);
#11841=CIRCLE('',#35334,7.3);
#11842=CIRCLE('',#35335,7.3);
#11843=CIRCLE('',#35337,7.3);
#11844=CIRCLE('',#35338,7.3);
#11845=CIRCLE('',#35341,4.7);
#11846=CIRCLE('',#35342,4.7);
#11847=CIRCLE('',#35343,4.7);
#11848=CIRCLE('',#35344,4.7);
#11849=CIRCLE('',#35345,4.7);
#11850=CIRCLE('',#35346,4.7);
#11851=CIRCLE('',#35347,4.7);
#11852=CIRCLE('',#35349,4.7);
#11853=CIRCLE('',#35350,4.7);
#11854=CIRCLE('',#35351,4.7);
#11855=CIRCLE('',#35352,4.7);
#11856=CIRCLE('',#35353,4.7);
#11857=CIRCLE('',#35354,4.7);
#11858=CIRCLE('',#35355,4.7);
#11859=CIRCLE('',#35358,6.24342636361);
#11860=CIRCLE('',#35359,6.24342636361);
#11861=CIRCLE('',#35361,0.3);
#11862=CIRCLE('',#35362,0.3);
#11863=CIRCLE('',#35364,10.);
#11864=CIRCLE('',#35365,10.);
#11865=CIRCLE('',#35367,0.3);
#11866=CIRCLE('',#35368,0.3);
#11867=CIRCLE('',#35370,6.24342636361);
#11868=CIRCLE('',#35371,6.24342636361);
#11869=CIRCLE('',#35376,4.44342636361);
#11870=CIRCLE('',#35377,4.44342636361);
#11871=CIRCLE('',#35380,3.);
#11872=CIRCLE('',#35384,0.300000000000001);
#11873=CIRCLE('',#35391,0.3);
#11874=CIRCLE('',#35392,0.3);
#11875=CIRCLE('',#35397,0.3);
#11876=CIRCLE('',#35398,0.3);
#11877=CIRCLE('',#35400,0.299999999999995);
#11878=CIRCLE('',#35407,5.69050581798992);
#11879=CIRCLE('',#35408,0.500000000000001);
#11880=CIRCLE('',#35409,1.1);
#11881=CIRCLE('',#35410,3.00000194400981);
#11882=CIRCLE('',#35411,3.);
#11883=CIRCLE('',#35412,5.24342636360999);
#11884=CIRCLE('',#35413,5.24342636361);
#11885=CIRCLE('',#35414,3.00000180903519);
#11886=CIRCLE('',#35415,1.1);
#11887=CIRCLE('',#35416,0.5);
#11888=CIRCLE('',#35417,5.69050581798992);
#11889=CIRCLE('',#35419,4.44342636361);
#11890=CIRCLE('',#35421,4.44342636361);
#11891=CIRCLE('',#35423,5.24342636361);
#11892=CIRCLE('',#35424,5.24342636361);
#11893=CIRCLE('',#35425,3.);
#11894=CIRCLE('',#35426,3.);
#11895=CIRCLE('',#35429,0.3);
#11896=CIRCLE('',#35431,0.3);
#11897=CIRCLE('',#35434,0.3);
#11898=CIRCLE('',#35436,0.3);
#11899=CIRCLE('',#35439,0.3);
#11900=CIRCLE('',#35441,0.3);
#11901=CIRCLE('',#35443,5.69050581799);
#11902=CIRCLE('',#35445,0.5);
#11903=CIRCLE('',#35448,1.1);
#11904=CIRCLE('',#35450,3.);
#11905=CIRCLE('',#35455,3.);
#11906=CIRCLE('',#35457,1.1);
#11907=CIRCLE('',#35460,0.5);
#11908=CIRCLE('',#35462,5.69050581799);
#11909=CIRCLE('',#35478,0.3);
#11910=CIRCLE('',#35480,0.3);
#11911=CIRCLE('',#35482,0.3);
#11912=CIRCLE('',#35483,0.3);
#11913=CIRCLE('',#35484,0.3);
#11914=CIRCLE('',#35485,0.3);
#11915=CIRCLE('',#35486,0.3);
#11916=CIRCLE('',#35487,0.3);
#11917=CIRCLE('',#35488,0.3);
#11918=CIRCLE('',#35489,0.3);
#11919=CIRCLE('',#35490,0.3);
#11920=CIRCLE('',#35491,0.3);
#11921=CIRCLE('',#35492,0.3);
#11922=CIRCLE('',#35493,0.3);
#11923=CIRCLE('',#35495,0.3);
#11924=CIRCLE('',#35497,0.3);
#11925=CIRCLE('',#35499,0.3);
#11926=CIRCLE('',#35500,0.300000000000001);
#11927=CIRCLE('',#35502,0.3);
#11928=CIRCLE('',#35504,0.299999999999999);
#11929=CIRCLE('',#35506,0.3);
#11930=CIRCLE('',#35508,0.3);
#11931=CIRCLE('',#35510,0.300000000000001);
#11932=CIRCLE('',#35511,16.1);
#11933=CIRCLE('',#35513,0.3);
#11934=CIRCLE('',#35515,0.300000000000001);
#11935=CIRCLE('',#35517,0.6);
#11936=CIRCLE('',#35518,15.7);
#11937=CIRCLE('',#35519,0.6);
#11938=CIRCLE('',#35521,0.300000000000001);
#11939=CIRCLE('',#35523,0.3);
#11940=CIRCLE('',#35524,0.3);
#11941=CIRCLE('',#35526,0.3);
#11942=CIRCLE('',#35528,0.3);
#11943=CIRCLE('',#35529,0.3);
#11944=CIRCLE('',#35531,0.300000000000001);
#11945=CIRCLE('',#35533,0.3);
#11946=CIRCLE('',#35534,0.3);
#11947=CIRCLE('',#35536,0.3);
#11948=CIRCLE('',#35538,0.3);
#11949=CIRCLE('',#35539,0.3);
#11950=CIRCLE('',#35541,0.299999999999999);
#11951=CIRCLE('',#35543,0.3);
#11952=CIRCLE('',#35544,0.300000000000001);
#11953=CIRCLE('',#35555,0.3);
#11954=CIRCLE('',#35556,0.300000000000001);
#11955=CIRCLE('',#35558,0.3);
#11956=CIRCLE('',#35560,0.300000000000001);
#11957=CIRCLE('',#35562,0.3);
#11958=CIRCLE('',#35564,0.3);
#11959=CIRCLE('',#35566,0.299999999999999);
#11960=CIRCLE('',#35567,16.1);
#11961=CIRCLE('',#35569,0.3);
#11962=CIRCLE('',#35571,0.300000000000001);
#11963=CIRCLE('',#35573,0.6);
#11964=CIRCLE('',#35574,15.7);
#11965=CIRCLE('',#35575,0.6);
#11966=CIRCLE('',#35577,0.300000000000001);
#11967=CIRCLE('',#35579,0.3);
#11968=CIRCLE('',#35580,0.3);
#11969=CIRCLE('',#35582,0.3);
#11970=CIRCLE('',#35584,0.3);
#11971=CIRCLE('',#35585,0.3);
#11972=CIRCLE('',#35587,0.300000000000001);
#11973=CIRCLE('',#35589,0.3);
#11974=CIRCLE('',#35590,0.3);
#11975=CIRCLE('',#35592,0.300000000000001);
#11976=CIRCLE('',#35594,0.3);
#11977=CIRCLE('',#35595,0.299999999999999);
#11978=CIRCLE('',#35597,0.3);
#11979=CIRCLE('',#35599,0.3);
#11980=CIRCLE('',#35600,0.3);
#11981=CIRCLE('',#35613,0.3);
#11982=CIRCLE('',#35614,0.300000000000001);
#11983=CIRCLE('',#35616,0.3);
#11984=CIRCLE('',#35618,0.299999999999999);
#11985=CIRCLE('',#35620,0.3);
#11986=CIRCLE('',#35622,0.3);
#11987=CIRCLE('',#35624,16.1);
#11988=CIRCLE('',#35625,0.300000000000001);
#11989=CIRCLE('',#35627,0.3);
#11990=CIRCLE('',#35629,0.300000000000001);
#11991=CIRCLE('',#35631,0.6);
#11992=CIRCLE('',#35632,15.7);
#11993=CIRCLE('',#35633,0.6);
#11994=CIRCLE('',#35635,0.300000000000001);
#11995=CIRCLE('',#35637,0.3);
#11996=CIRCLE('',#35638,0.3);
#11997=CIRCLE('',#35640,0.3);
#11998=CIRCLE('',#35642,0.3);
#11999=CIRCLE('',#35643,0.3);
#12000=CIRCLE('',#35645,0.300000000000001);
#12001=CIRCLE('',#35647,0.3);
#12002=CIRCLE('',#35648,0.3);
#12003=CIRCLE('',#35650,0.3);
#12004=CIRCLE('',#35652,0.3);
#12005=CIRCLE('',#35653,0.3);
#12006=CIRCLE('',#35655,0.299999999999999);
#12007=CIRCLE('',#35657,0.300000000000001);
#12008=CIRCLE('',#35658,0.3);
#12009=CIRCLE('',#35669,0.300000000000001);
#12010=CIRCLE('',#35670,0.3);
#12011=CIRCLE('',#35672,0.3);
#12012=CIRCLE('',#35674,0.3);
#12013=CIRCLE('',#35676,0.3);
#12014=CIRCLE('',#35678,0.3);
#12015=CIRCLE('',#35680,0.6);
#12016=CIRCLE('',#35681,15.7);
#12017=CIRCLE('',#35682,0.6);
#12018=CIRCLE('',#35683,16.1);
#12019=CIRCLE('',#35685,0.300000000000001);
#12020=CIRCLE('',#35687,0.300000000000001);
#12021=CIRCLE('',#35688,0.3);
#12022=CIRCLE('',#35690,0.3);
#12023=CIRCLE('',#35692,0.300000000000001);
#12024=CIRCLE('',#35693,0.3);
#12025=CIRCLE('',#35695,0.299999999999999);
#12026=CIRCLE('',#35696,0.3);
#12027=CIRCLE('',#35698,0.3);
#12028=CIRCLE('',#35699,0.3);
#12029=CIRCLE('',#35701,0.3);
#12030=CIRCLE('',#35702,0.3);
#12031=CIRCLE('',#35705,0.300000000000001);
#12032=CIRCLE('',#35707,0.299999999999999);
#12033=CIRCLE('',#35708,0.3);
#12034=CIRCLE('',#35710,0.300000000000001);
#12035=CIRCLE('',#35712,0.300000000000001);
#12036=CIRCLE('',#35713,0.3);
#14262=VERTEX_POINT('',#74303);
#14263=VERTEX_POINT('',#74304);
#14264=VERTEX_POINT('',#74309);
#14265=VERTEX_POINT('',#74313);
#14266=VERTEX_POINT('',#74315);
#14267=VERTEX_POINT('',#74319);
#14268=VERTEX_POINT('',#74336);
#14269=VERTEX_POINT('',#74337);
#14270=VERTEX_POINT('',#74342);
#14271=VERTEX_POINT('',#74346);
#14272=VERTEX_POINT('',#74348);
#14273=VERTEX_POINT('',#74352);
#14274=VERTEX_POINT('',#74369);
#14275=VERTEX_POINT('',#74370);
#14276=VERTEX_POINT('',#74372);
#14277=VERTEX_POINT('',#74374);
#14278=VERTEX_POINT('',#74376);
#14279=VERTEX_POINT('',#74380);
#14280=VERTEX_POINT('',#74381);
#14281=VERTEX_POINT('',#74383);
#14282=VERTEX_POINT('',#74385);
#14283=VERTEX_POINT('',#74389);
#14284=VERTEX_POINT('',#74390);
#14285=VERTEX_POINT('',#74392);
#14286=VERTEX_POINT('',#74394);
#14287=VERTEX_POINT('',#74396);
#14288=VERTEX_POINT('',#74400);
#14289=VERTEX_POINT('',#74401);
#14290=VERTEX_POINT('',#74403);
#14291=VERTEX_POINT('',#74409);
#14292=VERTEX_POINT('',#74411);
#14293=VERTEX_POINT('',#74413);
#14294=VERTEX_POINT('',#74415);
#14295=VERTEX_POINT('',#74421);
#14296=VERTEX_POINT('',#74423);
#14297=VERTEX_POINT('',#74425);
#14298=VERTEX_POINT('',#74427);
#14299=VERTEX_POINT('',#74433);
#14300=VERTEX_POINT('',#74435);
#14301=VERTEX_POINT('',#74437);
#14302=VERTEX_POINT('',#74439);
#14303=VERTEX_POINT('',#74445);
#14304=VERTEX_POINT('',#74448);
#14305=VERTEX_POINT('',#74449);
#14306=VERTEX_POINT('',#74451);
#14307=VERTEX_POINT('',#74453);
#14308=VERTEX_POINT('',#74455);
#14309=VERTEX_POINT('',#74457);
#14310=VERTEX_POINT('',#74460);
#14311=VERTEX_POINT('',#74461);
#14312=VERTEX_POINT('',#74463);
#14313=VERTEX_POINT('',#74465);
#14314=VERTEX_POINT('',#74467);
#14315=VERTEX_POINT('',#74469);
#14316=VERTEX_POINT('',#74471);
#14317=VERTEX_POINT('',#74474);
#14318=VERTEX_POINT('',#74475);
#14319=VERTEX_POINT('',#74477);
#14320=VERTEX_POINT('',#74479);
#14321=VERTEX_POINT('',#74481);
#14322=VERTEX_POINT('',#74485);
#14323=VERTEX_POINT('',#74486);
#14324=VERTEX_POINT('',#74488);
#14325=VERTEX_POINT('',#74490);
#14326=VERTEX_POINT('',#74492);
#14327=VERTEX_POINT('',#74494);
#14328=VERTEX_POINT('',#74496);
#14329=VERTEX_POINT('',#74499);
#14330=VERTEX_POINT('',#74500);
#14331=VERTEX_POINT('',#74502);
#14332=VERTEX_POINT('',#74504);
#14333=VERTEX_POINT('',#74506);
#14334=VERTEX_POINT('',#74508);
#14335=VERTEX_POINT('',#74510);
#14336=VERTEX_POINT('',#74512);
#14337=VERTEX_POINT('',#74516);
#14338=VERTEX_POINT('',#74517);
#14339=VERTEX_POINT('',#74519);
#14340=VERTEX_POINT('',#74521);
#14341=VERTEX_POINT('',#74523);
#14342=VERTEX_POINT('',#74525);
#14343=VERTEX_POINT('',#74527);
#14344=VERTEX_POINT('',#74531);
#14345=VERTEX_POINT('',#74535);
#14346=VERTEX_POINT('',#74539);
#14347=VERTEX_POINT('',#74541);
#14348=VERTEX_POINT('',#74543);
#14349=VERTEX_POINT('',#74550);
#14350=VERTEX_POINT('',#74552);
#14351=VERTEX_POINT('',#74556);
#14352=VERTEX_POINT('',#74560);
#14353=VERTEX_POINT('',#74561);
#14354=VERTEX_POINT('',#74563);
#14355=VERTEX_POINT('',#74565);
#14356=VERTEX_POINT('',#74567);
#14357=VERTEX_POINT('',#74569);
#14358=VERTEX_POINT('',#74571);
#14359=VERTEX_POINT('',#74573);
#14360=VERTEX_POINT('',#74575);
#14361=VERTEX_POINT('',#74577);
#14362=VERTEX_POINT('',#74579);
#14363=VERTEX_POINT('',#74581);
#14364=VERTEX_POINT('',#74583);
#14365=VERTEX_POINT('',#74585);
#14366=VERTEX_POINT('',#74587);
#14367=VERTEX_POINT('',#74590);
#14368=VERTEX_POINT('',#74592);
#14369=VERTEX_POINT('',#74594);
#14370=VERTEX_POINT('',#74598);
#14371=VERTEX_POINT('',#74611);
#14372=VERTEX_POINT('',#74619);
#14373=VERTEX_POINT('',#74623);
#14374=VERTEX_POINT('',#74625);
#14375=VERTEX_POINT('',#74627);
#14376=VERTEX_POINT('',#74629);
#14377=VERTEX_POINT('',#74640);
#14378=VERTEX_POINT('',#74642);
#14379=VERTEX_POINT('',#74653);
#14380=VERTEX_POINT('',#74657);
#14381=VERTEX_POINT('',#74670);
#14382=VERTEX_POINT('',#74678);
#14383=VERTEX_POINT('',#74682);
#14384=VERTEX_POINT('',#74683);
#14385=VERTEX_POINT('',#74685);
#14386=VERTEX_POINT('',#74687);
#14387=VERTEX_POINT('',#74689);
#14388=VERTEX_POINT('',#74691);
#14389=VERTEX_POINT('',#74693);
#14390=VERTEX_POINT('',#74695);
#14391=VERTEX_POINT('',#74697);
#14392=VERTEX_POINT('',#74699);
#14393=VERTEX_POINT('',#74701);
#14394=VERTEX_POINT('',#74703);
#14395=VERTEX_POINT('',#74705);
#14396=VERTEX_POINT('',#74707);
#14397=VERTEX_POINT('',#74710);
#14398=VERTEX_POINT('',#74712);
#14399=VERTEX_POINT('',#74714);
#14400=VERTEX_POINT('',#74718);
#14401=VERTEX_POINT('',#74731);
#14402=VERTEX_POINT('',#74739);
#14403=VERTEX_POINT('',#74743);
#14404=VERTEX_POINT('',#74745);
#14405=VERTEX_POINT('',#74747);
#14406=VERTEX_POINT('',#74749);
#14407=VERTEX_POINT('',#74760);
#14408=VERTEX_POINT('',#74762);
#14409=VERTEX_POINT('',#74773);
#14410=VERTEX_POINT('',#74777);
#14411=VERTEX_POINT('',#74790);
#14412=VERTEX_POINT('',#74800);
#14413=VERTEX_POINT('',#74802);
#14414=VERTEX_POINT('',#74804);
#14415=VERTEX_POINT('',#74806);
#14416=VERTEX_POINT('',#74810);
#14417=VERTEX_POINT('',#74812);
#14418=VERTEX_POINT('',#74816);
#14419=VERTEX_POINT('',#74818);
#14420=VERTEX_POINT('',#74820);
#14421=VERTEX_POINT('',#74822);
#14422=VERTEX_POINT('',#74826);
#14423=VERTEX_POINT('',#74830);
#14424=VERTEX_POINT('',#74831);
#14425=VERTEX_POINT('',#74833);
#14426=VERTEX_POINT('',#74835);
#14427=VERTEX_POINT('',#74840);
#14428=VERTEX_POINT('',#74844);
#14429=VERTEX_POINT('',#74846);
#14430=VERTEX_POINT('',#74848);
#14431=VERTEX_POINT('',#74852);
#14432=VERTEX_POINT('',#74854);
#14433=VERTEX_POINT('',#74858);
#14434=VERTEX_POINT('',#74862);
#14435=VERTEX_POINT('',#74864);
#14436=VERTEX_POINT('',#74868);
#14437=VERTEX_POINT('',#74872);
#14438=VERTEX_POINT('',#74874);
#14439=VERTEX_POINT('',#74880);
#14440=VERTEX_POINT('',#74890);
#14441=VERTEX_POINT('',#74892);
#14442=VERTEX_POINT('',#74896);
#14443=VERTEX_POINT('',#74900);
#14444=VERTEX_POINT('',#74902);
#14445=VERTEX_POINT('',#74906);
#14446=VERTEX_POINT('',#74908);
#14447=VERTEX_POINT('',#74912);
#14448=VERTEX_POINT('',#74916);
#14449=VERTEX_POINT('',#74920);
#14450=VERTEX_POINT('',#74922);
#14451=VERTEX_POINT('',#74925);
#14452=VERTEX_POINT('',#74927);
#14453=VERTEX_POINT('',#74931);
#14454=VERTEX_POINT('',#74935);
#14455=VERTEX_POINT('',#74939);
#14456=VERTEX_POINT('',#74943);
#14457=VERTEX_POINT('',#74947);
#14458=VERTEX_POINT('',#74951);
#14459=VERTEX_POINT('',#74955);
#14460=VERTEX_POINT('',#74959);
#14461=VERTEX_POINT('',#74965);
#14462=VERTEX_POINT('',#74967);
#14463=VERTEX_POINT('',#74971);
#14464=VERTEX_POINT('',#74975);
#14465=VERTEX_POINT('',#74977);
#14466=VERTEX_POINT('',#74981);
#14467=VERTEX_POINT('',#74983);
#14468=VERTEX_POINT('',#74987);
#14469=VERTEX_POINT('',#74991);
#14470=VERTEX_POINT('',#74995);
#14471=VERTEX_POINT('',#74996);
#14472=VERTEX_POINT('',#74998);
#14473=VERTEX_POINT('',#75002);
#14474=VERTEX_POINT('',#75004);
#14475=VERTEX_POINT('',#75011);
#14476=VERTEX_POINT('',#75015);
#14477=VERTEX_POINT('',#75016);
#14478=VERTEX_POINT('',#75018);
#14479=VERTEX_POINT('',#75020);
#14480=VERTEX_POINT('',#75023);
#14481=VERTEX_POINT('',#75025);
#14482=VERTEX_POINT('',#75029);
#14483=VERTEX_POINT('',#75033);
#14484=VERTEX_POINT('',#75034);
#14485=VERTEX_POINT('',#75036);
#14486=VERTEX_POINT('',#75039);
#14487=VERTEX_POINT('',#75041);
#14488=VERTEX_POINT('',#75045);
#14489=VERTEX_POINT('',#75053);
#14490=VERTEX_POINT('',#75059);
#14491=VERTEX_POINT('',#75063);
#14492=VERTEX_POINT('',#75065);
#14493=VERTEX_POINT('',#75067);
#14494=VERTEX_POINT('',#75069);
#14495=VERTEX_POINT('',#75071);
#14496=VERTEX_POINT('',#75073);
#14497=VERTEX_POINT('',#75077);
#14498=VERTEX_POINT('',#75081);
#14499=VERTEX_POINT('',#75083);
#14500=VERTEX_POINT('',#75085);
#14501=VERTEX_POINT('',#75087);
#14502=VERTEX_POINT('',#75089);
#14503=VERTEX_POINT('',#75093);
#14504=VERTEX_POINT('',#75095);
#14505=VERTEX_POINT('',#75121);
#14506=VERTEX_POINT('',#75130);
#14507=VERTEX_POINT('',#75137);
#14508=VERTEX_POINT('',#75145);
#14509=VERTEX_POINT('',#75155);
#14510=VERTEX_POINT('',#75162);
#14511=VERTEX_POINT('',#75172);
#14512=VERTEX_POINT('',#75184);
#14513=VERTEX_POINT('',#75191);
#14514=VERTEX_POINT('',#75195);
#14515=VERTEX_POINT('',#75196);
#14516=VERTEX_POINT('',#75198);
#14517=VERTEX_POINT('',#75200);
#14518=VERTEX_POINT('',#75202);
#14519=VERTEX_POINT('',#75204);
#14520=VERTEX_POINT('',#75206);
#14521=VERTEX_POINT('',#75208);
#14522=VERTEX_POINT('',#75210);
#14523=VERTEX_POINT('',#75213);
#14524=VERTEX_POINT('',#75215);
#14525=VERTEX_POINT('',#75220);
#14526=VERTEX_POINT('',#75225);
#14527=VERTEX_POINT('',#75229);
#14528=VERTEX_POINT('',#75242);
#14529=VERTEX_POINT('',#75256);
#14530=VERTEX_POINT('',#75257);
#14531=VERTEX_POINT('',#75262);
#14532=VERTEX_POINT('',#75263);
#14533=VERTEX_POINT('',#75265);
#14534=VERTEX_POINT('',#75267);
#14535=VERTEX_POINT('',#75271);
#14536=VERTEX_POINT('',#75272);
#14537=VERTEX_POINT('',#75274);
#14538=VERTEX_POINT('',#75276);
#14539=VERTEX_POINT('',#75280);
#14540=VERTEX_POINT('',#75281);
#14541=VERTEX_POINT('',#75283);
#14542=VERTEX_POINT('',#75285);
#14543=VERTEX_POINT('',#75289);
#14544=VERTEX_POINT('',#75290);
#14545=VERTEX_POINT('',#75292);
#14546=VERTEX_POINT('',#75294);
#14547=VERTEX_POINT('',#75298);
#14548=VERTEX_POINT('',#75299);
#14549=VERTEX_POINT('',#75310);
#14550=VERTEX_POINT('',#75311);
#14551=VERTEX_POINT('',#75313);
#14552=VERTEX_POINT('',#75323);
#14553=VERTEX_POINT('',#75325);
#14554=VERTEX_POINT('',#75329);
#14555=VERTEX_POINT('',#75330);
#14556=VERTEX_POINT('',#75332);
#14557=VERTEX_POINT('',#75334);
#14558=VERTEX_POINT('',#75336);
#14559=VERTEX_POINT('',#75365);
#14560=VERTEX_POINT('',#75369);
#14561=VERTEX_POINT('',#75370);
#14562=VERTEX_POINT('',#75373);
#14563=VERTEX_POINT('',#75375);
#14564=VERTEX_POINT('',#75377);
#14565=VERTEX_POINT('',#75379);
#14566=VERTEX_POINT('',#75381);
#14567=VERTEX_POINT('',#75384);
#14568=VERTEX_POINT('',#75386);
#14569=VERTEX_POINT('',#75388);
#14570=VERTEX_POINT('',#75390);
#14571=VERTEX_POINT('',#75392);
#14572=VERTEX_POINT('',#75395);
#14573=VERTEX_POINT('',#75397);
#14574=VERTEX_POINT('',#75399);
#14575=VERTEX_POINT('',#75401);
#14576=VERTEX_POINT('',#75414);
#14577=VERTEX_POINT('',#75440);
#14578=VERTEX_POINT('',#75444);
#14579=VERTEX_POINT('',#75446);
#14580=VERTEX_POINT('',#75450);
#14581=VERTEX_POINT('',#75452);
#14582=VERTEX_POINT('',#75456);
#14583=VERTEX_POINT('',#75457);
#14584=VERTEX_POINT('',#75459);
#14585=VERTEX_POINT('',#75461);
#14586=VERTEX_POINT('',#75465);
#14587=VERTEX_POINT('',#75466);
#14588=VERTEX_POINT('',#75468);
#14589=VERTEX_POINT('',#75470);
#14590=VERTEX_POINT('',#75474);
#14591=VERTEX_POINT('',#75475);
#14592=VERTEX_POINT('',#75491);
#14593=VERTEX_POINT('',#75493);
#14594=VERTEX_POINT('',#75495);
#14595=VERTEX_POINT('',#75507);
#14596=VERTEX_POINT('',#75508);
#14597=VERTEX_POINT('',#75511);
#14598=VERTEX_POINT('',#75513);
#14599=VERTEX_POINT('',#75544);
#14600=VERTEX_POINT('',#75546);
#14601=VERTEX_POINT('',#75548);
#14602=VERTEX_POINT('',#75550);
#14603=VERTEX_POINT('',#75552);
#14604=VERTEX_POINT('',#75555);
#14605=VERTEX_POINT('',#75557);
#14606=VERTEX_POINT('',#75570);
#14607=VERTEX_POINT('',#75583);
#14608=VERTEX_POINT('',#75596);
#14609=VERTEX_POINT('',#75598);
#14610=VERTEX_POINT('',#75601);
#14611=VERTEX_POINT('',#75603);
#14612=VERTEX_POINT('',#75605);
#14613=VERTEX_POINT('',#75607);
#14614=VERTEX_POINT('',#75609);
#14615=VERTEX_POINT('',#75613);
#14616=VERTEX_POINT('',#75616);
#14617=VERTEX_POINT('',#75618);
#14618=VERTEX_POINT('',#75622);
#14619=VERTEX_POINT('',#75626);
#14620=VERTEX_POINT('',#75630);
#14621=VERTEX_POINT('',#75634);
#14622=VERTEX_POINT('',#75638);
#14623=VERTEX_POINT('',#75642);
#14624=VERTEX_POINT('',#75646);
#14625=VERTEX_POINT('',#75652);
#14626=VERTEX_POINT('',#75656);
#14627=VERTEX_POINT('',#75660);
#14628=VERTEX_POINT('',#75663);
#14629=VERTEX_POINT('',#75664);
#14630=VERTEX_POINT('',#75669);
#14631=VERTEX_POINT('',#75696);
#14632=VERTEX_POINT('',#75734);
#14633=VERTEX_POINT('',#75772);
#14634=VERTEX_POINT('',#75804);
#14635=VERTEX_POINT('',#75806);
#14636=VERTEX_POINT('',#75854);
#14637=VERTEX_POINT('',#75855);
#14638=VERTEX_POINT('',#75868);
#14639=VERTEX_POINT('',#75872);
#14640=VERTEX_POINT('',#75873);
#14641=VERTEX_POINT('',#75895);
#14642=VERTEX_POINT('',#75924);
#14643=VERTEX_POINT('',#75926);
#14644=VERTEX_POINT('',#75980);
#14645=VERTEX_POINT('',#75982);
#14646=VERTEX_POINT('',#76020);
#14647=VERTEX_POINT('',#76058);
#14648=VERTEX_POINT('',#76073);
#14649=VERTEX_POINT('',#76077);
#14650=VERTEX_POINT('',#76081);
#14651=VERTEX_POINT('',#76085);
#14652=VERTEX_POINT('',#76087);
#14653=VERTEX_POINT('',#76089);
#14654=VERTEX_POINT('',#76091);
#14655=VERTEX_POINT('',#76095);
#14656=VERTEX_POINT('',#76098);
#14657=VERTEX_POINT('',#76101);
#14658=VERTEX_POINT('',#76106);
#14659=VERTEX_POINT('',#76108);
#14660=VERTEX_POINT('',#76112);
#14661=VERTEX_POINT('',#76114);
#14662=VERTEX_POINT('',#76121);
#14663=VERTEX_POINT('',#76125);
#14664=VERTEX_POINT('',#76127);
#14665=VERTEX_POINT('',#76131);
#14666=VERTEX_POINT('',#76133);
#14667=VERTEX_POINT('',#76137);
#14668=VERTEX_POINT('',#76139);
#14669=VERTEX_POINT('',#76143);
#14670=VERTEX_POINT('',#76145);
#14671=VERTEX_POINT('',#76147);
#14672=VERTEX_POINT('',#76149);
#14673=VERTEX_POINT('',#76151);
#14674=VERTEX_POINT('',#76153);
#14675=VERTEX_POINT('',#76155);
#14676=VERTEX_POINT('',#76159);
#14677=VERTEX_POINT('',#76160);
#14678=VERTEX_POINT('',#76163);
#14679=VERTEX_POINT('',#76165);
#14680=VERTEX_POINT('',#76167);
#14681=VERTEX_POINT('',#76169);
#14682=VERTEX_POINT('',#76171);
#14683=VERTEX_POINT('',#76176);
#14684=VERTEX_POINT('',#76177);
#14685=VERTEX_POINT('',#76179);
#14686=VERTEX_POINT('',#76181);
#14687=VERTEX_POINT('',#76185);
#14688=VERTEX_POINT('',#76186);
#14689=VERTEX_POINT('',#76220);
#14690=VERTEX_POINT('',#76236);
#14691=VERTEX_POINT('',#76271);
#14692=VERTEX_POINT('',#76272);
#14693=VERTEX_POINT('',#76328);
#14694=VERTEX_POINT('',#76347);
#14695=VERTEX_POINT('',#76368);
#14696=VERTEX_POINT('',#76370);
#14697=VERTEX_POINT('',#76409);
#14698=VERTEX_POINT('',#76410);
#14699=VERTEX_POINT('',#76466);
#14700=VERTEX_POINT('',#76476);
#14701=VERTEX_POINT('',#76517);
#14702=VERTEX_POINT('',#76518);
#14703=VERTEX_POINT('',#76551);
#14704=VERTEX_POINT('',#76552);
#14705=VERTEX_POINT('',#76560);
#14706=VERTEX_POINT('',#76564);
#14707=VERTEX_POINT('',#76571);
#14708=VERTEX_POINT('',#76573);
#14709=VERTEX_POINT('',#76600);
#14710=VERTEX_POINT('',#76601);
#14711=VERTEX_POINT('',#76608);
#14712=VERTEX_POINT('',#76618);
#14713=VERTEX_POINT('',#76632);
#14714=VERTEX_POINT('',#76634);
#14715=VERTEX_POINT('',#76678);
#14716=VERTEX_POINT('',#76680);
#14717=VERTEX_POINT('',#76689);
#14718=VERTEX_POINT('',#76691);
#14719=VERTEX_POINT('',#76705);
#14720=VERTEX_POINT('',#76712);
#14721=VERTEX_POINT('',#76720);
#14722=VERTEX_POINT('',#76727);
#14723=VERTEX_POINT('',#76734);
#14724=VERTEX_POINT('',#76750);
#14725=VERTEX_POINT('',#76775);
#14726=VERTEX_POINT('',#76782);
#14727=VERTEX_POINT('',#76784);
#14728=VERTEX_POINT('',#76786);
#14729=VERTEX_POINT('',#76806);
#14730=VERTEX_POINT('',#76808);
#14731=VERTEX_POINT('',#76810);
#14732=VERTEX_POINT('',#76812);
#14733=VERTEX_POINT('',#76821);
#14734=VERTEX_POINT('',#76834);
#14735=VERTEX_POINT('',#76837);
#14736=VERTEX_POINT('',#76842);
#14737=VERTEX_POINT('',#76852);
#14738=VERTEX_POINT('',#76854);
#14739=VERTEX_POINT('',#76861);
#14740=VERTEX_POINT('',#76877);
#14741=VERTEX_POINT('',#76891);
#14742=VERTEX_POINT('',#76892);
#14743=VERTEX_POINT('',#76908);
#14744=VERTEX_POINT('',#76915);
#14745=VERTEX_POINT('',#76917);
#14746=VERTEX_POINT('',#76919);
#14747=VERTEX_POINT('',#76921);
#14748=VERTEX_POINT('',#76923);
#14749=VERTEX_POINT('',#76925);
#14750=VERTEX_POINT('',#76950);
#14751=VERTEX_POINT('',#76951);
#14752=VERTEX_POINT('',#76961);
#14753=VERTEX_POINT('',#76979);
#14754=VERTEX_POINT('',#76981);
#14755=VERTEX_POINT('',#76994);
#14756=VERTEX_POINT('',#77009);
#14757=VERTEX_POINT('',#77012);
#14758=VERTEX_POINT('',#77013);
#14759=VERTEX_POINT('',#77015);
#14760=VERTEX_POINT('',#77017);
#14761=VERTEX_POINT('',#77019);
#14762=VERTEX_POINT('',#77021);
#14763=VERTEX_POINT('',#77023);
#14764=VERTEX_POINT('',#77030);
#14765=VERTEX_POINT('',#77046);
#14766=VERTEX_POINT('',#77072);
#14767=VERTEX_POINT('',#77113);
#14768=VERTEX_POINT('',#77134);
#14769=VERTEX_POINT('',#77135);
#14770=VERTEX_POINT('',#77153);
#14771=VERTEX_POINT('',#77163);
#14772=VERTEX_POINT('',#77165);
#14773=VERTEX_POINT('',#77167);
#14774=VERTEX_POINT('',#77182);
#14775=VERTEX_POINT('',#77196);
#14776=VERTEX_POINT('',#77278);
#14777=VERTEX_POINT('',#77280);
#14778=VERTEX_POINT('',#77295);
#14779=VERTEX_POINT('',#77316);
#14780=VERTEX_POINT('',#77339);
#14781=VERTEX_POINT('',#77377);
#14782=VERTEX_POINT('',#77406);
#14783=VERTEX_POINT('',#77444);
#14784=VERTEX_POINT('',#77462);
#14785=VERTEX_POINT('',#77466);
#14786=VERTEX_POINT('',#77501);
#14787=VERTEX_POINT('',#77502);
#14788=VERTEX_POINT('',#77538);
#14789=VERTEX_POINT('',#77539);
#14790=VERTEX_POINT('',#77552);
#14791=VERTEX_POINT('',#77556);
#14792=VERTEX_POINT('',#77562);
#14793=VERTEX_POINT('',#77589);
#14794=VERTEX_POINT('',#77615);
#14795=VERTEX_POINT('',#77653);
#14796=VERTEX_POINT('',#77718);
#14797=VERTEX_POINT('',#77720);
#14798=VERTEX_POINT('',#77749);
#14799=VERTEX_POINT('',#77758);
#14800=VERTEX_POINT('',#77762);
#14801=VERTEX_POINT('',#77766);
#14802=VERTEX_POINT('',#77770);
#14803=VERTEX_POINT('',#77774);
#14804=VERTEX_POINT('',#77807);
#14805=VERTEX_POINT('',#77966);
#14806=VERTEX_POINT('',#77967);
#14807=VERTEX_POINT('',#77972);
#14808=VERTEX_POINT('',#77976);
#14809=VERTEX_POINT('',#77980);
#14810=VERTEX_POINT('',#77984);
#14811=VERTEX_POINT('',#77999);
#14812=VERTEX_POINT('',#78037);
#14813=VERTEX_POINT('',#78072);
#14814=VERTEX_POINT('',#78139);
#14815=VERTEX_POINT('',#78141);
#14816=VERTEX_POINT('',#78143);
#14817=VERTEX_POINT('',#78147);
#14818=VERTEX_POINT('',#78149);
#14819=VERTEX_POINT('',#78151);
#14820=VERTEX_POINT('',#78153);
#14821=VERTEX_POINT('',#78157);
#14822=VERTEX_POINT('',#78159);
#14823=VERTEX_POINT('',#78161);
#14824=VERTEX_POINT('',#78163);
#14825=VERTEX_POINT('',#78167);
#14826=VERTEX_POINT('',#78169);
#14827=VERTEX_POINT('',#78171);
#14828=VERTEX_POINT('',#78175);
#14829=VERTEX_POINT('',#78177);
#14830=VERTEX_POINT('',#78179);
#14831=VERTEX_POINT('',#78183);
#14832=VERTEX_POINT('',#78185);
#14833=VERTEX_POINT('',#78187);
#14834=VERTEX_POINT('',#78189);
#14835=VERTEX_POINT('',#78193);
#14836=VERTEX_POINT('',#78195);
#14837=VERTEX_POINT('',#78197);
#14838=VERTEX_POINT('',#78199);
#14839=VERTEX_POINT('',#78203);
#14840=VERTEX_POINT('',#78205);
#14841=VERTEX_POINT('',#78207);
#14842=VERTEX_POINT('',#78213);
#14843=VERTEX_POINT('',#78217);
#14844=VERTEX_POINT('',#78219);
#14845=VERTEX_POINT('',#78224);
#14846=VERTEX_POINT('',#78226);
#14847=VERTEX_POINT('',#78229);
#14848=VERTEX_POINT('',#78231);
#14849=VERTEX_POINT('',#78234);
#14850=VERTEX_POINT('',#78237);
#14851=VERTEX_POINT('',#78240);
#14852=VERTEX_POINT('',#78242);
#14853=VERTEX_POINT('',#78248);
#14854=VERTEX_POINT('',#78252);
#14855=VERTEX_POINT('',#78254);
#14856=VERTEX_POINT('',#78262);
#14857=VERTEX_POINT('',#78268);
#14858=VERTEX_POINT('',#78276);
#14859=VERTEX_POINT('',#78278);
#14860=VERTEX_POINT('',#78280);
#14861=VERTEX_POINT('',#78282);
#14862=VERTEX_POINT('',#78284);
#14863=VERTEX_POINT('',#78286);
#14864=VERTEX_POINT('',#78288);
#14865=VERTEX_POINT('',#78292);
#14866=VERTEX_POINT('',#78301);
#14867=VERTEX_POINT('',#78305);
#14868=VERTEX_POINT('',#78333);
#14869=VERTEX_POINT('',#78335);
#14870=VERTEX_POINT('',#78339);
#14871=VERTEX_POINT('',#78341);
#14872=VERTEX_POINT('',#78349);
#14873=VERTEX_POINT('',#78355);
#14874=VERTEX_POINT('',#78359);
#14875=VERTEX_POINT('',#78365);
#14876=VERTEX_POINT('',#78367);
#14877=VERTEX_POINT('',#78369);
#14878=VERTEX_POINT('',#78371);
#14879=VERTEX_POINT('',#78373);
#14880=VERTEX_POINT('',#78375);
#14881=VERTEX_POINT('',#78377);
#14882=VERTEX_POINT('',#78381);
#14883=VERTEX_POINT('',#78385);
#14884=VERTEX_POINT('',#78389);
#14885=VERTEX_POINT('',#78393);
#14886=VERTEX_POINT('',#78397);
#14887=VERTEX_POINT('',#78401);
#14888=VERTEX_POINT('',#78405);
#14889=VERTEX_POINT('',#78414);
#14890=VERTEX_POINT('',#78438);
#14891=VERTEX_POINT('',#78440);
#14892=VERTEX_POINT('',#78448);
#14893=VERTEX_POINT('',#78454);
#14894=VERTEX_POINT('',#78462);
#14895=VERTEX_POINT('',#78464);
#14896=VERTEX_POINT('',#78466);
#14897=VERTEX_POINT('',#78468);
#14898=VERTEX_POINT('',#78470);
#14899=VERTEX_POINT('',#78472);
#14900=VERTEX_POINT('',#78474);
#14901=VERTEX_POINT('',#78478);
#14902=VERTEX_POINT('',#78487);
#14903=VERTEX_POINT('',#78491);
#14904=VERTEX_POINT('',#78519);
#14905=VERTEX_POINT('',#78521);
#14906=VERTEX_POINT('',#78525);
#14907=VERTEX_POINT('',#78527);
#14908=VERTEX_POINT('',#78531);
#14909=VERTEX_POINT('',#78541);
#14910=VERTEX_POINT('',#78543);
#14911=VERTEX_POINT('',#78545);
#14912=VERTEX_POINT('',#78547);
#14913=VERTEX_POINT('',#78549);
#14914=VERTEX_POINT('',#78551);
#14915=VERTEX_POINT('',#78553);
#14916=VERTEX_POINT('',#78555);
#14917=VERTEX_POINT('',#78559);
#14918=VERTEX_POINT('',#78563);
#14919=VERTEX_POINT('',#78569);
#14920=VERTEX_POINT('',#78573);
#14921=VERTEX_POINT('',#78575);
#14922=VERTEX_POINT('',#78579);
#14923=VERTEX_POINT('',#78583);
#14924=VERTEX_POINT('',#78589);
#14925=VERTEX_POINT('',#78598);
#17740=EDGE_CURVE('',#14262,#14263,#1636,.T.);
#17741=EDGE_CURVE('',#14264,#14263,#7949,.T.);
#17742=EDGE_CURVE('',#14262,#14264,#11640,.T.);
#17743=EDGE_CURVE('',#14262,#14265,#7950,.T.);
#17744=EDGE_CURVE('',#14266,#14264,#7951,.T.);
#17745=EDGE_CURVE('',#14265,#14266,#11641,.T.);
#17746=EDGE_CURVE('',#14267,#14263,#7952,.T.);
#17747=EDGE_CURVE('',#14266,#14267,#7953,.T.);
#17748=EDGE_CURVE('',#14265,#14267,#1637,.T.);
#17749=EDGE_CURVE('',#14268,#14269,#1638,.T.);
#17750=EDGE_CURVE('',#14268,#14270,#11642,.T.);
#17751=EDGE_CURVE('',#14270,#14269,#7954,.T.);
#17752=EDGE_CURVE('',#14271,#14270,#7955,.T.);
#17753=EDGE_CURVE('',#14271,#14272,#7956,.T.);
#17754=EDGE_CURVE('',#14272,#14269,#7957,.T.);
#17755=EDGE_CURVE('',#14273,#14268,#7958,.T.);
#17756=EDGE_CURVE('',#14273,#14271,#11643,.T.);
#17757=EDGE_CURVE('',#14273,#14272,#1639,.T.);
#17758=EDGE_CURVE('',#14274,#14275,#11644,.T.);
#17759=EDGE_CURVE('',#14275,#14276,#7959,.T.);
#17760=EDGE_CURVE('',#14277,#14276,#11645,.T.);
#17761=EDGE_CURVE('',#14278,#14277,#11646,.T.);
#17762=EDGE_CURVE('',#14274,#14278,#7960,.T.);
#17763=EDGE_CURVE('',#14279,#14280,#11647,.T.);
#17764=EDGE_CURVE('',#14281,#14279,#7961,.T.);
#17765=EDGE_CURVE('',#14281,#14282,#11648,.T.);
#17766=EDGE_CURVE('',#14282,#14280,#7962,.T.);
#17767=EDGE_CURVE('',#14283,#14284,#7963,.T.);
#17768=EDGE_CURVE('',#14284,#14285,#7964,.T.);
#17769=EDGE_CURVE('',#14285,#14286,#7965,.T.);
#17770=EDGE_CURVE('',#14287,#14286,#7966,.T.);
#17771=EDGE_CURVE('',#14283,#14287,#7967,.T.);
#17772=EDGE_CURVE('',#14288,#14289,#7968,.T.);
#17773=EDGE_CURVE('',#14290,#14289,#1640,.T.);
#17774=EDGE_CURVE('',#14291,#14290,#7969,.T.);
#17775=EDGE_CURVE('',#14292,#14291,#11649,.T.);
#17776=EDGE_CURVE('',#14292,#14293,#7970,.T.);
#17777=EDGE_CURVE('',#14293,#14294,#1641,.T.);
#17778=EDGE_CURVE('',#14294,#14295,#7971,.T.);
#17779=EDGE_CURVE('',#14295,#14296,#11650,.T.);
#17780=EDGE_CURVE('',#14296,#14297,#7972,.T.);
#17781=EDGE_CURVE('',#14297,#14298,#1642,.T.);
#17782=EDGE_CURVE('',#14298,#14299,#7973,.T.);
#17783=EDGE_CURVE('',#14300,#14299,#11651,.T.);
#17784=EDGE_CURVE('',#14301,#14300,#7974,.T.);
#17785=EDGE_CURVE('',#14302,#14301,#1643,.T.);
#17786=EDGE_CURVE('',#14302,#14303,#7975,.T.);
#17787=EDGE_CURVE('',#14288,#14303,#11652,.T.);
#17788=EDGE_CURVE('',#14304,#14305,#7976,.T.);
#17789=EDGE_CURVE('',#14304,#14306,#11653,.T.);
#17790=EDGE_CURVE('',#14306,#14307,#11654,.T.);
#17791=EDGE_CURVE('',#14308,#14307,#11655,.T.);
#17792=EDGE_CURVE('',#14308,#14309,#7977,.T.);
#17793=EDGE_CURVE('',#14309,#14305,#11656,.T.);
#17794=EDGE_CURVE('',#14310,#14311,#11657,.T.);
#17795=EDGE_CURVE('',#14310,#14312,#11658,.T.);
#17796=EDGE_CURVE('',#14313,#14312,#7978,.T.);
#17797=EDGE_CURVE('',#14314,#14313,#7979,.T.);
#17798=EDGE_CURVE('',#14314,#14315,#11659,.T.);
#17799=EDGE_CURVE('',#14316,#14315,#7980,.T.);
#17800=EDGE_CURVE('',#14316,#14311,#7981,.T.);
#17801=EDGE_CURVE('',#14317,#14318,#7982,.T.);
#17802=EDGE_CURVE('',#14318,#14319,#7983,.T.);
#17803=EDGE_CURVE('',#14320,#14319,#11660,.T.);
#17804=EDGE_CURVE('',#14320,#14321,#11661,.T.);
#17805=EDGE_CURVE('',#14283,#14321,#7984,.T.);
#17806=EDGE_CURVE('',#14287,#14317,#11662,.T.);
#17807=EDGE_CURVE('',#14322,#14323,#11663,.T.);
#17808=EDGE_CURVE('',#14323,#14324,#11664,.T.);
#17809=EDGE_CURVE('',#14324,#14325,#7985,.T.);
#17810=EDGE_CURVE('',#14325,#14326,#7986,.T.);
#17811=EDGE_CURVE('',#14326,#14327,#11665,.T.);
#17812=EDGE_CURVE('',#14328,#14327,#7987,.T.);
#17813=EDGE_CURVE('',#14328,#14322,#11666,.T.);
#17814=EDGE_CURVE('',#14329,#14330,#7988,.T.);
#17815=EDGE_CURVE('',#14330,#14331,#11667,.T.);
#17816=EDGE_CURVE('',#14331,#14332,#11668,.T.);
#17817=EDGE_CURVE('',#14332,#14333,#11669,.T.);
#17818=EDGE_CURVE('',#14333,#14334,#11670,.T.);
#17819=EDGE_CURVE('',#14335,#14334,#11671,.T.);
#17820=EDGE_CURVE('',#14335,#14336,#11672,.T.);
#17821=EDGE_CURVE('',#14282,#14336,#7989,.T.);
#17822=EDGE_CURVE('',#14281,#14329,#11673,.T.);
#17823=EDGE_CURVE('',#14337,#14338,#11674,.T.);
#17824=EDGE_CURVE('',#14339,#14338,#11675,.T.);
#17825=EDGE_CURVE('',#14339,#14340,#7990,.T.);
#17826=EDGE_CURVE('',#14340,#14341,#11676,.T.);
#17827=EDGE_CURVE('',#14342,#14341,#7991,.T.);
#17828=EDGE_CURVE('',#14343,#14342,#7992,.T.);
#17829=EDGE_CURVE('',#14337,#14343,#11677,.T.);
#17830=EDGE_CURVE('',#14286,#14344,#11678,.T.);
#17831=EDGE_CURVE('',#14317,#14344,#7993,.T.);
#17832=EDGE_CURVE('',#14285,#14345,#587,.T.);
#17833=EDGE_CURVE('',#14344,#14345,#7994,.T.);
#17834=EDGE_CURVE('',#14284,#14346,#7995,.T.);
#17835=EDGE_CURVE('',#14347,#14346,#588,.T.);
#17836=EDGE_CURVE('',#14348,#14347,#1644,.T.);
#17837=EDGE_CURVE('',#14348,#14349,#11679,.T.);
#17838=EDGE_CURVE('',#14350,#14349,#7996,.T.);
#17839=EDGE_CURVE('',#14345,#14350,#7997,.T.);
#17840=EDGE_CURVE('',#14321,#14351,#7998,.T.);
#17841=EDGE_CURVE('',#14346,#14351,#7999,.T.);
#17842=EDGE_CURVE('',#14352,#14353,#8000,.T.);
#17843=EDGE_CURVE('',#14353,#14354,#11680,.T.);
#17844=EDGE_CURVE('',#14355,#14354,#8001,.T.);
#17845=EDGE_CURVE('',#14355,#14356,#11681,.T.);
#17846=EDGE_CURVE('',#14357,#14356,#8002,.T.);
#17847=EDGE_CURVE('',#14357,#14358,#11682,.T.);
#17848=EDGE_CURVE('',#14358,#14359,#8003,.T.);
#17849=EDGE_CURVE('',#14359,#14360,#11683,.T.);
#17850=EDGE_CURVE('',#14360,#14361,#8004,.T.);
#17851=EDGE_CURVE('',#14361,#14362,#11684,.T.);
#17852=EDGE_CURVE('',#14363,#14362,#8005,.T.);
#17853=EDGE_CURVE('',#14363,#14364,#11685,.T.);
#17854=EDGE_CURVE('',#14364,#14365,#8006,.T.);
#17855=EDGE_CURVE('',#14365,#14366,#11686,.T.);
#17856=EDGE_CURVE('',#14366,#14288,#8007,.T.);
#17857=EDGE_CURVE('',#14367,#14303,#8008,.T.);
#17858=EDGE_CURVE('',#14367,#14368,#11687,.T.);
#17859=EDGE_CURVE('',#14369,#14368,#8009,.T.);
#17860=EDGE_CURVE('',#14369,#14352,#11688,.T.);
#17861=EDGE_CURVE('',#14302,#14370,#8010,.T.);
#17862=EDGE_CURVE('',#14370,#14367,#8011,.T.);
#17863=EDGE_CURVE('',#14301,#14371,#8012,.T.);
#17864=EDGE_CURVE('',#14370,#14371,#1645,.T.);
#17865=EDGE_CURVE('',#14371,#14372,#8013,.T.);
#17866=EDGE_CURVE('',#14300,#14372,#8014,.T.);
#17867=EDGE_CURVE('',#14299,#14373,#8015,.T.);
#17868=EDGE_CURVE('',#14373,#14374,#11689,.T.);
#17869=EDGE_CURVE('',#14375,#14374,#8016,.T.);
#17870=EDGE_CURVE('',#14376,#14375,#1646,.T.);
#17871=EDGE_CURVE('',#14376,#14377,#11690,.T.);
#17872=EDGE_CURVE('',#14378,#14377,#1647,.T.);
#17873=EDGE_CURVE('',#14378,#14379,#8017,.T.);
#17874=EDGE_CURVE('',#14379,#14372,#11691,.T.);
#17875=EDGE_CURVE('',#14298,#14380,#8018,.T.);
#17876=EDGE_CURVE('',#14380,#14373,#8019,.T.);
#17877=EDGE_CURVE('',#14297,#14381,#8020,.T.);
#17878=EDGE_CURVE('',#14381,#14380,#1648,.T.);
#17879=EDGE_CURVE('',#14382,#14296,#8021,.T.);
#17880=EDGE_CURVE('',#14382,#14381,#8022,.T.);
#17881=EDGE_CURVE('',#14383,#14384,#8023,.T.);
#17882=EDGE_CURVE('',#14385,#14384,#11692,.T.);
#17883=EDGE_CURVE('',#14386,#14385,#8024,.T.);
#17884=EDGE_CURVE('',#14386,#14387,#11693,.T.);
#17885=EDGE_CURVE('',#14388,#14387,#8025,.T.);
#17886=EDGE_CURVE('',#14389,#14388,#11694,.T.);
#17887=EDGE_CURVE('',#14389,#14390,#8026,.T.);
#17888=EDGE_CURVE('',#14390,#14391,#11695,.T.);
#17889=EDGE_CURVE('',#14391,#14392,#8027,.T.);
#17890=EDGE_CURVE('',#14393,#14392,#11696,.T.);
#17891=EDGE_CURVE('',#14394,#14393,#8028,.T.);
#17892=EDGE_CURVE('',#14394,#14395,#11697,.T.);
#17893=EDGE_CURVE('',#14395,#14396,#8029,.T.);
#17894=EDGE_CURVE('',#14396,#14382,#11698,.T.);
#17895=EDGE_CURVE('',#14397,#14295,#8030,.T.);
#17896=EDGE_CURVE('',#14397,#14398,#11699,.T.);
#17897=EDGE_CURVE('',#14399,#14398,#8031,.T.);
#17898=EDGE_CURVE('',#14399,#14383,#11700,.T.);
#17899=EDGE_CURVE('',#14294,#14400,#8032,.T.);
#17900=EDGE_CURVE('',#14400,#14397,#8033,.T.);
#17901=EDGE_CURVE('',#14293,#14401,#8034,.T.);
#17902=EDGE_CURVE('',#14401,#14400,#1649,.T.);
#17903=EDGE_CURVE('',#14402,#14401,#8035,.T.);
#17904=EDGE_CURVE('',#14292,#14402,#8036,.T.);
#17905=EDGE_CURVE('',#14291,#14403,#8037,.T.);
#17906=EDGE_CURVE('',#14403,#14404,#11701,.T.);
#17907=EDGE_CURVE('',#14405,#14404,#8038,.T.);
#17908=EDGE_CURVE('',#14406,#14405,#1650,.T.);
#17909=EDGE_CURVE('',#14406,#14407,#11702,.T.);
#17910=EDGE_CURVE('',#14408,#14407,#1651,.T.);
#17911=EDGE_CURVE('',#14408,#14409,#8039,.T.);
#17912=EDGE_CURVE('',#14409,#14402,#11703,.T.);
#17913=EDGE_CURVE('',#14290,#14410,#8040,.T.);
#17914=EDGE_CURVE('',#14403,#14410,#8041,.T.);
#17915=EDGE_CURVE('',#14410,#14411,#1652,.T.);
#17916=EDGE_CURVE('',#14289,#14411,#8042,.T.);
#17917=EDGE_CURVE('',#14366,#14411,#8043,.T.);
#17918=EDGE_CURVE('',#14305,#14412,#8044,.T.);
#17919=EDGE_CURVE('',#14309,#14413,#8045,.T.);
#17920=EDGE_CURVE('',#14413,#14414,#11704,.T.);
#17921=EDGE_CURVE('',#14414,#14415,#11705,.T.);
#17922=EDGE_CURVE('',#14415,#14412,#11706,.T.);
#17923=EDGE_CURVE('',#14308,#14416,#8046,.T.);
#17924=EDGE_CURVE('',#14417,#14416,#8047,.T.);
#17925=EDGE_CURVE('',#14413,#14417,#8048,.T.);
#17926=EDGE_CURVE('',#14307,#14418,#8049,.T.);
#17927=EDGE_CURVE('',#14419,#14418,#11707,.T.);
#17928=EDGE_CURVE('',#14420,#14419,#11708,.T.);
#17929=EDGE_CURVE('',#14421,#14420,#11709,.T.);
#17930=EDGE_CURVE('',#14416,#14421,#11710,.T.);
#17931=EDGE_CURVE('',#14306,#14422,#8050,.T.);
#17932=EDGE_CURVE('',#14422,#14418,#11711,.T.);
#17933=EDGE_CURVE('',#14423,#14424,#11712,.T.);
#17934=EDGE_CURVE('',#14425,#14423,#11713,.T.);
#17935=EDGE_CURVE('',#14426,#14425,#11714,.T.);
#17936=EDGE_CURVE('',#14422,#14426,#11715,.T.);
#17937=EDGE_CURVE('',#14304,#14424,#8051,.T.);
#17938=EDGE_CURVE('',#14427,#14412,#8052,.T.);
#17939=EDGE_CURVE('',#14424,#14427,#8053,.T.);
#17940=EDGE_CURVE('',#14316,#14428,#8054,.T.);
#17941=EDGE_CURVE('',#14428,#14429,#8055,.T.);
#17942=EDGE_CURVE('',#14429,#14430,#8056,.T.);
#17943=EDGE_CURVE('',#14430,#14311,#8057,.T.);
#17944=EDGE_CURVE('',#14315,#14431,#8058,.T.);
#17945=EDGE_CURVE('',#14432,#14431,#8059,.T.);
#17946=EDGE_CURVE('',#14428,#14432,#8060,.T.);
#17947=EDGE_CURVE('',#14314,#14433,#8061,.T.);
#17948=EDGE_CURVE('',#14433,#14431,#11716,.T.);
#17949=EDGE_CURVE('',#14313,#14434,#8062,.T.);
#17950=EDGE_CURVE('',#14434,#14435,#8063,.T.);
#17951=EDGE_CURVE('',#14435,#14433,#8064,.T.);
#17952=EDGE_CURVE('',#14312,#14436,#8065,.T.);
#17953=EDGE_CURVE('',#14434,#14436,#8066,.T.);
#17954=EDGE_CURVE('',#14437,#14310,#8067,.T.);
#17955=EDGE_CURVE('',#14438,#14437,#11717,.T.);
#17956=EDGE_CURVE('',#14436,#14438,#11718,.T.);
#17957=EDGE_CURVE('',#14437,#14430,#11719,.T.);
#17958=EDGE_CURVE('',#14320,#14439,#8068,.T.);
#17959=EDGE_CURVE('',#14439,#14351,#11720,.T.);
#17960=EDGE_CURVE('',#14439,#14348,#11721,.T.);
#17961=EDGE_CURVE('',#14319,#14349,#8069,.T.);
#17962=EDGE_CURVE('',#14318,#14350,#8070,.T.);
#17963=EDGE_CURVE('',#14440,#14328,#8071,.T.);
#17964=EDGE_CURVE('',#14440,#14441,#11722,.T.);
#17965=EDGE_CURVE('',#14441,#14322,#8072,.T.);
#17966=EDGE_CURVE('',#14327,#14442,#8073,.T.);
#17967=EDGE_CURVE('',#14442,#14440,#8074,.T.);
#17968=EDGE_CURVE('',#14326,#14443,#8075,.T.);
#17969=EDGE_CURVE('',#14443,#14444,#11723,.T.);
#17970=EDGE_CURVE('',#14444,#14442,#11724,.T.);
#17971=EDGE_CURVE('',#14325,#14445,#8076,.T.);
#17972=EDGE_CURVE('',#14445,#14446,#8077,.T.);
#17973=EDGE_CURVE('',#14446,#14443,#8078,.T.);
#17974=EDGE_CURVE('',#14324,#14447,#8079,.T.);
#17975=EDGE_CURVE('',#14447,#14445,#8080,.T.);
#17976=EDGE_CURVE('',#14448,#14447,#11725,.T.);
#17977=EDGE_CURVE('',#14448,#14323,#8081,.T.);
#17978=EDGE_CURVE('',#14449,#14449,#11726,.T.);
#17979=EDGE_CURVE('',#14449,#14450,#8082,.T.);
#17980=EDGE_CURVE('',#14450,#14448,#11727,.T.);
#17981=EDGE_CURVE('',#14441,#14451,#11728,.T.);
#17982=EDGE_CURVE('',#14451,#14452,#11729,.T.);
#17983=EDGE_CURVE('',#14452,#14450,#11730,.T.);
#17984=EDGE_CURVE('',#14329,#14453,#8083,.T.);
#17985=EDGE_CURVE('',#14279,#14453,#11731,.T.);
#17986=EDGE_CURVE('',#14336,#14454,#8084,.T.);
#17987=EDGE_CURVE('',#14280,#14454,#8085,.T.);
#17988=EDGE_CURVE('',#14455,#14454,#11732,.T.);
#17989=EDGE_CURVE('',#14335,#14455,#8086,.T.);
#17990=EDGE_CURVE('',#14455,#14456,#11733,.T.);
#17991=EDGE_CURVE('',#14334,#14456,#8087,.T.);
#17992=EDGE_CURVE('',#14457,#14456,#11734,.T.);
#17993=EDGE_CURVE('',#14333,#14457,#8088,.T.);
#17994=EDGE_CURVE('',#14458,#14457,#11735,.T.);
#17995=EDGE_CURVE('',#14332,#14458,#8089,.T.);
#17996=EDGE_CURVE('',#14331,#14459,#8090,.T.);
#17997=EDGE_CURVE('',#14459,#14458,#11736,.T.);
#17998=EDGE_CURVE('',#14460,#14459,#11737,.T.);
#17999=EDGE_CURVE('',#14330,#14460,#8091,.T.);
#18000=EDGE_CURVE('',#14453,#14460,#8092,.T.);
#18001=EDGE_CURVE('',#14343,#14461,#8093,.T.);
#18002=EDGE_CURVE('',#14462,#14461,#11738,.T.);
#18003=EDGE_CURVE('',#14462,#14337,#8094,.T.);
#18004=EDGE_CURVE('',#14461,#14463,#8095,.T.);
#18005=EDGE_CURVE('',#14342,#14463,#8096,.T.);
#18006=EDGE_CURVE('',#14341,#14464,#8097,.T.);
#18007=EDGE_CURVE('',#14465,#14464,#8098,.T.);
#18008=EDGE_CURVE('',#14463,#14465,#8099,.T.);
#18009=EDGE_CURVE('',#14340,#14466,#8100,.T.);
#18010=EDGE_CURVE('',#14466,#14467,#11739,.T.);
#18011=EDGE_CURVE('',#14467,#14464,#11740,.T.);
#18012=EDGE_CURVE('',#14339,#14468,#8101,.T.);
#18013=EDGE_CURVE('',#14466,#14468,#8102,.T.);
#18014=EDGE_CURVE('',#14468,#14469,#11741,.T.);
#18015=EDGE_CURVE('',#14469,#14338,#8103,.T.);
#18016=EDGE_CURVE('',#14470,#14471,#11742,.T.);
#18017=EDGE_CURVE('',#14472,#14470,#11743,.T.);
#18018=EDGE_CURVE('',#14469,#14472,#11744,.T.);
#18019=EDGE_CURVE('',#14471,#14462,#11745,.T.);
#18020=EDGE_CURVE('',#14471,#14473,#8104,.T.);
#18021=EDGE_CURVE('',#14474,#14473,#11746,.T.);
#18022=EDGE_CURVE('',#14473,#14474,#11747,.T.);
#18023=EDGE_CURVE('',#14379,#14368,#8105,.T.);
#18024=EDGE_CURVE('',#14378,#14475,#8106,.T.);
#18025=EDGE_CURVE('',#14475,#14369,#8107,.T.);
#18026=EDGE_CURVE('',#14476,#14477,#8108,.T.);
#18027=EDGE_CURVE('',#14476,#14478,#8109,.T.);
#18028=EDGE_CURVE('',#14479,#14478,#8110,.T.);
#18029=EDGE_CURVE('',#14357,#14479,#8111,.T.);
#18030=EDGE_CURVE('',#14480,#14356,#8112,.T.);
#18031=EDGE_CURVE('',#14481,#14480,#8113,.T.);
#18032=EDGE_CURVE('',#14477,#14481,#8114,.T.);
#18033=EDGE_CURVE('',#14482,#14479,#11748,.T.);
#18034=EDGE_CURVE('',#14358,#14482,#8115,.T.);
#18035=EDGE_CURVE('',#14483,#14484,#8116,.T.);
#18036=EDGE_CURVE('',#14484,#14485,#8117,.T.);
#18037=EDGE_CURVE('',#14485,#14359,#8118,.T.);
#18038=EDGE_CURVE('',#14482,#14486,#8119,.T.);
#18039=EDGE_CURVE('',#14487,#14486,#8120,.T.);
#18040=EDGE_CURVE('',#14487,#14483,#8121,.T.);
#18041=EDGE_CURVE('',#14488,#14405,#8122,.T.);
#18042=EDGE_CURVE('',#14365,#14404,#8123,.T.);
#18043=EDGE_CURVE('',#14488,#14364,#8124,.T.);
#18044=EDGE_CURVE('',#14374,#14396,#8125,.T.);
#18045=EDGE_CURVE('',#14489,#14395,#8126,.T.);
#18046=EDGE_CURVE('',#14375,#14489,#8127,.T.);
#18047=EDGE_CURVE('',#14398,#14409,#8128,.T.);
#18048=EDGE_CURVE('',#14490,#14399,#8129,.T.);
#18049=EDGE_CURVE('',#14490,#14408,#8130,.T.);
#18050=EDGE_CURVE('',#14387,#14491,#8131,.T.);
#18051=EDGE_CURVE('',#14492,#14491,#8132,.T.);
#18052=EDGE_CURVE('',#14492,#14493,#8133,.T.);
#18053=EDGE_CURVE('',#14494,#14493,#8134,.T.);
#18054=EDGE_CURVE('',#14494,#14495,#8135,.T.);
#18055=EDGE_CURVE('',#14496,#14495,#8136,.T.);
#18056=EDGE_CURVE('',#14388,#14496,#8137,.T.);
#18057=EDGE_CURVE('',#14496,#14497,#11749,.T.);
#18058=EDGE_CURVE('',#14389,#14497,#8138,.T.);
#18059=EDGE_CURVE('',#14497,#14498,#8139,.T.);
#18060=EDGE_CURVE('',#14499,#14498,#8140,.T.);
#18061=EDGE_CURVE('',#14499,#14500,#8141,.T.);
#18062=EDGE_CURVE('',#14501,#14500,#8142,.T.);
#18063=EDGE_CURVE('',#14501,#14502,#8143,.T.);
#18064=EDGE_CURVE('',#14390,#14502,#8144,.T.);
#18065=EDGE_CURVE('',#14503,#14407,#8145,.T.);
#18066=EDGE_CURVE('',#14504,#14406,#8146,.T.);
#18067=EDGE_CURVE('',#14504,#14503,#11750,.T.);
#18068=EDGE_CURVE('',#14503,#14490,#1653,.T.);
#18069=EDGE_CURVE('',#14504,#14488,#1654,.T.);
#18070=EDGE_CURVE('',#14505,#14415,#8147,.T.);
#18071=EDGE_CURVE('',#14505,#14427,#1655,.T.);
#18072=EDGE_CURVE('',#14506,#14421,#1656,.T.);
#18073=EDGE_CURVE('',#14506,#14507,#589,.T.);
#18074=EDGE_CURVE('',#14507,#14423,#1657,.T.);
#18075=EDGE_CURVE('',#14508,#14414,#8148,.T.);
#18076=EDGE_CURVE('',#14417,#14508,#1658,.T.);
#18077=EDGE_CURVE('',#14420,#14509,#1659,.T.);
#18078=EDGE_CURVE('',#14419,#14509,#8149,.T.);
#18079=EDGE_CURVE('',#14426,#14510,#8150,.T.);
#18080=EDGE_CURVE('',#14510,#14425,#1660,.T.);
#18081=EDGE_CURVE('',#14438,#14511,#1661,.T.);
#18082=EDGE_CURVE('',#14429,#14511,#590,.T.);
#18083=EDGE_CURVE('',#14435,#14432,#591,.T.);
#18084=EDGE_CURVE('',#14444,#14512,#8151,.T.);
#18085=EDGE_CURVE('',#14451,#14512,#592,.T.);
#18086=EDGE_CURVE('',#14446,#14452,#593,.T.);
#18087=EDGE_CURVE('',#14449,#14513,#11751,.T.);
#18088=EDGE_CURVE('',#14513,#14513,#11752,.T.);
#18089=EDGE_CURVE('',#14514,#14515,#11753,.T.);
#18090=EDGE_CURVE('',#14516,#14514,#11754,.T.);
#18091=EDGE_CURVE('',#14517,#14516,#11755,.T.);
#18092=EDGE_CURVE('',#14517,#14518,#11756,.T.);
#18093=EDGE_CURVE('',#14519,#14518,#11757,.T.);
#18094=EDGE_CURVE('',#14520,#14519,#8152,.T.);
#18095=EDGE_CURVE('',#14521,#14520,#11758,.T.);
#18096=EDGE_CURVE('',#14521,#14522,#11759,.T.);
#18097=EDGE_CURVE('',#14522,#14515,#8153,.T.);
#18098=EDGE_CURVE('',#14523,#14523,#11760,.T.);
#18099=EDGE_CURVE('',#14524,#14524,#11761,.T.);
#18100=EDGE_CURVE('',#14470,#14465,#594,.T.);
#18101=EDGE_CURVE('',#14467,#14525,#8154,.T.);
#18102=EDGE_CURVE('',#14525,#14472,#595,.T.);
#18103=EDGE_CURVE('',#14474,#14526,#11762,.T.);
#18104=EDGE_CURVE('',#14526,#14526,#11763,.T.);
#18105=EDGE_CURVE('',#14377,#14527,#8155,.T.);
#18106=EDGE_CURVE('',#14527,#14475,#1662,.T.);
#18107=EDGE_CURVE('',#14528,#14527,#11764,.T.);
#18108=EDGE_CURVE('',#14489,#14528,#1663,.T.);
#18109=EDGE_CURVE('',#14395,#14369,#11765,.T.);
#18110=EDGE_CURVE('',#14529,#14530,#8156,.T.);
#18111=EDGE_CURVE('',#14529,#14481,#11766,.T.);
#18112=EDGE_CURVE('',#14480,#14530,#11767,.T.);
#18113=EDGE_CURVE('',#14531,#14532,#11768,.T.);
#18114=EDGE_CURVE('',#14533,#14532,#8157,.T.);
#18115=EDGE_CURVE('',#14533,#14534,#11769,.T.);
#18116=EDGE_CURVE('',#14534,#14531,#8158,.T.);
#18117=EDGE_CURVE('',#14535,#14536,#8159,.T.);
#18118=EDGE_CURVE('',#14536,#14537,#11770,.T.);
#18119=EDGE_CURVE('',#14538,#14537,#8160,.T.);
#18120=EDGE_CURVE('',#14538,#14535,#11771,.T.);
#18121=EDGE_CURVE('',#14539,#14540,#8161,.T.);
#18122=EDGE_CURVE('',#14539,#14541,#11772,.T.);
#18123=EDGE_CURVE('',#14541,#14542,#8162,.T.);
#18124=EDGE_CURVE('',#14542,#14540,#11773,.T.);
#18125=EDGE_CURVE('',#14543,#14544,#11774,.T.);
#18126=EDGE_CURVE('',#14545,#14544,#8163,.T.);
#18127=EDGE_CURVE('',#14546,#14545,#11775,.T.);
#18128=EDGE_CURVE('',#14546,#14543,#8164,.T.);
#18129=EDGE_CURVE('',#14547,#14548,#8165,.T.);
#18130=EDGE_CURVE('',#14548,#14502,#11776,.T.);
#18131=EDGE_CURVE('',#14501,#14547,#11777,.T.);
#18132=EDGE_CURVE('',#14476,#14487,#8166,.T.);
#18133=EDGE_CURVE('',#14477,#14483,#8167,.T.);
#18134=EDGE_CURVE('',#14486,#14478,#11778,.T.);
#18135=EDGE_CURVE('',#14549,#14550,#8168,.T.);
#18136=EDGE_CURVE('',#14551,#14550,#1664,.T.);
#18137=EDGE_CURVE('',#14552,#14551,#11779,.T.);
#18138=EDGE_CURVE('',#14552,#14553,#8169,.T.);
#18139=EDGE_CURVE('',#14549,#14553,#11780,.T.);
#18140=EDGE_CURVE('',#14554,#14555,#11781,.T.);
#18141=EDGE_CURVE('',#14554,#14556,#11782,.T.);
#18142=EDGE_CURVE('',#14556,#14557,#8170,.T.);
#18143=EDGE_CURVE('',#14558,#14557,#1665,.T.);
#18144=EDGE_CURVE('',#14559,#14558,#8171,.T.);
#18145=EDGE_CURVE('',#14559,#14555,#11783,.T.);
#18146=EDGE_CURVE('',#14560,#14561,#8172,.T.);
#18147=EDGE_CURVE('',#14484,#14560,#11784,.T.);
#18148=EDGE_CURVE('',#14562,#14529,#8173,.T.);
#18149=EDGE_CURVE('',#14563,#14562,#11785,.T.);
#18150=EDGE_CURVE('',#14563,#14564,#8174,.T.);
#18151=EDGE_CURVE('',#14565,#14564,#11786,.T.);
#18152=EDGE_CURVE('',#14565,#14566,#8175,.T.);
#18153=EDGE_CURVE('',#14566,#14532,#11787,.T.);
#18154=EDGE_CURVE('',#14531,#14567,#11788,.T.);
#18155=EDGE_CURVE('',#14568,#14567,#8176,.T.);
#18156=EDGE_CURVE('',#14569,#14568,#11789,.T.);
#18157=EDGE_CURVE('',#14569,#14570,#8177,.T.);
#18158=EDGE_CURVE('',#14571,#14570,#11790,.T.);
#18159=EDGE_CURVE('',#14571,#14535,#8178,.T.);
#18160=EDGE_CURVE('',#14538,#14572,#8179,.T.);
#18161=EDGE_CURVE('',#14572,#14573,#11791,.T.);
#18162=EDGE_CURVE('',#14573,#14574,#11792,.T.);
#18163=EDGE_CURVE('',#14575,#14574,#1666,.T.);
#18164=EDGE_CURVE('',#14575,#14576,#1667,.T.);
#18165=EDGE_CURVE('',#14561,#14576,#1668,.T.);
#18166=EDGE_CURVE('',#14560,#14577,#8180,.T.);
#18167=EDGE_CURVE('',#14577,#14485,#11793,.T.);
#18168=EDGE_CURVE('',#14578,#14555,#8181,.T.);
#18169=EDGE_CURVE('',#14578,#14579,#11794,.T.);
#18170=EDGE_CURVE('',#14579,#14554,#8182,.T.);
#18171=EDGE_CURVE('',#14549,#14580,#8183,.T.);
#18172=EDGE_CURVE('',#14553,#14581,#8184,.T.);
#18173=EDGE_CURVE('',#14581,#14580,#11795,.T.);
#18174=EDGE_CURVE('',#14582,#14583,#8185,.T.);
#18175=EDGE_CURVE('',#14583,#14584,#11796,.T.);
#18176=EDGE_CURVE('',#14585,#14584,#8186,.T.);
#18177=EDGE_CURVE('',#14585,#14582,#11797,.T.);
#18178=EDGE_CURVE('',#14586,#14587,#11798,.T.);
#18179=EDGE_CURVE('',#14588,#14587,#8187,.T.);
#18180=EDGE_CURVE('',#14589,#14588,#11799,.T.);
#18181=EDGE_CURVE('',#14589,#14586,#8188,.T.);
#18182=EDGE_CURVE('',#14590,#14591,#8189,.T.);
#18183=EDGE_CURVE('',#14590,#14492,#11800,.T.);
#18184=EDGE_CURVE('',#14491,#14591,#11801,.T.);
#18185=EDGE_CURVE('',#14364,#14399,#11802,.T.);
#18186=EDGE_CURVE('',#14376,#14528,#8190,.T.);
#18187=EDGE_CURVE('',#14495,#14498,#11803,.T.);
#18188=EDGE_CURVE('',#14499,#14494,#8191,.T.);
#18189=EDGE_CURVE('',#14500,#14493,#8192,.T.);
#18190=EDGE_CURVE('',#14592,#14585,#8193,.T.);
#18191=EDGE_CURVE('',#14593,#14592,#11804,.T.);
#18192=EDGE_CURVE('',#14593,#14594,#1669,.T.);
#18193=EDGE_CURVE('',#14582,#14594,#8194,.T.);
#18194=EDGE_CURVE('',#14595,#14596,#8195,.T.);
#18195=EDGE_CURVE('',#14595,#14587,#11805,.T.);
#18196=EDGE_CURVE('',#14586,#14597,#11806,.T.);
#18197=EDGE_CURVE('',#14597,#14598,#8196,.T.);
#18198=EDGE_CURVE('',#14598,#14596,#1670,.T.);
#18199=EDGE_CURVE('',#14543,#14599,#11807,.T.);
#18200=EDGE_CURVE('',#14600,#14599,#8197,.T.);
#18201=EDGE_CURVE('',#14601,#14600,#11808,.T.);
#18202=EDGE_CURVE('',#14602,#14601,#8198,.T.);
#18203=EDGE_CURVE('',#14603,#14602,#11809,.T.);
#18204=EDGE_CURVE('',#14603,#14547,#8199,.T.);
#18205=EDGE_CURVE('',#14590,#14604,#8200,.T.);
#18206=EDGE_CURVE('',#14604,#14605,#1671,.T.);
#18207=EDGE_CURVE('',#14606,#14605,#1672,.T.);
#18208=EDGE_CURVE('',#14606,#14607,#1673,.T.);
#18209=EDGE_CURVE('',#14608,#14607,#11810,.T.);
#18210=EDGE_CURVE('',#14609,#14608,#11811,.T.);
#18211=EDGE_CURVE('',#14541,#14609,#8201,.T.);
#18212=EDGE_CURVE('',#14610,#14539,#8202,.T.);
#18213=EDGE_CURVE('',#14611,#14610,#11812,.T.);
#18214=EDGE_CURVE('',#14612,#14611,#8203,.T.);
#18215=EDGE_CURVE('',#14613,#14612,#11813,.T.);
#18216=EDGE_CURVE('',#14613,#14614,#8204,.T.);
#18217=EDGE_CURVE('',#14614,#14544,#11814,.T.);
#18218=EDGE_CURVE('',#14615,#14615,#11815,.T.);
#18219=EDGE_CURVE('',#14616,#14515,#8205,.T.);
#18220=EDGE_CURVE('',#14616,#14617,#11816,.T.);
#18221=EDGE_CURVE('',#14617,#14514,#8206,.T.);
#18222=EDGE_CURVE('',#14617,#14618,#11817,.T.);
#18223=EDGE_CURVE('',#14618,#14516,#8207,.T.);
#18224=EDGE_CURVE('',#14618,#14619,#11818,.T.);
#18225=EDGE_CURVE('',#14619,#14517,#8208,.T.);
#18226=EDGE_CURVE('',#14620,#14518,#8209,.T.);
#18227=EDGE_CURVE('',#14620,#14619,#11819,.T.);
#18228=EDGE_CURVE('',#14620,#14621,#11820,.T.);
#18229=EDGE_CURVE('',#14621,#14519,#8210,.T.);
#18230=EDGE_CURVE('',#14622,#14621,#8211,.T.);
#18231=EDGE_CURVE('',#14622,#14520,#8212,.T.);
#18232=EDGE_CURVE('',#14623,#14622,#11821,.T.);
#18233=EDGE_CURVE('',#14623,#14521,#8213,.T.);
#18234=EDGE_CURVE('',#14623,#14624,#11822,.T.);
#18235=EDGE_CURVE('',#14624,#14522,#8214,.T.);
#18236=EDGE_CURVE('',#14624,#14616,#8215,.T.);
#18237=EDGE_CURVE('',#14523,#14625,#8216,.T.);
#18238=EDGE_CURVE('',#14625,#14625,#11823,.T.);
#18239=EDGE_CURVE('',#14626,#14626,#11824,.T.);
#18240=EDGE_CURVE('',#14626,#14524,#8217,.T.);
#18241=EDGE_CURVE('',#14627,#14627,#11825,.T.);
#18242=EDGE_CURVE('',#14628,#14629,#11826,.T.);
#18243=EDGE_CURVE('',#14573,#14629,#8218,.T.);
#18244=EDGE_CURVE('',#14572,#14628,#8219,.T.);
#18245=EDGE_CURVE('',#14630,#14629,#11827,.T.);
#18246=EDGE_CURVE('',#14574,#14630,#8220,.T.);
#18247=EDGE_CURVE('',#14575,#14631,#8221,.T.);
#18248=EDGE_CURVE('',#14631,#14630,#1674,.T.);
#18249=EDGE_CURVE('',#14631,#14632,#1675,.T.);
#18250=EDGE_CURVE('',#14576,#14632,#8222,.T.);
#18251=EDGE_CURVE('',#14633,#14632,#1676,.T.);
#18252=EDGE_CURVE('',#14561,#14633,#8223,.T.);
#18253=EDGE_CURVE('',#14557,#14634,#8224,.T.);
#18254=EDGE_CURVE('',#14635,#14634,#1677,.T.);
#18255=EDGE_CURVE('',#14558,#14635,#8225,.T.);
#18256=EDGE_CURVE('',#14636,#14637,#1678,.T.);
#18257=EDGE_CURVE('',#14551,#14636,#8226,.T.);
#18258=EDGE_CURVE('',#14550,#14637,#8227,.T.);
#18259=EDGE_CURVE('',#14636,#14638,#11828,.T.);
#18260=EDGE_CURVE('',#14552,#14638,#8228,.T.);
#18261=EDGE_CURVE('',#14639,#14640,#11829,.T.);
#18262=EDGE_CURVE('',#14593,#14640,#8229,.T.);
#18263=EDGE_CURVE('',#14592,#14639,#8230,.T.);
#18264=EDGE_CURVE('',#14594,#14641,#8231,.T.);
#18265=EDGE_CURVE('',#14640,#14641,#1679,.T.);
#18266=EDGE_CURVE('',#14596,#14642,#8232,.T.);
#18267=EDGE_CURVE('',#14598,#14643,#8233,.T.);
#18268=EDGE_CURVE('',#14643,#14642,#1680,.T.);
#18269=EDGE_CURVE('',#14604,#14644,#8234,.T.);
#18270=EDGE_CURVE('',#14644,#14645,#1681,.T.);
#18271=EDGE_CURVE('',#14605,#14645,#8235,.T.);
#18272=EDGE_CURVE('',#14606,#14646,#8236,.T.);
#18273=EDGE_CURVE('',#14646,#14645,#1682,.T.);
#18274=EDGE_CURVE('',#14646,#14647,#1683,.T.);
#18275=EDGE_CURVE('',#14647,#14607,#8237,.T.);
#18276=EDGE_CURVE('',#14648,#14647,#11830,.T.);
#18277=EDGE_CURVE('',#14648,#14608,#8238,.T.);
#18278=EDGE_CURVE('',#14649,#14648,#11831,.T.);
#18279=EDGE_CURVE('',#14609,#14649,#8239,.T.);
#18280=EDGE_CURVE('',#14650,#14650,#11832,.T.);
#18281=EDGE_CURVE('',#14650,#14615,#8240,.T.);
#18282=EDGE_CURVE('',#14651,#14275,#11833,.T.);
#18283=EDGE_CURVE('',#14652,#14274,#8241,.T.);
#18284=EDGE_CURVE('',#14653,#14652,#11834,.T.);
#18285=EDGE_CURVE('',#14653,#14654,#11835,.T.);
#18286=EDGE_CURVE('',#14654,#14651,#8242,.T.);
#18287=EDGE_CURVE('',#14655,#14655,#11836,.T.);
#18288=EDGE_CURVE('',#14656,#14656,#11837,.T.);
#18289=EDGE_CURVE('',#14627,#14657,#8243,.T.);
#18290=EDGE_CURVE('',#14657,#14657,#11838,.T.);
#18291=EDGE_CURVE('',#14651,#14658,#8244,.T.);
#18292=EDGE_CURVE('',#14658,#14659,#11839,.T.);
#18293=EDGE_CURVE('',#14659,#14276,#11840,.T.);
#18294=EDGE_CURVE('',#14660,#14278,#8245,.T.);
#18295=EDGE_CURVE('',#14661,#14660,#1684,.T.);
#18296=EDGE_CURVE('',#14662,#14661,#8246,.T.);
#18297=EDGE_CURVE('',#14652,#14662,#8247,.T.);
#18298=EDGE_CURVE('',#14663,#14662,#11841,.T.);
#18299=EDGE_CURVE('',#14664,#14663,#11842,.T.);
#18300=EDGE_CURVE('',#14653,#14664,#8248,.T.);
#18301=EDGE_CURVE('',#14664,#14665,#11843,.T.);
#18302=EDGE_CURVE('',#14665,#14666,#11844,.T.);
#18303=EDGE_CURVE('',#14654,#14666,#8249,.T.);
#18304=EDGE_CURVE('',#14666,#14667,#8250,.T.);
#18305=EDGE_CURVE('',#14667,#14668,#8251,.T.);
#18306=EDGE_CURVE('',#14668,#14658,#8252,.T.);
#18307=EDGE_CURVE('',#14655,#14669,#8253,.T.);
#18308=EDGE_CURVE('',#14670,#14669,#11845,.T.);
#18309=EDGE_CURVE('',#14671,#14670,#11846,.T.);
#18310=EDGE_CURVE('',#14672,#14671,#11847,.T.);
#18311=EDGE_CURVE('',#14673,#14672,#11848,.T.);
#18312=EDGE_CURVE('',#14674,#14673,#11849,.T.);
#18313=EDGE_CURVE('',#14675,#14674,#11850,.T.);
#18314=EDGE_CURVE('',#14669,#14675,#11851,.T.);
#18315=EDGE_CURVE('',#14676,#14677,#11852,.T.);
#18316=EDGE_CURVE('',#14677,#14656,#8254,.T.);
#18317=EDGE_CURVE('',#14677,#14678,#11853,.T.);
#18318=EDGE_CURVE('',#14678,#14679,#11854,.T.);
#18319=EDGE_CURVE('',#14679,#14680,#11855,.T.);
#18320=EDGE_CURVE('',#14680,#14681,#11856,.T.);
#18321=EDGE_CURVE('',#14681,#14682,#11857,.T.);
#18322=EDGE_CURVE('',#14682,#14676,#11858,.T.);
#18323=EDGE_CURVE('',#14683,#14684,#11859,.T.);
#18324=EDGE_CURVE('',#14685,#14683,#8255,.T.);
#18325=EDGE_CURVE('',#14685,#14686,#11860,.T.);
#18326=EDGE_CURVE('',#14684,#14686,#8256,.T.);
#18327=EDGE_CURVE('',#14687,#14688,#8257,.T.);
#18328=EDGE_CURVE('',#14687,#14684,#11861,.T.);
#18329=EDGE_CURVE('',#14688,#14686,#11862,.T.);
#18330=EDGE_CURVE('',#14689,#14688,#1685,.T.);
#18331=EDGE_CURVE('',#14689,#14690,#8258,.T.);
#18332=EDGE_CURVE('',#14690,#14687,#1686,.T.);
#18333=EDGE_CURVE('',#14691,#14692,#8259,.T.);
#18334=EDGE_CURVE('',#14690,#14692,#1687,.T.);
#18335=EDGE_CURVE('',#14689,#14691,#1688,.T.);
#18336=EDGE_CURVE('',#14693,#14692,#1689,.T.);
#18337=EDGE_CURVE('',#14694,#14691,#1690,.T.);
#18338=EDGE_CURVE('',#14693,#14694,#8260,.T.);
#18339=EDGE_CURVE('',#14693,#14695,#11863,.T.);
#18340=EDGE_CURVE('',#14694,#14696,#11864,.T.);
#18341=EDGE_CURVE('',#14695,#14696,#8261,.T.);
#18342=EDGE_CURVE('',#14697,#14698,#8262,.T.);
#18343=EDGE_CURVE('',#14695,#14698,#1691,.T.);
#18344=EDGE_CURVE('',#14696,#14697,#1692,.T.);
#18345=EDGE_CURVE('',#14699,#14698,#1693,.T.);
#18346=EDGE_CURVE('',#14700,#14697,#1694,.T.);
#18347=EDGE_CURVE('',#14700,#14699,#8263,.T.);
#18348=EDGE_CURVE('',#14701,#14702,#8264,.T.);
#18349=EDGE_CURVE('',#14699,#14702,#1695,.T.);
#18350=EDGE_CURVE('',#14700,#14701,#1696,.T.);
#18351=EDGE_CURVE('',#14703,#14704,#8265,.T.);
#18352=EDGE_CURVE('',#14704,#14702,#11865,.T.);
#18353=EDGE_CURVE('',#14701,#14703,#11866,.T.);
#18354=EDGE_CURVE('',#14683,#14704,#11867,.T.);
#18355=EDGE_CURVE('',#14685,#14703,#11868,.T.);
#18356=EDGE_CURVE('',#14705,#14659,#596,.T.);
#18357=EDGE_CURVE('',#14705,#14277,#597,.T.);
#18358=EDGE_CURVE('',#14706,#14668,#1697,.T.);
#18359=EDGE_CURVE('',#14707,#14706,#11869,.T.);
#18360=EDGE_CURVE('',#14707,#14708,#11870,.T.);
#18361=EDGE_CURVE('',#14708,#14660,#1698,.T.);
#18362=EDGE_CURVE('',#14661,#14663,#1699,.T.);
#18363=EDGE_CURVE('',#14709,#14710,#1700,.T.);
#18364=EDGE_CURVE('',#14710,#14711,#8266,.T.);
#18365=EDGE_CURVE('',#14663,#14711,#1701,.T.);
#18366=EDGE_CURVE('',#14709,#14708,#8267,.T.);
#18367=EDGE_CURVE('',#14712,#14711,#1702,.T.);
#18368=EDGE_CURVE('',#14713,#14712,#11871,.T.);
#18369=EDGE_CURVE('',#14713,#14714,#1703,.T.);
#18370=EDGE_CURVE('',#14665,#14714,#1704,.T.);
#18371=EDGE_CURVE('',#14667,#14665,#1705,.T.);
#18372=EDGE_CURVE('',#14715,#14706,#8268,.T.);
#18373=EDGE_CURVE('',#14716,#14714,#8269,.T.);
#18374=EDGE_CURVE('',#14715,#14716,#1706,.T.);
#18375=EDGE_CURVE('',#14717,#14671,#598,.T.);
#18376=EDGE_CURVE('',#14717,#14718,#11872,.T.);
#18377=EDGE_CURVE('',#14674,#14718,#1707,.T.);
#18378=EDGE_CURVE('',#14673,#14719,#1708,.T.);
#18379=EDGE_CURVE('',#14720,#14719,#599,.T.);
#18380=EDGE_CURVE('',#14720,#14672,#1709,.T.);
#18381=EDGE_CURVE('',#14721,#14674,#1710,.T.);
#18382=EDGE_CURVE('',#14722,#14721,#1711,.T.);
#18383=EDGE_CURVE('',#14723,#14722,#1712,.T.);
#18384=EDGE_CURVE('',#14723,#14724,#1713,.T.);
#18385=EDGE_CURVE('',#14675,#14724,#600,.T.);
#18386=EDGE_CURVE('',#14670,#14675,#1714,.T.);
#18387=EDGE_CURVE('',#14725,#14670,#1715,.T.);
#18388=EDGE_CURVE('',#14725,#14726,#11873,.T.);
#18389=EDGE_CURVE('',#14727,#14726,#8270,.T.);
#18390=EDGE_CURVE('',#14727,#14728,#11874,.T.);
#18391=EDGE_CURVE('',#14671,#14728,#601,.T.);
#18392=EDGE_CURVE('',#14676,#14678,#1716,.T.);
#18393=EDGE_CURVE('',#14682,#14729,#602,.T.);
#18394=EDGE_CURVE('',#14730,#14729,#11875,.T.);
#18395=EDGE_CURVE('',#14730,#14731,#8271,.T.);
#18396=EDGE_CURVE('',#14732,#14731,#11876,.T.);
#18397=EDGE_CURVE('',#14732,#14676,#1717,.T.);
#18398=EDGE_CURVE('',#14679,#14733,#1718,.T.);
#18399=EDGE_CURVE('',#14734,#14733,#11877,.T.);
#18400=EDGE_CURVE('',#14734,#14682,#603,.T.);
#18401=EDGE_CURVE('',#14735,#14681,#1719,.T.);
#18402=EDGE_CURVE('',#14735,#14736,#604,.T.);
#18403=EDGE_CURVE('',#14680,#14736,#1720,.T.);
#18404=EDGE_CURVE('',#14678,#14737,#605,.T.);
#18405=EDGE_CURVE('',#14738,#14737,#1721,.T.);
#18406=EDGE_CURVE('',#14738,#14739,#1722,.T.);
#18407=EDGE_CURVE('',#14739,#14740,#1723,.T.);
#18408=EDGE_CURVE('',#14740,#14679,#1724,.T.);
#18409=EDGE_CURVE('',#14741,#14742,#1725,.T.);
#18410=EDGE_CURVE('',#14742,#14743,#1726,.T.);
#18411=EDGE_CURVE('',#14743,#14744,#11878,.T.);
#18412=EDGE_CURVE('',#14744,#14745,#11879,.T.);
#18413=EDGE_CURVE('',#14745,#14746,#8272,.T.);
#18414=EDGE_CURVE('',#14747,#14746,#11880,.T.);
#18415=EDGE_CURVE('',#14748,#14747,#11881,.T.);
#18416=EDGE_CURVE('',#14748,#14749,#1727,.T.);
#18417=EDGE_CURVE('',#14741,#14749,#1728,.T.);
#18418=EDGE_CURVE('',#14750,#14751,#1729,.T.);
#18419=EDGE_CURVE('',#14752,#14751,#1730,.T.);
#18420=EDGE_CURVE('',#14753,#14752,#11882,.T.);
#18421=EDGE_CURVE('',#14753,#14754,#1731,.T.);
#18422=EDGE_CURVE('',#14755,#14754,#1732,.T.);
#18423=EDGE_CURVE('',#14756,#14755,#11883,.T.);
#18424=EDGE_CURVE('',#14756,#14750,#11884,.T.);
#18425=EDGE_CURVE('',#14757,#14758,#11885,.T.);
#18426=EDGE_CURVE('',#14758,#14759,#11886,.T.);
#18427=EDGE_CURVE('',#14760,#14759,#8273,.T.);
#18428=EDGE_CURVE('',#14761,#14760,#11887,.T.);
#18429=EDGE_CURVE('',#14762,#14761,#11888,.T.);
#18430=EDGE_CURVE('',#14763,#14762,#1733,.T.);
#18431=EDGE_CURVE('',#14764,#14763,#1734,.T.);
#18432=EDGE_CURVE('',#14764,#14765,#1735,.T.);
#18433=EDGE_CURVE('',#14757,#14765,#1736,.T.);
#18434=EDGE_CURVE('',#14766,#14709,#11889,.T.);
#18435=EDGE_CURVE('',#14766,#14707,#8274,.T.);
#18436=EDGE_CURVE('',#14766,#14715,#11890,.T.);
#18437=EDGE_CURVE('',#14767,#14710,#1737,.T.);
#18438=EDGE_CURVE('',#14767,#14712,#8275,.T.);
#18439=EDGE_CURVE('',#14768,#14769,#1738,.T.);
#18440=EDGE_CURVE('',#14770,#14769,#1739,.T.);
#18441=EDGE_CURVE('',#14771,#14770,#11891,.T.);
#18442=EDGE_CURVE('',#14771,#14772,#11892,.T.);
#18443=EDGE_CURVE('',#14772,#14773,#1740,.T.);
#18444=EDGE_CURVE('',#14774,#14773,#1741,.T.);
#18445=EDGE_CURVE('',#14768,#14774,#11893,.T.);
#18446=EDGE_CURVE('',#14775,#14767,#11894,.T.);
#18447=EDGE_CURVE('',#14775,#14716,#1742,.T.);
#18448=EDGE_CURVE('',#14775,#14713,#8276,.T.);
#18449=EDGE_CURVE('',#14776,#14718,#8277,.T.);
#18450=EDGE_CURVE('',#14777,#14776,#1743,.T.);
#18451=EDGE_CURVE('',#14777,#14721,#8278,.T.);
#18452=EDGE_CURVE('',#14778,#14776,#11895,.T.);
#18453=EDGE_CURVE('',#14778,#14717,#8279,.T.);
#18454=EDGE_CURVE('',#14779,#14728,#8280,.T.);
#18455=EDGE_CURVE('',#14778,#14779,#1744,.T.);
#18456=EDGE_CURVE('',#14780,#14722,#8281,.T.);
#18457=EDGE_CURVE('',#14780,#14777,#1745,.T.);
#18458=EDGE_CURVE('',#14781,#14723,#8282,.T.);
#18459=EDGE_CURVE('',#14781,#14780,#1746,.T.);
#18460=EDGE_CURVE('',#14781,#14782,#1747,.T.);
#18461=EDGE_CURVE('',#14782,#14724,#8283,.T.);
#18462=EDGE_CURVE('',#14783,#14782,#1748,.T.);
#18463=EDGE_CURVE('',#14783,#14725,#8284,.T.);
#18464=EDGE_CURVE('',#14783,#14784,#11896,.T.);
#18465=EDGE_CURVE('',#14784,#14726,#8285,.T.);
#18466=EDGE_CURVE('',#14785,#14784,#8286,.T.);
#18467=EDGE_CURVE('',#14785,#14727,#8287,.T.);
#18468=EDGE_CURVE('',#14785,#14779,#11897,.T.);
#18469=EDGE_CURVE('',#14786,#14787,#1749,.T.);
#18470=EDGE_CURVE('',#14787,#14737,#8288,.T.);
#18471=EDGE_CURVE('',#14786,#14732,#8289,.T.);
#18472=EDGE_CURVE('',#14788,#14789,#1750,.T.);
#18473=EDGE_CURVE('',#14789,#14729,#8290,.T.);
#18474=EDGE_CURVE('',#14788,#14734,#8291,.T.);
#18475=EDGE_CURVE('',#14790,#14789,#11898,.T.);
#18476=EDGE_CURVE('',#14790,#14730,#8292,.T.);
#18477=EDGE_CURVE('',#14790,#14791,#8293,.T.);
#18478=EDGE_CURVE('',#14791,#14731,#8294,.T.);
#18479=EDGE_CURVE('',#14786,#14791,#11899,.T.);
#18480=EDGE_CURVE('',#14788,#14792,#11900,.T.);
#18481=EDGE_CURVE('',#14792,#14733,#8295,.T.);
#18482=EDGE_CURVE('',#14793,#14792,#1751,.T.);
#18483=EDGE_CURVE('',#14793,#14740,#8296,.T.);
#18484=EDGE_CURVE('',#14794,#14787,#1752,.T.);
#18485=EDGE_CURVE('',#14794,#14738,#8297,.T.);
#18486=EDGE_CURVE('',#14794,#14795,#1753,.T.);
#18487=EDGE_CURVE('',#14795,#14739,#8298,.T.);
#18488=EDGE_CURVE('',#14795,#14793,#1754,.T.);
#18489=EDGE_CURVE('',#14741,#14796,#8299,.T.);
#18490=EDGE_CURVE('',#14796,#14797,#1755,.T.);
#18491=EDGE_CURVE('',#14742,#14797,#8300,.T.);
#18492=EDGE_CURVE('',#14797,#14798,#1756,.T.);
#18493=EDGE_CURVE('',#14743,#14798,#8301,.T.);
#18494=EDGE_CURVE('',#14798,#14799,#11901,.T.);
#18495=EDGE_CURVE('',#14799,#14744,#8302,.T.);
#18496=EDGE_CURVE('',#14800,#14745,#8303,.T.);
#18497=EDGE_CURVE('',#14799,#14800,#11902,.T.);
#18498=EDGE_CURVE('',#14800,#14801,#8304,.T.);
#18499=EDGE_CURVE('',#14746,#14801,#8305,.T.);
#18500=EDGE_CURVE('',#14802,#14747,#8306,.T.);
#18501=EDGE_CURVE('',#14802,#14801,#11903,.T.);
#18502=EDGE_CURVE('',#14803,#14802,#11904,.T.);
#18503=EDGE_CURVE('',#14803,#14748,#8307,.T.);
#18504=EDGE_CURVE('',#14803,#14804,#1757,.T.);
#18505=EDGE_CURVE('',#14749,#14804,#8308,.T.);
#18506=EDGE_CURVE('',#14796,#14804,#1758,.T.);
#18507=EDGE_CURVE('',#14751,#14769,#8309,.T.);
#18508=EDGE_CURVE('',#14750,#14770,#8310,.T.);
#18509=EDGE_CURVE('',#14752,#14768,#8311,.T.);
#18510=EDGE_CURVE('',#14753,#14774,#8312,.T.);
#18511=EDGE_CURVE('',#14754,#14773,#8313,.T.);
#18512=EDGE_CURVE('',#14755,#14772,#8314,.T.);
#18513=EDGE_CURVE('',#14756,#14771,#8315,.T.);
#18514=EDGE_CURVE('',#14805,#14806,#11905,.T.);
#18515=EDGE_CURVE('',#14758,#14805,#8316,.T.);
#18516=EDGE_CURVE('',#14757,#14806,#8317,.T.);
#18517=EDGE_CURVE('',#14805,#14807,#11906,.T.);
#18518=EDGE_CURVE('',#14759,#14807,#8318,.T.);
#18519=EDGE_CURVE('',#14808,#14807,#8319,.T.);
#18520=EDGE_CURVE('',#14760,#14808,#8320,.T.);
#18521=EDGE_CURVE('',#14808,#14809,#11907,.T.);
#18522=EDGE_CURVE('',#14761,#14809,#8321,.T.);
#18523=EDGE_CURVE('',#14810,#14809,#11908,.T.);
#18524=EDGE_CURVE('',#14762,#14810,#8322,.T.);
#18525=EDGE_CURVE('',#14811,#14810,#1759,.T.);
#18526=EDGE_CURVE('',#14763,#14811,#8323,.T.);
#18527=EDGE_CURVE('',#14812,#14811,#1760,.T.);
#18528=EDGE_CURVE('',#14764,#14812,#8324,.T.);
#18529=EDGE_CURVE('',#14812,#14813,#1761,.T.);
#18530=EDGE_CURVE('',#14765,#14813,#8325,.T.);
#18531=EDGE_CURVE('',#14806,#14813,#1762,.T.);
#18532=EDGE_CURVE('',#14649,#14542,#8326,.T.);
#18533=EDGE_CURVE('',#14628,#14537,#8327,.T.);
#18534=EDGE_CURVE('',#14584,#14639,#8328,.T.);
#18535=EDGE_CURVE('',#14581,#14638,#8329,.T.);
#18536=EDGE_CURVE('',#14814,#14556,#8330,.T.);
#18537=EDGE_CURVE('',#14814,#14815,#8331,.T.);
#18538=EDGE_CURVE('',#14816,#14815,#8332,.T.);
#18539=EDGE_CURVE('',#14816,#14634,#8333,.T.);
#18540=EDGE_CURVE('',#14817,#14633,#8334,.T.);
#18541=EDGE_CURVE('',#14817,#14818,#8335,.T.);
#18542=EDGE_CURVE('',#14818,#14819,#8336,.T.);
#18543=EDGE_CURVE('',#14820,#14819,#8337,.T.);
#18544=EDGE_CURVE('',#14577,#14820,#8338,.T.);
#18545=EDGE_CURVE('',#14580,#14821,#8339,.T.);
#18546=EDGE_CURVE('',#14821,#14822,#8340,.T.);
#18547=EDGE_CURVE('',#14822,#14823,#8341,.T.);
#18548=EDGE_CURVE('',#14824,#14823,#8342,.T.);
#18549=EDGE_CURVE('',#14824,#14637,#8343,.T.);
#18550=EDGE_CURVE('',#14825,#14635,#8344,.T.);
#18551=EDGE_CURVE('',#14825,#14826,#8345,.T.);
#18552=EDGE_CURVE('',#14826,#14827,#8346,.T.);
#18553=EDGE_CURVE('',#14827,#14559,#8347,.T.);
#18554=EDGE_CURVE('',#14828,#14597,#8348,.T.);
#18555=EDGE_CURVE('',#14829,#14828,#8349,.T.);
#18556=EDGE_CURVE('',#14830,#14829,#8350,.T.);
#18557=EDGE_CURVE('',#14830,#14643,#8351,.T.);
#18558=EDGE_CURVE('',#14831,#14641,#8352,.T.);
#18559=EDGE_CURVE('',#14831,#14832,#8353,.T.);
#18560=EDGE_CURVE('',#14833,#14832,#8354,.T.);
#18561=EDGE_CURVE('',#14834,#14833,#8355,.T.);
#18562=EDGE_CURVE('',#14583,#14834,#8356,.T.);
#18563=EDGE_CURVE('',#14591,#14835,#8357,.T.);
#18564=EDGE_CURVE('',#14835,#14836,#8358,.T.);
#18565=EDGE_CURVE('',#14837,#14836,#8359,.T.);
#18566=EDGE_CURVE('',#14838,#14837,#8360,.T.);
#18567=EDGE_CURVE('',#14838,#14644,#8361,.T.);
#18568=EDGE_CURVE('',#14839,#14642,#8362,.T.);
#18569=EDGE_CURVE('',#14839,#14840,#8363,.T.);
#18570=EDGE_CURVE('',#14841,#14840,#8364,.T.);
#18571=EDGE_CURVE('',#14841,#14595,#8365,.T.);
#18572=EDGE_CURVE('',#14835,#14386,#11909,.T.);
#18573=EDGE_CURVE('',#14548,#14842,#8366,.T.);
#18574=EDGE_CURVE('',#14391,#14842,#11910,.T.);
#18575=EDGE_CURVE('',#14843,#14830,#11911,.T.);
#18576=EDGE_CURVE('',#14843,#14844,#8367,.T.);
#18577=EDGE_CURVE('',#14831,#14844,#11912,.T.);
#18578=EDGE_CURVE('',#14383,#14834,#11913,.T.);
#18579=EDGE_CURVE('',#14821,#14363,#11914,.T.);
#18580=EDGE_CURVE('',#14845,#14824,#11915,.T.);
#18581=EDGE_CURVE('',#14846,#14845,#8368,.T.);
#18582=EDGE_CURVE('',#14825,#14846,#11916,.T.);
#18583=EDGE_CURVE('',#14847,#14816,#11917,.T.);
#18584=EDGE_CURVE('',#14848,#14847,#8369,.T.);
#18585=EDGE_CURVE('',#14817,#14848,#11918,.T.);
#18586=EDGE_CURVE('',#14536,#14849,#8370,.T.);
#18587=EDGE_CURVE('',#14352,#14849,#11919,.T.);
#18588=EDGE_CURVE('',#14850,#14394,#11920,.T.);
#18589=EDGE_CURVE('',#14540,#14850,#8371,.T.);
#18590=EDGE_CURVE('',#14851,#14838,#11921,.T.);
#18591=EDGE_CURVE('',#14851,#14852,#8372,.T.);
#18592=EDGE_CURVE('',#14839,#14852,#11922,.T.);
#18593=EDGE_CURVE('',#14360,#14820,#11923,.T.);
#18594=EDGE_CURVE('',#14853,#14355,#11924,.T.);
#18595=EDGE_CURVE('',#14530,#14853,#8373,.T.);
#18596=EDGE_CURVE('',#14854,#14837,#11925,.T.);
#18597=EDGE_CURVE('',#14855,#14836,#11926,.T.);
#18598=EDGE_CURVE('',#14854,#14855,#8374,.T.);
#18599=EDGE_CURVE('',#14836,#14385,#11927,.T.);
#18600=EDGE_CURVE('',#14855,#14385,#11928,.T.);
#18601=EDGE_CURVE('',#14856,#14837,#11929,.T.);
#18602=EDGE_CURVE('',#14851,#14856,#8375,.T.);
#18603=EDGE_CURVE('',#14854,#14856,#11930,.T.);
#18604=EDGE_CURVE('',#14857,#14384,#11931,.T.);
#18605=EDGE_CURVE('',#14855,#14857,#11932,.T.);
#18606=EDGE_CURVE('',#14384,#14833,#11933,.T.);
#18607=EDGE_CURVE('',#14857,#14833,#11934,.T.);
#18608=EDGE_CURVE('',#14857,#14858,#8376,.T.);
#18609=EDGE_CURVE('',#14858,#14859,#8377,.T.);
#18610=EDGE_CURVE('',#14859,#14860,#8378,.T.);
#18611=EDGE_CURVE('',#14860,#14861,#11935,.T.);
#18612=EDGE_CURVE('',#14861,#14862,#11936,.T.);
#18613=EDGE_CURVE('',#14862,#14863,#11937,.T.);
#18614=EDGE_CURVE('',#14863,#14864,#8379,.T.);
#18615=EDGE_CURVE('',#14864,#14854,#8380,.T.);
#18616=EDGE_CURVE('',#14864,#14865,#11938,.T.);
#18617=EDGE_CURVE('',#14865,#14856,#8381,.T.);
#18618=EDGE_CURVE('',#14864,#14840,#11939,.T.);
#18619=EDGE_CURVE('',#14840,#14865,#11940,.T.);
#18620=EDGE_CURVE('',#14858,#14832,#11941,.T.);
#18621=EDGE_CURVE('',#14832,#14866,#11942,.T.);
#18622=EDGE_CURVE('',#14858,#14866,#11943,.T.);
#18623=EDGE_CURVE('',#14866,#14867,#8382,.T.);
#18624=EDGE_CURVE('',#14859,#14867,#11944,.T.);
#18625=EDGE_CURVE('',#14867,#14829,#11945,.T.);
#18626=EDGE_CURVE('',#14859,#14829,#11946,.T.);
#18627=EDGE_CURVE('',#14860,#14828,#11947,.T.);
#18628=EDGE_CURVE('',#14828,#14589,#11948,.T.);
#18629=EDGE_CURVE('',#14861,#14589,#11949,.T.);
#18630=EDGE_CURVE('',#14862,#14588,#11950,.T.);
#18631=EDGE_CURVE('',#14588,#14841,#11951,.T.);
#18632=EDGE_CURVE('',#14863,#14841,#11952,.T.);
#18633=EDGE_CURVE('',#14852,#14865,#8383,.T.);
#18634=EDGE_CURVE('',#14844,#14866,#8384,.T.);
#18635=EDGE_CURVE('',#14843,#14867,#8385,.T.);
#18636=EDGE_CURVE('',#14850,#14868,#8386,.T.);
#18637=EDGE_CURVE('',#14869,#14868,#8387,.T.);
#18638=EDGE_CURVE('',#14610,#14869,#8388,.T.);
#18639=EDGE_CURVE('',#14870,#14869,#11953,.T.);
#18640=EDGE_CURVE('',#14871,#14868,#11954,.T.);
#18641=EDGE_CURVE('',#14870,#14871,#8389,.T.);
#18642=EDGE_CURVE('',#14868,#14393,#11955,.T.);
#18643=EDGE_CURVE('',#14871,#14393,#11956,.T.);
#18644=EDGE_CURVE('',#14611,#14872,#8390,.T.);
#18645=EDGE_CURVE('',#14872,#14869,#11957,.T.);
#18646=EDGE_CURVE('',#14870,#14872,#11958,.T.);
#18647=EDGE_CURVE('',#14873,#14392,#11959,.T.);
#18648=EDGE_CURVE('',#14871,#14873,#11960,.T.);
#18649=EDGE_CURVE('',#14842,#14874,#8391,.T.);
#18650=EDGE_CURVE('',#14392,#14874,#11961,.T.);
#18651=EDGE_CURVE('',#14873,#14874,#11962,.T.);
#18652=EDGE_CURVE('',#14873,#14875,#8392,.T.);
#18653=EDGE_CURVE('',#14875,#14876,#8393,.T.);
#18654=EDGE_CURVE('',#14876,#14877,#8394,.T.);
#18655=EDGE_CURVE('',#14877,#14878,#11963,.T.);
#18656=EDGE_CURVE('',#14878,#14879,#11964,.T.);
#18657=EDGE_CURVE('',#14879,#14880,#11965,.T.);
#18658=EDGE_CURVE('',#14880,#14881,#8395,.T.);
#18659=EDGE_CURVE('',#14881,#14870,#8396,.T.);
#18660=EDGE_CURVE('',#14881,#14882,#11966,.T.);
#18661=EDGE_CURVE('',#14882,#14872,#8397,.T.);
#18662=EDGE_CURVE('',#14881,#14883,#11967,.T.);
#18663=EDGE_CURVE('',#14883,#14882,#11968,.T.);
#18664=EDGE_CURVE('',#14874,#14884,#8398,.T.);
#18665=EDGE_CURVE('',#14875,#14884,#11969,.T.);
#18666=EDGE_CURVE('',#14884,#14885,#11970,.T.);
#18667=EDGE_CURVE('',#14875,#14885,#11971,.T.);
#18668=EDGE_CURVE('',#14885,#14886,#8399,.T.);
#18669=EDGE_CURVE('',#14876,#14886,#11972,.T.);
#18670=EDGE_CURVE('',#14886,#14887,#11973,.T.);
#18671=EDGE_CURVE('',#14876,#14887,#11974,.T.);
#18672=EDGE_CURVE('',#14887,#14888,#8400,.T.);
#18673=EDGE_CURVE('',#14877,#14888,#11975,.T.);
#18674=EDGE_CURVE('',#14888,#14546,#11976,.T.);
#18675=EDGE_CURVE('',#14878,#14546,#11977,.T.);
#18676=EDGE_CURVE('',#14879,#14545,#11978,.T.);
#18677=EDGE_CURVE('',#14545,#14889,#11979,.T.);
#18678=EDGE_CURVE('',#14880,#14889,#11980,.T.);
#18679=EDGE_CURVE('',#14889,#14883,#8401,.T.);
#18680=EDGE_CURVE('',#14612,#14882,#8402,.T.);
#18681=EDGE_CURVE('',#14613,#14883,#8403,.T.);
#18682=EDGE_CURVE('',#14603,#14884,#8404,.T.);
#18683=EDGE_CURVE('',#14602,#14885,#8405,.T.);
#18684=EDGE_CURVE('',#14601,#14886,#8406,.T.);
#18685=EDGE_CURVE('',#14600,#14887,#8407,.T.);
#18686=EDGE_CURVE('',#14888,#14599,#8408,.T.);
#18687=EDGE_CURVE('',#14889,#14614,#8409,.T.);
#18688=EDGE_CURVE('',#14818,#14890,#11981,.T.);
#18689=EDGE_CURVE('',#14890,#14891,#8410,.T.);
#18690=EDGE_CURVE('',#14819,#14891,#11982,.T.);
#18691=EDGE_CURVE('',#14819,#14361,#11983,.T.);
#18692=EDGE_CURVE('',#14361,#14891,#11984,.T.);
#18693=EDGE_CURVE('',#14848,#14892,#8411,.T.);
#18694=EDGE_CURVE('',#14892,#14818,#11985,.T.);
#18695=EDGE_CURVE('',#14892,#14890,#11986,.T.);
#18696=EDGE_CURVE('',#14891,#14893,#11987,.T.);
#18697=EDGE_CURVE('',#14362,#14893,#11988,.T.);
#18698=EDGE_CURVE('',#14362,#14822,#11989,.T.);
#18699=EDGE_CURVE('',#14822,#14893,#11990,.T.);
#18700=EDGE_CURVE('',#14894,#14890,#8412,.T.);
#18701=EDGE_CURVE('',#14895,#14894,#8413,.T.);
#18702=EDGE_CURVE('',#14896,#14895,#11991,.T.);
#18703=EDGE_CURVE('',#14897,#14896,#11992,.T.);
#18704=EDGE_CURVE('',#14898,#14897,#11993,.T.);
#18705=EDGE_CURVE('',#14899,#14898,#8414,.T.);
#18706=EDGE_CURVE('',#14900,#14899,#8415,.T.);
#18707=EDGE_CURVE('',#14893,#14900,#8416,.T.);
#18708=EDGE_CURVE('',#14901,#14894,#11994,.T.);
#18709=EDGE_CURVE('',#14901,#14892,#8417,.T.);
#18710=EDGE_CURVE('',#14815,#14894,#11995,.T.);
#18711=EDGE_CURVE('',#14815,#14901,#11996,.T.);
#18712=EDGE_CURVE('',#14823,#14900,#11997,.T.);
#18713=EDGE_CURVE('',#14902,#14900,#11998,.T.);
#18714=EDGE_CURVE('',#14823,#14902,#11999,.T.);
#18715=EDGE_CURVE('',#14903,#14899,#12000,.T.);
#18716=EDGE_CURVE('',#14902,#14903,#8418,.T.);
#18717=EDGE_CURVE('',#14826,#14899,#12001,.T.);
#18718=EDGE_CURVE('',#14903,#14826,#12002,.T.);
#18719=EDGE_CURVE('',#14827,#14898,#12003,.T.);
#18720=EDGE_CURVE('',#14578,#14897,#12004,.T.);
#18721=EDGE_CURVE('',#14827,#14578,#12005,.T.);
#18722=EDGE_CURVE('',#14579,#14896,#12006,.T.);
#18723=EDGE_CURVE('',#14814,#14895,#12007,.T.);
#18724=EDGE_CURVE('',#14579,#14814,#12008,.T.);
#18725=EDGE_CURVE('',#14847,#14901,#8419,.T.);
#18726=EDGE_CURVE('',#14845,#14902,#8420,.T.);
#18727=EDGE_CURVE('',#14846,#14903,#8421,.T.);
#18728=EDGE_CURVE('',#14571,#14904,#8422,.T.);
#18729=EDGE_CURVE('',#14904,#14905,#8423,.T.);
#18730=EDGE_CURVE('',#14849,#14905,#8424,.T.);
#18731=EDGE_CURVE('',#14904,#14906,#12009,.T.);
#18732=EDGE_CURVE('',#14906,#14907,#8425,.T.);
#18733=EDGE_CURVE('',#14905,#14907,#12010,.T.);
#18734=EDGE_CURVE('',#14570,#14908,#8426,.T.);
#18735=EDGE_CURVE('',#14908,#14904,#12011,.T.);
#18736=EDGE_CURVE('',#14908,#14906,#12012,.T.);
#18737=EDGE_CURVE('',#14905,#14353,#12013,.T.);
#18738=EDGE_CURVE('',#14353,#14907,#12014,.T.);
#18739=EDGE_CURVE('',#14909,#14906,#8427,.T.);
#18740=EDGE_CURVE('',#14910,#14909,#8428,.T.);
#18741=EDGE_CURVE('',#14911,#14910,#12015,.T.);
#18742=EDGE_CURVE('',#14912,#14911,#12016,.T.);
#18743=EDGE_CURVE('',#14913,#14912,#12017,.T.);
#18744=EDGE_CURVE('',#14914,#14913,#8429,.T.);
#18745=EDGE_CURVE('',#14915,#14914,#8430,.T.);
#18746=EDGE_CURVE('',#14916,#14915,#8431,.T.);
#18747=EDGE_CURVE('',#14907,#14916,#12018,.T.);
#18748=EDGE_CURVE('',#14917,#14909,#12019,.T.);
#18749=EDGE_CURVE('',#14917,#14908,#8432,.T.);
#18750=EDGE_CURVE('',#14918,#14909,#12020,.T.);
#18751=EDGE_CURVE('',#14918,#14917,#12021,.T.);
#18752=EDGE_CURVE('',#14354,#14916,#12022,.T.);
#18753=EDGE_CURVE('',#14919,#14916,#12023,.T.);
#18754=EDGE_CURVE('',#14354,#14919,#12024,.T.);
#18755=EDGE_CURVE('',#14920,#14915,#12025,.T.);
#18756=EDGE_CURVE('',#14921,#14914,#12026,.T.);
#18757=EDGE_CURVE('',#14920,#14921,#8433,.T.);
#18758=EDGE_CURVE('',#14922,#14915,#12027,.T.);
#18759=EDGE_CURVE('',#14922,#14920,#12028,.T.);
#18760=EDGE_CURVE('',#14923,#14914,#12029,.T.);
#18761=EDGE_CURVE('',#14921,#14923,#12030,.T.);
#18762=EDGE_CURVE('',#14919,#14922,#8434,.T.);
#18763=EDGE_CURVE('',#14924,#14913,#12031,.T.);
#18764=EDGE_CURVE('',#14923,#14924,#8435,.T.);
#18765=EDGE_CURVE('',#14533,#14912,#12032,.T.);
#18766=EDGE_CURVE('',#14924,#14533,#12033,.T.);
#18767=EDGE_CURVE('',#14534,#14911,#12034,.T.);
#18768=EDGE_CURVE('',#14925,#14910,#12035,.T.);
#18769=EDGE_CURVE('',#14534,#14925,#12036,.T.);
#18770=EDGE_CURVE('',#14925,#14918,#8436,.T.);
#18771=EDGE_CURVE('',#14569,#14917,#8437,.T.);
#18772=EDGE_CURVE('',#14568,#14918,#8438,.T.);
#18773=EDGE_CURVE('',#14853,#14919,#8439,.T.);
#18774=EDGE_CURVE('',#14564,#14921,#8440,.T.);
#18775=EDGE_CURVE('',#14563,#14920,#8441,.T.);
#18776=EDGE_CURVE('',#14562,#14922,#8442,.T.);
#18777=EDGE_CURVE('',#14565,#14923,#8443,.T.);
#18778=EDGE_CURVE('',#14924,#14566,#8444,.T.);
#18779=EDGE_CURVE('',#14925,#14567,#8445,.T.);
#23937=ORIENTED_EDGE('',*,*,#17740,.T.);
#23938=ORIENTED_EDGE('',*,*,#17741,.F.);
#23939=ORIENTED_EDGE('',*,*,#17742,.F.);
#23940=ORIENTED_EDGE('',*,*,#17743,.F.);
#23941=ORIENTED_EDGE('',*,*,#17742,.T.);
#23942=ORIENTED_EDGE('',*,*,#17744,.F.);
#23943=ORIENTED_EDGE('',*,*,#17745,.F.);
#23944=ORIENTED_EDGE('',*,*,#17746,.F.);
#23945=ORIENTED_EDGE('',*,*,#17747,.F.);
#23946=ORIENTED_EDGE('',*,*,#17744,.T.);
#23947=ORIENTED_EDGE('',*,*,#17741,.T.);
#23948=ORIENTED_EDGE('',*,*,#17743,.T.);
#23949=ORIENTED_EDGE('',*,*,#17748,.T.);
#23950=ORIENTED_EDGE('',*,*,#17746,.T.);
#23951=ORIENTED_EDGE('',*,*,#17740,.F.);
#23952=ORIENTED_EDGE('',*,*,#17745,.T.);
#23953=ORIENTED_EDGE('',*,*,#17747,.T.);
#23954=ORIENTED_EDGE('',*,*,#17748,.F.);
#23955=ORIENTED_EDGE('',*,*,#17749,.F.);
#23956=ORIENTED_EDGE('',*,*,#17750,.T.);
#23957=ORIENTED_EDGE('',*,*,#17751,.T.);
#23958=ORIENTED_EDGE('',*,*,#17752,.F.);
#23959=ORIENTED_EDGE('',*,*,#17753,.T.);
#23960=ORIENTED_EDGE('',*,*,#17754,.T.);
#23961=ORIENTED_EDGE('',*,*,#17751,.F.);
#23962=ORIENTED_EDGE('',*,*,#17752,.T.);
#23963=ORIENTED_EDGE('',*,*,#17750,.F.);
#23964=ORIENTED_EDGE('',*,*,#17755,.F.);
#23965=ORIENTED_EDGE('',*,*,#17756,.T.);
#23966=ORIENTED_EDGE('',*,*,#17754,.F.);
#23967=ORIENTED_EDGE('',*,*,#17757,.F.);
#23968=ORIENTED_EDGE('',*,*,#17755,.T.);
#23969=ORIENTED_EDGE('',*,*,#17749,.T.);
#23970=ORIENTED_EDGE('',*,*,#17757,.T.);
#23971=ORIENTED_EDGE('',*,*,#17753,.F.);
#23972=ORIENTED_EDGE('',*,*,#17756,.F.);
#23973=ORIENTED_EDGE('',*,*,#17758,.T.);
#23974=ORIENTED_EDGE('',*,*,#17759,.T.);
#23975=ORIENTED_EDGE('',*,*,#17760,.F.);
#23976=ORIENTED_EDGE('',*,*,#17761,.F.);
#23977=ORIENTED_EDGE('',*,*,#17762,.F.);
#23978=ORIENTED_EDGE('',*,*,#17763,.F.);
#23979=ORIENTED_EDGE('',*,*,#17764,.F.);
#23980=ORIENTED_EDGE('',*,*,#17765,.T.);
#23981=ORIENTED_EDGE('',*,*,#17766,.T.);
#23982=ORIENTED_EDGE('',*,*,#17767,.T.);
#23983=ORIENTED_EDGE('',*,*,#17768,.T.);
#23984=ORIENTED_EDGE('',*,*,#17769,.T.);
#23985=ORIENTED_EDGE('',*,*,#17770,.F.);
#23986=ORIENTED_EDGE('',*,*,#17771,.F.);
#23987=ORIENTED_EDGE('',*,*,#17772,.T.);
#23988=ORIENTED_EDGE('',*,*,#17773,.F.);
#23989=ORIENTED_EDGE('',*,*,#17774,.F.);
#23990=ORIENTED_EDGE('',*,*,#17775,.F.);
#23991=ORIENTED_EDGE('',*,*,#17776,.T.);
#23992=ORIENTED_EDGE('',*,*,#17777,.T.);
#23993=ORIENTED_EDGE('',*,*,#17778,.T.);
#23994=ORIENTED_EDGE('',*,*,#17779,.T.);
#23995=ORIENTED_EDGE('',*,*,#17780,.T.);
#23996=ORIENTED_EDGE('',*,*,#17781,.T.);
#23997=ORIENTED_EDGE('',*,*,#17782,.T.);
#23998=ORIENTED_EDGE('',*,*,#17783,.F.);
#23999=ORIENTED_EDGE('',*,*,#17784,.F.);
#24000=ORIENTED_EDGE('',*,*,#17785,.F.);
#24001=ORIENTED_EDGE('',*,*,#17786,.T.);
#24002=ORIENTED_EDGE('',*,*,#17787,.F.);
#24003=ORIENTED_EDGE('',*,*,#17788,.F.);
#24004=ORIENTED_EDGE('',*,*,#17789,.T.);
#24005=ORIENTED_EDGE('',*,*,#17790,.T.);
#24006=ORIENTED_EDGE('',*,*,#17791,.F.);
#24007=ORIENTED_EDGE('',*,*,#17792,.T.);
#24008=ORIENTED_EDGE('',*,*,#17793,.T.);
#24009=ORIENTED_EDGE('',*,*,#17794,.F.);
#24010=ORIENTED_EDGE('',*,*,#17795,.T.);
#24011=ORIENTED_EDGE('',*,*,#17796,.F.);
#24012=ORIENTED_EDGE('',*,*,#17797,.F.);
#24013=ORIENTED_EDGE('',*,*,#17798,.T.);
#24014=ORIENTED_EDGE('',*,*,#17799,.F.);
#24015=ORIENTED_EDGE('',*,*,#17800,.T.);
#24016=ORIENTED_EDGE('',*,*,#17801,.T.);
#24017=ORIENTED_EDGE('',*,*,#17802,.T.);
#24018=ORIENTED_EDGE('',*,*,#17803,.F.);
#24019=ORIENTED_EDGE('',*,*,#17804,.T.);
#24020=ORIENTED_EDGE('',*,*,#17805,.F.);
#24021=ORIENTED_EDGE('',*,*,#17771,.T.);
#24022=ORIENTED_EDGE('',*,*,#17806,.T.);
#24023=ORIENTED_EDGE('',*,*,#17807,.T.);
#24024=ORIENTED_EDGE('',*,*,#17808,.T.);
#24025=ORIENTED_EDGE('',*,*,#17809,.T.);
#24026=ORIENTED_EDGE('',*,*,#17810,.T.);
#24027=ORIENTED_EDGE('',*,*,#17811,.T.);
#24028=ORIENTED_EDGE('',*,*,#17812,.F.);
#24029=ORIENTED_EDGE('',*,*,#17813,.T.);
#24030=ORIENTED_EDGE('',*,*,#17814,.T.);
#24031=ORIENTED_EDGE('',*,*,#17815,.T.);
#24032=ORIENTED_EDGE('',*,*,#17816,.T.);
#24033=ORIENTED_EDGE('',*,*,#17817,.T.);
#24034=ORIENTED_EDGE('',*,*,#17818,.T.);
#24035=ORIENTED_EDGE('',*,*,#17819,.F.);
#24036=ORIENTED_EDGE('',*,*,#17820,.T.);
#24037=ORIENTED_EDGE('',*,*,#17821,.F.);
#24038=ORIENTED_EDGE('',*,*,#17765,.F.);
#24039=ORIENTED_EDGE('',*,*,#17822,.T.);
#24040=ORIENTED_EDGE('',*,*,#17823,.T.);
#24041=ORIENTED_EDGE('',*,*,#17824,.F.);
#24042=ORIENTED_EDGE('',*,*,#17825,.T.);
#24043=ORIENTED_EDGE('',*,*,#17826,.T.);
#24044=ORIENTED_EDGE('',*,*,#17827,.F.);
#24045=ORIENTED_EDGE('',*,*,#17828,.F.);
#24046=ORIENTED_EDGE('',*,*,#17829,.F.);
#24047=ORIENTED_EDGE('',*,*,#17770,.T.);
#24048=ORIENTED_EDGE('',*,*,#17830,.T.);
#24049=ORIENTED_EDGE('',*,*,#17831,.F.);
#24050=ORIENTED_EDGE('',*,*,#17806,.F.);
#24051=ORIENTED_EDGE('',*,*,#17769,.F.);
#24052=ORIENTED_EDGE('',*,*,#17832,.T.);
#24053=ORIENTED_EDGE('',*,*,#17833,.F.);
#24054=ORIENTED_EDGE('',*,*,#17830,.F.);
#24055=ORIENTED_EDGE('',*,*,#17768,.F.);
#24056=ORIENTED_EDGE('',*,*,#17834,.T.);
#24057=ORIENTED_EDGE('',*,*,#17835,.F.);
#24058=ORIENTED_EDGE('',*,*,#17836,.F.);
#24059=ORIENTED_EDGE('',*,*,#17837,.T.);
#24060=ORIENTED_EDGE('',*,*,#17838,.F.);
#24061=ORIENTED_EDGE('',*,*,#17839,.F.);
#24062=ORIENTED_EDGE('',*,*,#17832,.F.);
#24063=ORIENTED_EDGE('',*,*,#17805,.T.);
#24064=ORIENTED_EDGE('',*,*,#17840,.T.);
#24065=ORIENTED_EDGE('',*,*,#17841,.F.);
#24066=ORIENTED_EDGE('',*,*,#17834,.F.);
#24067=ORIENTED_EDGE('',*,*,#17767,.F.);
#24068=ORIENTED_EDGE('',*,*,#17842,.T.);
#24069=ORIENTED_EDGE('',*,*,#17843,.T.);
#24070=ORIENTED_EDGE('',*,*,#17844,.F.);
#24071=ORIENTED_EDGE('',*,*,#17845,.T.);
#24072=ORIENTED_EDGE('',*,*,#17846,.F.);
#24073=ORIENTED_EDGE('',*,*,#17847,.T.);
#24074=ORIENTED_EDGE('',*,*,#17848,.T.);
#24075=ORIENTED_EDGE('',*,*,#17849,.T.);
#24076=ORIENTED_EDGE('',*,*,#17850,.T.);
#24077=ORIENTED_EDGE('',*,*,#17851,.T.);
#24078=ORIENTED_EDGE('',*,*,#17852,.F.);
#24079=ORIENTED_EDGE('',*,*,#17853,.T.);
#24080=ORIENTED_EDGE('',*,*,#17854,.T.);
#24081=ORIENTED_EDGE('',*,*,#17855,.T.);
#24082=ORIENTED_EDGE('',*,*,#17856,.T.);
#24083=ORIENTED_EDGE('',*,*,#17787,.T.);
#24084=ORIENTED_EDGE('',*,*,#17857,.F.);
#24085=ORIENTED_EDGE('',*,*,#17858,.T.);
#24086=ORIENTED_EDGE('',*,*,#17859,.F.);
#24087=ORIENTED_EDGE('',*,*,#17860,.T.);
#24088=ORIENTED_EDGE('',*,*,#17786,.F.);
#24089=ORIENTED_EDGE('',*,*,#17861,.T.);
#24090=ORIENTED_EDGE('',*,*,#17862,.T.);
#24091=ORIENTED_EDGE('',*,*,#17857,.T.);
#24092=ORIENTED_EDGE('',*,*,#17861,.F.);
#24093=ORIENTED_EDGE('',*,*,#17785,.T.);
#24094=ORIENTED_EDGE('',*,*,#17863,.T.);
#24095=ORIENTED_EDGE('',*,*,#17864,.F.);
#24096=ORIENTED_EDGE('',*,*,#17865,.F.);
#24097=ORIENTED_EDGE('',*,*,#17863,.F.);
#24098=ORIENTED_EDGE('',*,*,#17784,.T.);
#24099=ORIENTED_EDGE('',*,*,#17866,.T.);
#24100=ORIENTED_EDGE('',*,*,#17783,.T.);
#24101=ORIENTED_EDGE('',*,*,#17867,.T.);
#24102=ORIENTED_EDGE('',*,*,#17868,.T.);
#24103=ORIENTED_EDGE('',*,*,#17869,.F.);
#24104=ORIENTED_EDGE('',*,*,#17870,.F.);
#24105=ORIENTED_EDGE('',*,*,#17871,.T.);
#24106=ORIENTED_EDGE('',*,*,#17872,.F.);
#24107=ORIENTED_EDGE('',*,*,#17873,.T.);
#24108=ORIENTED_EDGE('',*,*,#17874,.T.);
#24109=ORIENTED_EDGE('',*,*,#17866,.F.);
#24110=ORIENTED_EDGE('',*,*,#17782,.F.);
#24111=ORIENTED_EDGE('',*,*,#17875,.T.);
#24112=ORIENTED_EDGE('',*,*,#17876,.T.);
#24113=ORIENTED_EDGE('',*,*,#17867,.F.);
#24114=ORIENTED_EDGE('',*,*,#17781,.F.);
#24115=ORIENTED_EDGE('',*,*,#17877,.T.);
#24116=ORIENTED_EDGE('',*,*,#17878,.T.);
#24117=ORIENTED_EDGE('',*,*,#17875,.F.);
#24118=ORIENTED_EDGE('',*,*,#17879,.F.);
#24119=ORIENTED_EDGE('',*,*,#17880,.T.);
#24120=ORIENTED_EDGE('',*,*,#17877,.F.);
#24121=ORIENTED_EDGE('',*,*,#17780,.F.);
#24122=ORIENTED_EDGE('',*,*,#17881,.T.);
#24123=ORIENTED_EDGE('',*,*,#17882,.F.);
#24124=ORIENTED_EDGE('',*,*,#17883,.F.);
#24125=ORIENTED_EDGE('',*,*,#17884,.T.);
#24126=ORIENTED_EDGE('',*,*,#17885,.F.);
#24127=ORIENTED_EDGE('',*,*,#17886,.F.);
#24128=ORIENTED_EDGE('',*,*,#17887,.T.);
#24129=ORIENTED_EDGE('',*,*,#17888,.T.);
#24130=ORIENTED_EDGE('',*,*,#17889,.T.);
#24131=ORIENTED_EDGE('',*,*,#17890,.F.);
#24132=ORIENTED_EDGE('',*,*,#17891,.F.);
#24133=ORIENTED_EDGE('',*,*,#17892,.T.);
#24134=ORIENTED_EDGE('',*,*,#17893,.T.);
#24135=ORIENTED_EDGE('',*,*,#17894,.T.);
#24136=ORIENTED_EDGE('',*,*,#17879,.T.);
#24137=ORIENTED_EDGE('',*,*,#17779,.F.);
#24138=ORIENTED_EDGE('',*,*,#17895,.F.);
#24139=ORIENTED_EDGE('',*,*,#17896,.T.);
#24140=ORIENTED_EDGE('',*,*,#17897,.F.);
#24141=ORIENTED_EDGE('',*,*,#17898,.T.);
#24142=ORIENTED_EDGE('',*,*,#17778,.F.);
#24143=ORIENTED_EDGE('',*,*,#17899,.T.);
#24144=ORIENTED_EDGE('',*,*,#17900,.T.);
#24145=ORIENTED_EDGE('',*,*,#17895,.T.);
#24146=ORIENTED_EDGE('',*,*,#17901,.T.);
#24147=ORIENTED_EDGE('',*,*,#17902,.T.);
#24148=ORIENTED_EDGE('',*,*,#17899,.F.);
#24149=ORIENTED_EDGE('',*,*,#17777,.F.);
#24150=ORIENTED_EDGE('',*,*,#17903,.T.);
#24151=ORIENTED_EDGE('',*,*,#17901,.F.);
#24152=ORIENTED_EDGE('',*,*,#17776,.F.);
#24153=ORIENTED_EDGE('',*,*,#17904,.T.);
#24154=ORIENTED_EDGE('',*,*,#17775,.T.);
#24155=ORIENTED_EDGE('',*,*,#17905,.T.);
#24156=ORIENTED_EDGE('',*,*,#17906,.T.);
#24157=ORIENTED_EDGE('',*,*,#17907,.F.);
#24158=ORIENTED_EDGE('',*,*,#17908,.F.);
#24159=ORIENTED_EDGE('',*,*,#17909,.T.);
#24160=ORIENTED_EDGE('',*,*,#17910,.F.);
#24161=ORIENTED_EDGE('',*,*,#17911,.T.);
#24162=ORIENTED_EDGE('',*,*,#17912,.T.);
#24163=ORIENTED_EDGE('',*,*,#17904,.F.);
#24164=ORIENTED_EDGE('',*,*,#17774,.T.);
#24165=ORIENTED_EDGE('',*,*,#17913,.T.);
#24166=ORIENTED_EDGE('',*,*,#17914,.F.);
#24167=ORIENTED_EDGE('',*,*,#17905,.F.);
#24168=ORIENTED_EDGE('',*,*,#17915,.F.);
#24169=ORIENTED_EDGE('',*,*,#17913,.F.);
#24170=ORIENTED_EDGE('',*,*,#17773,.T.);
#24171=ORIENTED_EDGE('',*,*,#17916,.T.);
#24172=ORIENTED_EDGE('',*,*,#17856,.F.);
#24173=ORIENTED_EDGE('',*,*,#17917,.T.);
#24174=ORIENTED_EDGE('',*,*,#17916,.F.);
#24175=ORIENTED_EDGE('',*,*,#17772,.F.);
#24176=ORIENTED_EDGE('',*,*,#17918,.F.);
#24177=ORIENTED_EDGE('',*,*,#17793,.F.);
#24178=ORIENTED_EDGE('',*,*,#17919,.T.);
#24179=ORIENTED_EDGE('',*,*,#17920,.T.);
#24180=ORIENTED_EDGE('',*,*,#17921,.T.);
#24181=ORIENTED_EDGE('',*,*,#17922,.T.);
#24182=ORIENTED_EDGE('',*,*,#17792,.F.);
#24183=ORIENTED_EDGE('',*,*,#17923,.T.);
#24184=ORIENTED_EDGE('',*,*,#17924,.F.);
#24185=ORIENTED_EDGE('',*,*,#17925,.F.);
#24186=ORIENTED_EDGE('',*,*,#17919,.F.);
#24187=ORIENTED_EDGE('',*,*,#17791,.T.);
#24188=ORIENTED_EDGE('',*,*,#17926,.T.);
#24189=ORIENTED_EDGE('',*,*,#17927,.F.);
#24190=ORIENTED_EDGE('',*,*,#17928,.F.);
#24191=ORIENTED_EDGE('',*,*,#17929,.F.);
#24192=ORIENTED_EDGE('',*,*,#17930,.F.);
#24193=ORIENTED_EDGE('',*,*,#17923,.F.);
#24194=ORIENTED_EDGE('',*,*,#17790,.F.);
#24195=ORIENTED_EDGE('',*,*,#17931,.T.);
#24196=ORIENTED_EDGE('',*,*,#17932,.T.);
#24197=ORIENTED_EDGE('',*,*,#17926,.F.);
#24198=ORIENTED_EDGE('',*,*,#17933,.F.);
#24199=ORIENTED_EDGE('',*,*,#17934,.F.);
#24200=ORIENTED_EDGE('',*,*,#17935,.F.);
#24201=ORIENTED_EDGE('',*,*,#17936,.F.);
#24202=ORIENTED_EDGE('',*,*,#17931,.F.);
#24203=ORIENTED_EDGE('',*,*,#17789,.F.);
#24204=ORIENTED_EDGE('',*,*,#17937,.T.);
#24205=ORIENTED_EDGE('',*,*,#17788,.T.);
#24206=ORIENTED_EDGE('',*,*,#17918,.T.);
#24207=ORIENTED_EDGE('',*,*,#17938,.F.);
#24208=ORIENTED_EDGE('',*,*,#17939,.F.);
#24209=ORIENTED_EDGE('',*,*,#17937,.F.);
#24210=ORIENTED_EDGE('',*,*,#17940,.T.);
#24211=ORIENTED_EDGE('',*,*,#17941,.T.);
#24212=ORIENTED_EDGE('',*,*,#17942,.T.);
#24213=ORIENTED_EDGE('',*,*,#17943,.T.);
#24214=ORIENTED_EDGE('',*,*,#17800,.F.);
#24215=ORIENTED_EDGE('',*,*,#17799,.T.);
#24216=ORIENTED_EDGE('',*,*,#17944,.T.);
#24217=ORIENTED_EDGE('',*,*,#17945,.F.);
#24218=ORIENTED_EDGE('',*,*,#17946,.F.);
#24219=ORIENTED_EDGE('',*,*,#17940,.F.);
#24220=ORIENTED_EDGE('',*,*,#17944,.F.);
#24221=ORIENTED_EDGE('',*,*,#17798,.F.);
#24222=ORIENTED_EDGE('',*,*,#17947,.T.);
#24223=ORIENTED_EDGE('',*,*,#17948,.T.);
#24224=ORIENTED_EDGE('',*,*,#17797,.T.);
#24225=ORIENTED_EDGE('',*,*,#17949,.T.);
#24226=ORIENTED_EDGE('',*,*,#17950,.T.);
#24227=ORIENTED_EDGE('',*,*,#17951,.T.);
#24228=ORIENTED_EDGE('',*,*,#17947,.F.);
#24229=ORIENTED_EDGE('',*,*,#17949,.F.);
#24230=ORIENTED_EDGE('',*,*,#17796,.T.);
#24231=ORIENTED_EDGE('',*,*,#17952,.T.);
#24232=ORIENTED_EDGE('',*,*,#17953,.F.);
#24233=ORIENTED_EDGE('',*,*,#17954,.F.);
#24234=ORIENTED_EDGE('',*,*,#17955,.F.);
#24235=ORIENTED_EDGE('',*,*,#17956,.F.);
#24236=ORIENTED_EDGE('',*,*,#17952,.F.);
#24237=ORIENTED_EDGE('',*,*,#17795,.F.);
#24238=ORIENTED_EDGE('',*,*,#17794,.T.);
#24239=ORIENTED_EDGE('',*,*,#17943,.F.);
#24240=ORIENTED_EDGE('',*,*,#17957,.F.);
#24241=ORIENTED_EDGE('',*,*,#17954,.T.);
#24242=ORIENTED_EDGE('',*,*,#17804,.F.);
#24243=ORIENTED_EDGE('',*,*,#17958,.T.);
#24244=ORIENTED_EDGE('',*,*,#17959,.T.);
#24245=ORIENTED_EDGE('',*,*,#17840,.F.);
#24246=ORIENTED_EDGE('',*,*,#17837,.F.);
#24247=ORIENTED_EDGE('',*,*,#17960,.F.);
#24248=ORIENTED_EDGE('',*,*,#17958,.F.);
#24249=ORIENTED_EDGE('',*,*,#17803,.T.);
#24250=ORIENTED_EDGE('',*,*,#17961,.T.);
#24251=ORIENTED_EDGE('',*,*,#17961,.F.);
#24252=ORIENTED_EDGE('',*,*,#17802,.F.);
#24253=ORIENTED_EDGE('',*,*,#17962,.T.);
#24254=ORIENTED_EDGE('',*,*,#17838,.T.);
#24255=ORIENTED_EDGE('',*,*,#17962,.F.);
#24256=ORIENTED_EDGE('',*,*,#17801,.F.);
#24257=ORIENTED_EDGE('',*,*,#17831,.T.);
#24258=ORIENTED_EDGE('',*,*,#17833,.T.);
#24259=ORIENTED_EDGE('',*,*,#17839,.T.);
#24260=ORIENTED_EDGE('',*,*,#17813,.F.);
#24261=ORIENTED_EDGE('',*,*,#17963,.F.);
#24262=ORIENTED_EDGE('',*,*,#17964,.T.);
#24263=ORIENTED_EDGE('',*,*,#17965,.T.);
#24264=ORIENTED_EDGE('',*,*,#17812,.T.);
#24265=ORIENTED_EDGE('',*,*,#17966,.T.);
#24266=ORIENTED_EDGE('',*,*,#17967,.T.);
#24267=ORIENTED_EDGE('',*,*,#17963,.T.);
#24268=ORIENTED_EDGE('',*,*,#17968,.T.);
#24269=ORIENTED_EDGE('',*,*,#17969,.T.);
#24270=ORIENTED_EDGE('',*,*,#17970,.T.);
#24271=ORIENTED_EDGE('',*,*,#17966,.F.);
#24272=ORIENTED_EDGE('',*,*,#17811,.F.);
#24273=ORIENTED_EDGE('',*,*,#17971,.T.);
#24274=ORIENTED_EDGE('',*,*,#17972,.T.);
#24275=ORIENTED_EDGE('',*,*,#17973,.T.);
#24276=ORIENTED_EDGE('',*,*,#17968,.F.);
#24277=ORIENTED_EDGE('',*,*,#17810,.F.);
#24278=ORIENTED_EDGE('',*,*,#17971,.F.);
#24279=ORIENTED_EDGE('',*,*,#17809,.F.);
#24280=ORIENTED_EDGE('',*,*,#17974,.T.);
#24281=ORIENTED_EDGE('',*,*,#17975,.T.);
#24282=ORIENTED_EDGE('',*,*,#17976,.T.);
#24283=ORIENTED_EDGE('',*,*,#17974,.F.);
#24284=ORIENTED_EDGE('',*,*,#17808,.F.);
#24285=ORIENTED_EDGE('',*,*,#17977,.F.);
#24286=ORIENTED_EDGE('',*,*,#17978,.T.);
#24287=ORIENTED_EDGE('',*,*,#17979,.T.);
#24288=ORIENTED_EDGE('',*,*,#17980,.T.);
#24289=ORIENTED_EDGE('',*,*,#17977,.T.);
#24290=ORIENTED_EDGE('',*,*,#17807,.F.);
#24291=ORIENTED_EDGE('',*,*,#17965,.F.);
#24292=ORIENTED_EDGE('',*,*,#17981,.T.);
#24293=ORIENTED_EDGE('',*,*,#17982,.T.);
#24294=ORIENTED_EDGE('',*,*,#17983,.T.);
#24295=ORIENTED_EDGE('',*,*,#17979,.F.);
#24296=ORIENTED_EDGE('',*,*,#17984,.F.);
#24297=ORIENTED_EDGE('',*,*,#17822,.F.);
#24298=ORIENTED_EDGE('',*,*,#17764,.T.);
#24299=ORIENTED_EDGE('',*,*,#17985,.T.);
#24300=ORIENTED_EDGE('',*,*,#17986,.T.);
#24301=ORIENTED_EDGE('',*,*,#17987,.F.);
#24302=ORIENTED_EDGE('',*,*,#17766,.F.);
#24303=ORIENTED_EDGE('',*,*,#17821,.T.);
#24304=ORIENTED_EDGE('',*,*,#17988,.T.);
#24305=ORIENTED_EDGE('',*,*,#17986,.F.);
#24306=ORIENTED_EDGE('',*,*,#17820,.F.);
#24307=ORIENTED_EDGE('',*,*,#17989,.T.);
#24308=ORIENTED_EDGE('',*,*,#17990,.F.);
#24309=ORIENTED_EDGE('',*,*,#17989,.F.);
#24310=ORIENTED_EDGE('',*,*,#17819,.T.);
#24311=ORIENTED_EDGE('',*,*,#17991,.T.);
#24312=ORIENTED_EDGE('',*,*,#17992,.T.);
#24313=ORIENTED_EDGE('',*,*,#17991,.F.);
#24314=ORIENTED_EDGE('',*,*,#17818,.F.);
#24315=ORIENTED_EDGE('',*,*,#17993,.T.);
#24316=ORIENTED_EDGE('',*,*,#17994,.T.);
#24317=ORIENTED_EDGE('',*,*,#17993,.F.);
#24318=ORIENTED_EDGE('',*,*,#17817,.F.);
#24319=ORIENTED_EDGE('',*,*,#17995,.T.);
#24320=ORIENTED_EDGE('',*,*,#17995,.F.);
#24321=ORIENTED_EDGE('',*,*,#17816,.F.);
#24322=ORIENTED_EDGE('',*,*,#17996,.T.);
#24323=ORIENTED_EDGE('',*,*,#17997,.T.);
#24324=ORIENTED_EDGE('',*,*,#17998,.T.);
#24325=ORIENTED_EDGE('',*,*,#17996,.F.);
#24326=ORIENTED_EDGE('',*,*,#17815,.F.);
#24327=ORIENTED_EDGE('',*,*,#17999,.T.);
#24328=ORIENTED_EDGE('',*,*,#17999,.F.);
#24329=ORIENTED_EDGE('',*,*,#17814,.F.);
#24330=ORIENTED_EDGE('',*,*,#17984,.T.);
#24331=ORIENTED_EDGE('',*,*,#18000,.T.);
#24332=ORIENTED_EDGE('',*,*,#17829,.T.);
#24333=ORIENTED_EDGE('',*,*,#18001,.T.);
#24334=ORIENTED_EDGE('',*,*,#18002,.F.);
#24335=ORIENTED_EDGE('',*,*,#18003,.T.);
#24336=ORIENTED_EDGE('',*,*,#18004,.F.);
#24337=ORIENTED_EDGE('',*,*,#18001,.F.);
#24338=ORIENTED_EDGE('',*,*,#17828,.T.);
#24339=ORIENTED_EDGE('',*,*,#18005,.T.);
#24340=ORIENTED_EDGE('',*,*,#17827,.T.);
#24341=ORIENTED_EDGE('',*,*,#18006,.T.);
#24342=ORIENTED_EDGE('',*,*,#18007,.F.);
#24343=ORIENTED_EDGE('',*,*,#18008,.F.);
#24344=ORIENTED_EDGE('',*,*,#18005,.F.);
#24345=ORIENTED_EDGE('',*,*,#18006,.F.);
#24346=ORIENTED_EDGE('',*,*,#17826,.F.);
#24347=ORIENTED_EDGE('',*,*,#18009,.T.);
#24348=ORIENTED_EDGE('',*,*,#18010,.T.);
#24349=ORIENTED_EDGE('',*,*,#18011,.T.);
#24350=ORIENTED_EDGE('',*,*,#18012,.T.);
#24351=ORIENTED_EDGE('',*,*,#18013,.F.);
#24352=ORIENTED_EDGE('',*,*,#18009,.F.);
#24353=ORIENTED_EDGE('',*,*,#17825,.F.);
#24354=ORIENTED_EDGE('',*,*,#18014,.F.);
#24355=ORIENTED_EDGE('',*,*,#18012,.F.);
#24356=ORIENTED_EDGE('',*,*,#17824,.T.);
#24357=ORIENTED_EDGE('',*,*,#18015,.F.);
#24358=ORIENTED_EDGE('',*,*,#18016,.F.);
#24359=ORIENTED_EDGE('',*,*,#18017,.F.);
#24360=ORIENTED_EDGE('',*,*,#18018,.F.);
#24361=ORIENTED_EDGE('',*,*,#18015,.T.);
#24362=ORIENTED_EDGE('',*,*,#17823,.F.);
#24363=ORIENTED_EDGE('',*,*,#18003,.F.);
#24364=ORIENTED_EDGE('',*,*,#18019,.F.);
#24365=ORIENTED_EDGE('',*,*,#18020,.T.);
#24366=ORIENTED_EDGE('',*,*,#18021,.F.);
#24367=ORIENTED_EDGE('',*,*,#18022,.F.);
#24368=ORIENTED_EDGE('',*,*,#18020,.F.);
#24369=ORIENTED_EDGE('',*,*,#17836,.T.);
#24370=ORIENTED_EDGE('',*,*,#17835,.T.);
#24371=ORIENTED_EDGE('',*,*,#17841,.T.);
#24372=ORIENTED_EDGE('',*,*,#17959,.F.);
#24373=ORIENTED_EDGE('',*,*,#17960,.T.);
#24374=ORIENTED_EDGE('',*,*,#17862,.F.);
#24375=ORIENTED_EDGE('',*,*,#17864,.T.);
#24376=ORIENTED_EDGE('',*,*,#17865,.T.);
#24377=ORIENTED_EDGE('',*,*,#17874,.F.);
#24378=ORIENTED_EDGE('',*,*,#18023,.T.);
#24379=ORIENTED_EDGE('',*,*,#17858,.F.);
#24380=ORIENTED_EDGE('',*,*,#18024,.T.);
#24381=ORIENTED_EDGE('',*,*,#18025,.T.);
#24382=ORIENTED_EDGE('',*,*,#17859,.T.);
#24383=ORIENTED_EDGE('',*,*,#18023,.F.);
#24384=ORIENTED_EDGE('',*,*,#17873,.F.);
#24385=ORIENTED_EDGE('',*,*,#18026,.F.);
#24386=ORIENTED_EDGE('',*,*,#18027,.T.);
#24387=ORIENTED_EDGE('',*,*,#18028,.F.);
#24388=ORIENTED_EDGE('',*,*,#18029,.F.);
#24389=ORIENTED_EDGE('',*,*,#17846,.T.);
#24390=ORIENTED_EDGE('',*,*,#18030,.F.);
#24391=ORIENTED_EDGE('',*,*,#18031,.F.);
#24392=ORIENTED_EDGE('',*,*,#18032,.F.);
#24393=ORIENTED_EDGE('',*,*,#18029,.T.);
#24394=ORIENTED_EDGE('',*,*,#18033,.F.);
#24395=ORIENTED_EDGE('',*,*,#18034,.F.);
#24396=ORIENTED_EDGE('',*,*,#17847,.F.);
#24397=ORIENTED_EDGE('',*,*,#18035,.T.);
#24398=ORIENTED_EDGE('',*,*,#18036,.T.);
#24399=ORIENTED_EDGE('',*,*,#18037,.T.);
#24400=ORIENTED_EDGE('',*,*,#17848,.F.);
#24401=ORIENTED_EDGE('',*,*,#18034,.T.);
#24402=ORIENTED_EDGE('',*,*,#18038,.T.);
#24403=ORIENTED_EDGE('',*,*,#18039,.F.);
#24404=ORIENTED_EDGE('',*,*,#18040,.T.);
#24405=ORIENTED_EDGE('',*,*,#18041,.T.);
#24406=ORIENTED_EDGE('',*,*,#17907,.T.);
#24407=ORIENTED_EDGE('',*,*,#18042,.F.);
#24408=ORIENTED_EDGE('',*,*,#17854,.F.);
#24409=ORIENTED_EDGE('',*,*,#18043,.F.);
#24410=ORIENTED_EDGE('',*,*,#17855,.F.);
#24411=ORIENTED_EDGE('',*,*,#18042,.T.);
#24412=ORIENTED_EDGE('',*,*,#17906,.F.);
#24413=ORIENTED_EDGE('',*,*,#17914,.T.);
#24414=ORIENTED_EDGE('',*,*,#17915,.T.);
#24415=ORIENTED_EDGE('',*,*,#17917,.F.);
#24416=ORIENTED_EDGE('',*,*,#17894,.F.);
#24417=ORIENTED_EDGE('',*,*,#18044,.F.);
#24418=ORIENTED_EDGE('',*,*,#17868,.F.);
#24419=ORIENTED_EDGE('',*,*,#17876,.F.);
#24420=ORIENTED_EDGE('',*,*,#17878,.F.);
#24421=ORIENTED_EDGE('',*,*,#17880,.F.);
#24422=ORIENTED_EDGE('',*,*,#17869,.T.);
#24423=ORIENTED_EDGE('',*,*,#18044,.T.);
#24424=ORIENTED_EDGE('',*,*,#17893,.F.);
#24425=ORIENTED_EDGE('',*,*,#18045,.F.);
#24426=ORIENTED_EDGE('',*,*,#18046,.F.);
#24427=ORIENTED_EDGE('',*,*,#17900,.F.);
#24428=ORIENTED_EDGE('',*,*,#17902,.F.);
#24429=ORIENTED_EDGE('',*,*,#17903,.F.);
#24430=ORIENTED_EDGE('',*,*,#17912,.F.);
#24431=ORIENTED_EDGE('',*,*,#18047,.F.);
#24432=ORIENTED_EDGE('',*,*,#17896,.F.);
#24433=ORIENTED_EDGE('',*,*,#18048,.T.);
#24434=ORIENTED_EDGE('',*,*,#17897,.T.);
#24435=ORIENTED_EDGE('',*,*,#18047,.T.);
#24436=ORIENTED_EDGE('',*,*,#17911,.F.);
#24437=ORIENTED_EDGE('',*,*,#18049,.F.);
#24438=ORIENTED_EDGE('',*,*,#18050,.T.);
#24439=ORIENTED_EDGE('',*,*,#18051,.F.);
#24440=ORIENTED_EDGE('',*,*,#18052,.T.);
#24441=ORIENTED_EDGE('',*,*,#18053,.F.);
#24442=ORIENTED_EDGE('',*,*,#18054,.T.);
#24443=ORIENTED_EDGE('',*,*,#18055,.F.);
#24444=ORIENTED_EDGE('',*,*,#18056,.F.);
#24445=ORIENTED_EDGE('',*,*,#17885,.T.);
#24446=ORIENTED_EDGE('',*,*,#17886,.T.);
#24447=ORIENTED_EDGE('',*,*,#18056,.T.);
#24448=ORIENTED_EDGE('',*,*,#18057,.T.);
#24449=ORIENTED_EDGE('',*,*,#18058,.F.);
#24450=ORIENTED_EDGE('',*,*,#17887,.F.);
#24451=ORIENTED_EDGE('',*,*,#18058,.T.);
#24452=ORIENTED_EDGE('',*,*,#18059,.T.);
#24453=ORIENTED_EDGE('',*,*,#18060,.F.);
#24454=ORIENTED_EDGE('',*,*,#18061,.T.);
#24455=ORIENTED_EDGE('',*,*,#18062,.F.);
#24456=ORIENTED_EDGE('',*,*,#18063,.T.);
#24457=ORIENTED_EDGE('',*,*,#18064,.F.);
#24458=ORIENTED_EDGE('',*,*,#18065,.T.);
#24459=ORIENTED_EDGE('',*,*,#17909,.F.);
#24460=ORIENTED_EDGE('',*,*,#18066,.F.);
#24461=ORIENTED_EDGE('',*,*,#18067,.T.);
#24462=ORIENTED_EDGE('',*,*,#18049,.T.);
#24463=ORIENTED_EDGE('',*,*,#17910,.T.);
#24464=ORIENTED_EDGE('',*,*,#18065,.F.);
#24465=ORIENTED_EDGE('',*,*,#18068,.T.);
#24466=ORIENTED_EDGE('',*,*,#18041,.F.);
#24467=ORIENTED_EDGE('',*,*,#18069,.F.);
#24468=ORIENTED_EDGE('',*,*,#18066,.T.);
#24469=ORIENTED_EDGE('',*,*,#17908,.T.);
#24470=ORIENTED_EDGE('',*,*,#17938,.T.);
#24471=ORIENTED_EDGE('',*,*,#17922,.F.);
#24472=ORIENTED_EDGE('',*,*,#18070,.F.);
#24473=ORIENTED_EDGE('',*,*,#18071,.T.);
#24474=ORIENTED_EDGE('',*,*,#17924,.T.);
#24475=ORIENTED_EDGE('',*,*,#17930,.T.);
#24476=ORIENTED_EDGE('',*,*,#18072,.F.);
#24477=ORIENTED_EDGE('',*,*,#18073,.T.);
#24478=ORIENTED_EDGE('',*,*,#18074,.T.);
#24479=ORIENTED_EDGE('',*,*,#17933,.T.);
#24480=ORIENTED_EDGE('',*,*,#17939,.T.);
#24481=ORIENTED_EDGE('',*,*,#18071,.F.);
#24482=ORIENTED_EDGE('',*,*,#18070,.T.);
#24483=ORIENTED_EDGE('',*,*,#17921,.F.);
#24484=ORIENTED_EDGE('',*,*,#18075,.F.);
#24485=ORIENTED_EDGE('',*,*,#18076,.F.);
#24486=ORIENTED_EDGE('',*,*,#17925,.T.);
#24487=ORIENTED_EDGE('',*,*,#18076,.T.);
#24488=ORIENTED_EDGE('',*,*,#18075,.T.);
#24489=ORIENTED_EDGE('',*,*,#17920,.F.);
#24490=ORIENTED_EDGE('',*,*,#17934,.T.);
#24491=ORIENTED_EDGE('',*,*,#18074,.F.);
#24492=ORIENTED_EDGE('',*,*,#18073,.F.);
#24493=ORIENTED_EDGE('',*,*,#18072,.T.);
#24494=ORIENTED_EDGE('',*,*,#17929,.T.);
#24495=ORIENTED_EDGE('',*,*,#18077,.T.);
#24496=ORIENTED_EDGE('',*,*,#18078,.F.);
#24497=ORIENTED_EDGE('',*,*,#17927,.T.);
#24498=ORIENTED_EDGE('',*,*,#17932,.F.);
#24499=ORIENTED_EDGE('',*,*,#17936,.T.);
#24500=ORIENTED_EDGE('',*,*,#18079,.T.);
#24501=ORIENTED_EDGE('',*,*,#18080,.T.);
#24502=ORIENTED_EDGE('',*,*,#17928,.T.);
#24503=ORIENTED_EDGE('',*,*,#18078,.T.);
#24504=ORIENTED_EDGE('',*,*,#18077,.F.);
#24505=ORIENTED_EDGE('',*,*,#18080,.F.);
#24506=ORIENTED_EDGE('',*,*,#18079,.F.);
#24507=ORIENTED_EDGE('',*,*,#17935,.T.);
#24508=ORIENTED_EDGE('',*,*,#18081,.F.);
#24509=ORIENTED_EDGE('',*,*,#17955,.T.);
#24510=ORIENTED_EDGE('',*,*,#17957,.T.);
#24511=ORIENTED_EDGE('',*,*,#17942,.F.);
#24512=ORIENTED_EDGE('',*,*,#18082,.T.);
#24513=ORIENTED_EDGE('',*,*,#17946,.T.);
#24514=ORIENTED_EDGE('',*,*,#18083,.F.);
#24515=ORIENTED_EDGE('',*,*,#17950,.F.);
#24516=ORIENTED_EDGE('',*,*,#17953,.T.);
#24517=ORIENTED_EDGE('',*,*,#17956,.T.);
#24518=ORIENTED_EDGE('',*,*,#18081,.T.);
#24519=ORIENTED_EDGE('',*,*,#18082,.F.);
#24520=ORIENTED_EDGE('',*,*,#17941,.F.);
#24521=ORIENTED_EDGE('',*,*,#17945,.T.);
#24522=ORIENTED_EDGE('',*,*,#17948,.F.);
#24523=ORIENTED_EDGE('',*,*,#17951,.F.);
#24524=ORIENTED_EDGE('',*,*,#18083,.T.);
#24525=ORIENTED_EDGE('',*,*,#17981,.F.);
#24526=ORIENTED_EDGE('',*,*,#17964,.F.);
#24527=ORIENTED_EDGE('',*,*,#17967,.F.);
#24528=ORIENTED_EDGE('',*,*,#17970,.F.);
#24529=ORIENTED_EDGE('',*,*,#18084,.T.);
#24530=ORIENTED_EDGE('',*,*,#18085,.F.);
#24531=ORIENTED_EDGE('',*,*,#17982,.F.);
#24532=ORIENTED_EDGE('',*,*,#18085,.T.);
#24533=ORIENTED_EDGE('',*,*,#18084,.F.);
#24534=ORIENTED_EDGE('',*,*,#17969,.F.);
#24535=ORIENTED_EDGE('',*,*,#17973,.F.);
#24536=ORIENTED_EDGE('',*,*,#18086,.T.);
#24537=ORIENTED_EDGE('',*,*,#17983,.F.);
#24538=ORIENTED_EDGE('',*,*,#18086,.F.);
#24539=ORIENTED_EDGE('',*,*,#17972,.F.);
#24540=ORIENTED_EDGE('',*,*,#17975,.F.);
#24541=ORIENTED_EDGE('',*,*,#17976,.F.);
#24542=ORIENTED_EDGE('',*,*,#17980,.F.);
#24543=ORIENTED_EDGE('',*,*,#17978,.F.);
#24544=ORIENTED_EDGE('',*,*,#18087,.T.);
#24545=ORIENTED_EDGE('',*,*,#18088,.T.);
#24546=ORIENTED_EDGE('',*,*,#18087,.F.);
#24547=ORIENTED_EDGE('',*,*,#17998,.F.);
#24548=ORIENTED_EDGE('',*,*,#18000,.F.);
#24549=ORIENTED_EDGE('',*,*,#17985,.F.);
#24550=ORIENTED_EDGE('',*,*,#17763,.T.);
#24551=ORIENTED_EDGE('',*,*,#17987,.T.);
#24552=ORIENTED_EDGE('',*,*,#17988,.F.);
#24553=ORIENTED_EDGE('',*,*,#17990,.T.);
#24554=ORIENTED_EDGE('',*,*,#17992,.F.);
#24555=ORIENTED_EDGE('',*,*,#17994,.F.);
#24556=ORIENTED_EDGE('',*,*,#17997,.F.);
#24557=ORIENTED_EDGE('',*,*,#18089,.F.);
#24558=ORIENTED_EDGE('',*,*,#18090,.F.);
#24559=ORIENTED_EDGE('',*,*,#18091,.F.);
#24560=ORIENTED_EDGE('',*,*,#18092,.T.);
#24561=ORIENTED_EDGE('',*,*,#18093,.F.);
#24562=ORIENTED_EDGE('',*,*,#18094,.F.);
#24563=ORIENTED_EDGE('',*,*,#18095,.F.);
#24564=ORIENTED_EDGE('',*,*,#18096,.T.);
#24565=ORIENTED_EDGE('',*,*,#18097,.T.);
#24566=ORIENTED_EDGE('',*,*,#18098,.T.);
#24567=ORIENTED_EDGE('',*,*,#18099,.F.);
#24568=ORIENTED_EDGE('',*,*,#18016,.T.);
#24569=ORIENTED_EDGE('',*,*,#18019,.T.);
#24570=ORIENTED_EDGE('',*,*,#18002,.T.);
#24571=ORIENTED_EDGE('',*,*,#18004,.T.);
#24572=ORIENTED_EDGE('',*,*,#18008,.T.);
#24573=ORIENTED_EDGE('',*,*,#18100,.F.);
#24574=ORIENTED_EDGE('',*,*,#18017,.T.);
#24575=ORIENTED_EDGE('',*,*,#18100,.T.);
#24576=ORIENTED_EDGE('',*,*,#18007,.T.);
#24577=ORIENTED_EDGE('',*,*,#18011,.F.);
#24578=ORIENTED_EDGE('',*,*,#18101,.T.);
#24579=ORIENTED_EDGE('',*,*,#18102,.T.);
#24580=ORIENTED_EDGE('',*,*,#18018,.T.);
#24581=ORIENTED_EDGE('',*,*,#18102,.F.);
#24582=ORIENTED_EDGE('',*,*,#18101,.F.);
#24583=ORIENTED_EDGE('',*,*,#18010,.F.);
#24584=ORIENTED_EDGE('',*,*,#18013,.T.);
#24585=ORIENTED_EDGE('',*,*,#18014,.T.);
#24586=ORIENTED_EDGE('',*,*,#18022,.T.);
#24587=ORIENTED_EDGE('',*,*,#18103,.T.);
#24588=ORIENTED_EDGE('',*,*,#18104,.F.);
#24589=ORIENTED_EDGE('',*,*,#18103,.F.);
#24590=ORIENTED_EDGE('',*,*,#18021,.T.);
#24591=ORIENTED_EDGE('',*,*,#18024,.F.);
#24592=ORIENTED_EDGE('',*,*,#17872,.T.);
#24593=ORIENTED_EDGE('',*,*,#18105,.T.);
#24594=ORIENTED_EDGE('',*,*,#18106,.T.);
#24595=ORIENTED_EDGE('',*,*,#18025,.F.);
#24596=ORIENTED_EDGE('',*,*,#18106,.F.);
#24597=ORIENTED_EDGE('',*,*,#18107,.F.);
#24598=ORIENTED_EDGE('',*,*,#18108,.F.);
#24599=ORIENTED_EDGE('',*,*,#18045,.T.);
#24600=ORIENTED_EDGE('',*,*,#18109,.T.);
#24601=ORIENTED_EDGE('',*,*,#18110,.F.);
#24602=ORIENTED_EDGE('',*,*,#18111,.T.);
#24603=ORIENTED_EDGE('',*,*,#18031,.T.);
#24604=ORIENTED_EDGE('',*,*,#18112,.T.);
#24605=ORIENTED_EDGE('',*,*,#18113,.T.);
#24606=ORIENTED_EDGE('',*,*,#18114,.F.);
#24607=ORIENTED_EDGE('',*,*,#18115,.T.);
#24608=ORIENTED_EDGE('',*,*,#18116,.T.);
#24609=ORIENTED_EDGE('',*,*,#18117,.T.);
#24610=ORIENTED_EDGE('',*,*,#18118,.T.);
#24611=ORIENTED_EDGE('',*,*,#18119,.F.);
#24612=ORIENTED_EDGE('',*,*,#18120,.T.);
#24613=ORIENTED_EDGE('',*,*,#18121,.F.);
#24614=ORIENTED_EDGE('',*,*,#18122,.T.);
#24615=ORIENTED_EDGE('',*,*,#18123,.T.);
#24616=ORIENTED_EDGE('',*,*,#18124,.T.);
#24617=ORIENTED_EDGE('',*,*,#18125,.T.);
#24618=ORIENTED_EDGE('',*,*,#18126,.F.);
#24619=ORIENTED_EDGE('',*,*,#18127,.F.);
#24620=ORIENTED_EDGE('',*,*,#18128,.T.);
#24621=ORIENTED_EDGE('',*,*,#18129,.T.);
#24622=ORIENTED_EDGE('',*,*,#18130,.T.);
#24623=ORIENTED_EDGE('',*,*,#18063,.F.);
#24624=ORIENTED_EDGE('',*,*,#18131,.T.);
#24625=ORIENTED_EDGE('',*,*,#18040,.F.);
#24626=ORIENTED_EDGE('',*,*,#18132,.F.);
#24627=ORIENTED_EDGE('',*,*,#18026,.T.);
#24628=ORIENTED_EDGE('',*,*,#18133,.T.);
#24629=ORIENTED_EDGE('',*,*,#18134,.T.);
#24630=ORIENTED_EDGE('',*,*,#18027,.F.);
#24631=ORIENTED_EDGE('',*,*,#18132,.T.);
#24632=ORIENTED_EDGE('',*,*,#18039,.T.);
#24633=ORIENTED_EDGE('',*,*,#18033,.T.);
#24634=ORIENTED_EDGE('',*,*,#18028,.T.);
#24635=ORIENTED_EDGE('',*,*,#18134,.F.);
#24636=ORIENTED_EDGE('',*,*,#18038,.F.);
#24637=ORIENTED_EDGE('',*,*,#18135,.T.);
#24638=ORIENTED_EDGE('',*,*,#18136,.F.);
#24639=ORIENTED_EDGE('',*,*,#18137,.F.);
#24640=ORIENTED_EDGE('',*,*,#18138,.T.);
#24641=ORIENTED_EDGE('',*,*,#18139,.F.);
#24642=ORIENTED_EDGE('',*,*,#18140,.F.);
#24643=ORIENTED_EDGE('',*,*,#18141,.T.);
#24644=ORIENTED_EDGE('',*,*,#18142,.T.);
#24645=ORIENTED_EDGE('',*,*,#18143,.F.);
#24646=ORIENTED_EDGE('',*,*,#18144,.F.);
#24647=ORIENTED_EDGE('',*,*,#18145,.T.);
#24648=ORIENTED_EDGE('',*,*,#18146,.F.);
#24649=ORIENTED_EDGE('',*,*,#18147,.F.);
#24650=ORIENTED_EDGE('',*,*,#18035,.F.);
#24651=ORIENTED_EDGE('',*,*,#18133,.F.);
#24652=ORIENTED_EDGE('',*,*,#18032,.T.);
#24653=ORIENTED_EDGE('',*,*,#18111,.F.);
#24654=ORIENTED_EDGE('',*,*,#18148,.F.);
#24655=ORIENTED_EDGE('',*,*,#18149,.F.);
#24656=ORIENTED_EDGE('',*,*,#18150,.T.);
#24657=ORIENTED_EDGE('',*,*,#18151,.F.);
#24658=ORIENTED_EDGE('',*,*,#18152,.T.);
#24659=ORIENTED_EDGE('',*,*,#18153,.T.);
#24660=ORIENTED_EDGE('',*,*,#18113,.F.);
#24661=ORIENTED_EDGE('',*,*,#18154,.T.);
#24662=ORIENTED_EDGE('',*,*,#18155,.F.);
#24663=ORIENTED_EDGE('',*,*,#18156,.F.);
#24664=ORIENTED_EDGE('',*,*,#18157,.T.);
#24665=ORIENTED_EDGE('',*,*,#18158,.F.);
#24666=ORIENTED_EDGE('',*,*,#18159,.T.);
#24667=ORIENTED_EDGE('',*,*,#18120,.F.);
#24668=ORIENTED_EDGE('',*,*,#18160,.T.);
#24669=ORIENTED_EDGE('',*,*,#18161,.T.);
#24670=ORIENTED_EDGE('',*,*,#18162,.T.);
#24671=ORIENTED_EDGE('',*,*,#18163,.F.);
#24672=ORIENTED_EDGE('',*,*,#18164,.T.);
#24673=ORIENTED_EDGE('',*,*,#18165,.F.);
#24674=ORIENTED_EDGE('',*,*,#18166,.T.);
#24675=ORIENTED_EDGE('',*,*,#18167,.T.);
#24676=ORIENTED_EDGE('',*,*,#18036,.F.);
#24677=ORIENTED_EDGE('',*,*,#18147,.T.);
#24678=ORIENTED_EDGE('',*,*,#18140,.T.);
#24679=ORIENTED_EDGE('',*,*,#18168,.F.);
#24680=ORIENTED_EDGE('',*,*,#18169,.T.);
#24681=ORIENTED_EDGE('',*,*,#18170,.T.);
#24682=ORIENTED_EDGE('',*,*,#18171,.F.);
#24683=ORIENTED_EDGE('',*,*,#18139,.T.);
#24684=ORIENTED_EDGE('',*,*,#18172,.T.);
#24685=ORIENTED_EDGE('',*,*,#18173,.T.);
#24686=ORIENTED_EDGE('',*,*,#18174,.T.);
#24687=ORIENTED_EDGE('',*,*,#18175,.T.);
#24688=ORIENTED_EDGE('',*,*,#18176,.F.);
#24689=ORIENTED_EDGE('',*,*,#18177,.T.);
#24690=ORIENTED_EDGE('',*,*,#18178,.T.);
#24691=ORIENTED_EDGE('',*,*,#18179,.F.);
#24692=ORIENTED_EDGE('',*,*,#18180,.F.);
#24693=ORIENTED_EDGE('',*,*,#18181,.T.);
#24694=ORIENTED_EDGE('',*,*,#18182,.F.);
#24695=ORIENTED_EDGE('',*,*,#18183,.T.);
#24696=ORIENTED_EDGE('',*,*,#18051,.T.);
#24697=ORIENTED_EDGE('',*,*,#18184,.T.);
#24698=ORIENTED_EDGE('',*,*,#18185,.T.);
#24699=ORIENTED_EDGE('',*,*,#18048,.F.);
#24700=ORIENTED_EDGE('',*,*,#18068,.F.);
#24701=ORIENTED_EDGE('',*,*,#18067,.F.);
#24702=ORIENTED_EDGE('',*,*,#18069,.T.);
#24703=ORIENTED_EDGE('',*,*,#18043,.T.);
#24704=ORIENTED_EDGE('',*,*,#18107,.T.);
#24705=ORIENTED_EDGE('',*,*,#18105,.F.);
#24706=ORIENTED_EDGE('',*,*,#17871,.F.);
#24707=ORIENTED_EDGE('',*,*,#18186,.T.);
#24708=ORIENTED_EDGE('',*,*,#18186,.F.);
#24709=ORIENTED_EDGE('',*,*,#17870,.T.);
#24710=ORIENTED_EDGE('',*,*,#18046,.T.);
#24711=ORIENTED_EDGE('',*,*,#18108,.T.);
#24712=ORIENTED_EDGE('',*,*,#18055,.T.);
#24713=ORIENTED_EDGE('',*,*,#18187,.T.);
#24714=ORIENTED_EDGE('',*,*,#18059,.F.);
#24715=ORIENTED_EDGE('',*,*,#18057,.F.);
#24716=ORIENTED_EDGE('',*,*,#18054,.F.);
#24717=ORIENTED_EDGE('',*,*,#18188,.F.);
#24718=ORIENTED_EDGE('',*,*,#18060,.T.);
#24719=ORIENTED_EDGE('',*,*,#18187,.F.);
#24720=ORIENTED_EDGE('',*,*,#18189,.F.);
#24721=ORIENTED_EDGE('',*,*,#18061,.F.);
#24722=ORIENTED_EDGE('',*,*,#18188,.T.);
#24723=ORIENTED_EDGE('',*,*,#18053,.T.);
#24724=ORIENTED_EDGE('',*,*,#18177,.F.);
#24725=ORIENTED_EDGE('',*,*,#18190,.F.);
#24726=ORIENTED_EDGE('',*,*,#18191,.F.);
#24727=ORIENTED_EDGE('',*,*,#18192,.T.);
#24728=ORIENTED_EDGE('',*,*,#18193,.F.);
#24729=ORIENTED_EDGE('',*,*,#18194,.F.);
#24730=ORIENTED_EDGE('',*,*,#18195,.T.);
#24731=ORIENTED_EDGE('',*,*,#18178,.F.);
#24732=ORIENTED_EDGE('',*,*,#18196,.T.);
#24733=ORIENTED_EDGE('',*,*,#18197,.T.);
#24734=ORIENTED_EDGE('',*,*,#18198,.T.);
#24735=ORIENTED_EDGE('',*,*,#18125,.F.);
#24736=ORIENTED_EDGE('',*,*,#18199,.T.);
#24737=ORIENTED_EDGE('',*,*,#18200,.F.);
#24738=ORIENTED_EDGE('',*,*,#18201,.F.);
#24739=ORIENTED_EDGE('',*,*,#18202,.F.);
#24740=ORIENTED_EDGE('',*,*,#18203,.F.);
#24741=ORIENTED_EDGE('',*,*,#18204,.T.);
#24742=ORIENTED_EDGE('',*,*,#18131,.F.);
#24743=ORIENTED_EDGE('',*,*,#18062,.T.);
#24744=ORIENTED_EDGE('',*,*,#18189,.T.);
#24745=ORIENTED_EDGE('',*,*,#18052,.F.);
#24746=ORIENTED_EDGE('',*,*,#18183,.F.);
#24747=ORIENTED_EDGE('',*,*,#18205,.T.);
#24748=ORIENTED_EDGE('',*,*,#18206,.T.);
#24749=ORIENTED_EDGE('',*,*,#18207,.F.);
#24750=ORIENTED_EDGE('',*,*,#18208,.T.);
#24751=ORIENTED_EDGE('',*,*,#18209,.F.);
#24752=ORIENTED_EDGE('',*,*,#18210,.F.);
#24753=ORIENTED_EDGE('',*,*,#18211,.F.);
#24754=ORIENTED_EDGE('',*,*,#18122,.F.);
#24755=ORIENTED_EDGE('',*,*,#18212,.F.);
#24756=ORIENTED_EDGE('',*,*,#18213,.F.);
#24757=ORIENTED_EDGE('',*,*,#18214,.F.);
#24758=ORIENTED_EDGE('',*,*,#18215,.F.);
#24759=ORIENTED_EDGE('',*,*,#18216,.T.);
#24760=ORIENTED_EDGE('',*,*,#18217,.T.);
#24761=ORIENTED_EDGE('',*,*,#18088,.F.);
#24762=ORIENTED_EDGE('',*,*,#18218,.T.);
#24763=ORIENTED_EDGE('',*,*,#18089,.T.);
#24764=ORIENTED_EDGE('',*,*,#18219,.F.);
#24765=ORIENTED_EDGE('',*,*,#18220,.T.);
#24766=ORIENTED_EDGE('',*,*,#18221,.T.);
#24767=ORIENTED_EDGE('',*,*,#18221,.F.);
#24768=ORIENTED_EDGE('',*,*,#18222,.T.);
#24769=ORIENTED_EDGE('',*,*,#18223,.T.);
#24770=ORIENTED_EDGE('',*,*,#18090,.T.);
#24771=ORIENTED_EDGE('',*,*,#18091,.T.);
#24772=ORIENTED_EDGE('',*,*,#18223,.F.);
#24773=ORIENTED_EDGE('',*,*,#18224,.T.);
#24774=ORIENTED_EDGE('',*,*,#18225,.T.);
#24775=ORIENTED_EDGE('',*,*,#18226,.T.);
#24776=ORIENTED_EDGE('',*,*,#18092,.F.);
#24777=ORIENTED_EDGE('',*,*,#18225,.F.);
#24778=ORIENTED_EDGE('',*,*,#18227,.F.);
#24779=ORIENTED_EDGE('',*,*,#18093,.T.);
#24780=ORIENTED_EDGE('',*,*,#18226,.F.);
#24781=ORIENTED_EDGE('',*,*,#18228,.T.);
#24782=ORIENTED_EDGE('',*,*,#18229,.T.);
#24783=ORIENTED_EDGE('',*,*,#18229,.F.);
#24784=ORIENTED_EDGE('',*,*,#18230,.F.);
#24785=ORIENTED_EDGE('',*,*,#18231,.T.);
#24786=ORIENTED_EDGE('',*,*,#18094,.T.);
#24787=ORIENTED_EDGE('',*,*,#18231,.F.);
#24788=ORIENTED_EDGE('',*,*,#18232,.F.);
#24789=ORIENTED_EDGE('',*,*,#18233,.T.);
#24790=ORIENTED_EDGE('',*,*,#18095,.T.);
#24791=ORIENTED_EDGE('',*,*,#18233,.F.);
#24792=ORIENTED_EDGE('',*,*,#18234,.T.);
#24793=ORIENTED_EDGE('',*,*,#18235,.T.);
#24794=ORIENTED_EDGE('',*,*,#18096,.F.);
#24795=ORIENTED_EDGE('',*,*,#18097,.F.);
#24796=ORIENTED_EDGE('',*,*,#18235,.F.);
#24797=ORIENTED_EDGE('',*,*,#18236,.T.);
#24798=ORIENTED_EDGE('',*,*,#18219,.T.);
#24799=ORIENTED_EDGE('',*,*,#18098,.F.);
#24800=ORIENTED_EDGE('',*,*,#18237,.T.);
#24801=ORIENTED_EDGE('',*,*,#18238,.T.);
#24802=ORIENTED_EDGE('',*,*,#18237,.F.);
#24803=ORIENTED_EDGE('',*,*,#18239,.F.);
#24804=ORIENTED_EDGE('',*,*,#18240,.T.);
#24805=ORIENTED_EDGE('',*,*,#18099,.T.);
#24806=ORIENTED_EDGE('',*,*,#18240,.F.);
#24807=ORIENTED_EDGE('',*,*,#18104,.T.);
#24808=ORIENTED_EDGE('',*,*,#18241,.F.);
#24809=ORIENTED_EDGE('',*,*,#18242,.T.);
#24810=ORIENTED_EDGE('',*,*,#18243,.F.);
#24811=ORIENTED_EDGE('',*,*,#18161,.F.);
#24812=ORIENTED_EDGE('',*,*,#18244,.T.);
#24813=ORIENTED_EDGE('',*,*,#18162,.F.);
#24814=ORIENTED_EDGE('',*,*,#18243,.T.);
#24815=ORIENTED_EDGE('',*,*,#18245,.F.);
#24816=ORIENTED_EDGE('',*,*,#18246,.F.);
#24817=ORIENTED_EDGE('',*,*,#18247,.F.);
#24818=ORIENTED_EDGE('',*,*,#18163,.T.);
#24819=ORIENTED_EDGE('',*,*,#18246,.T.);
#24820=ORIENTED_EDGE('',*,*,#18248,.F.);
#24821=ORIENTED_EDGE('',*,*,#18164,.F.);
#24822=ORIENTED_EDGE('',*,*,#18247,.T.);
#24823=ORIENTED_EDGE('',*,*,#18249,.T.);
#24824=ORIENTED_EDGE('',*,*,#18250,.F.);
#24825=ORIENTED_EDGE('',*,*,#18165,.T.);
#24826=ORIENTED_EDGE('',*,*,#18250,.T.);
#24827=ORIENTED_EDGE('',*,*,#18251,.F.);
#24828=ORIENTED_EDGE('',*,*,#18252,.F.);
#24829=ORIENTED_EDGE('',*,*,#18143,.T.);
#24830=ORIENTED_EDGE('',*,*,#18253,.T.);
#24831=ORIENTED_EDGE('',*,*,#18254,.F.);
#24832=ORIENTED_EDGE('',*,*,#18255,.F.);
#24833=ORIENTED_EDGE('',*,*,#18256,.F.);
#24834=ORIENTED_EDGE('',*,*,#18257,.F.);
#24835=ORIENTED_EDGE('',*,*,#18136,.T.);
#24836=ORIENTED_EDGE('',*,*,#18258,.T.);
#24837=ORIENTED_EDGE('',*,*,#18137,.T.);
#24838=ORIENTED_EDGE('',*,*,#18257,.T.);
#24839=ORIENTED_EDGE('',*,*,#18259,.T.);
#24840=ORIENTED_EDGE('',*,*,#18260,.F.);
#24841=ORIENTED_EDGE('',*,*,#18261,.T.);
#24842=ORIENTED_EDGE('',*,*,#18262,.F.);
#24843=ORIENTED_EDGE('',*,*,#18191,.T.);
#24844=ORIENTED_EDGE('',*,*,#18263,.T.);
#24845=ORIENTED_EDGE('',*,*,#18264,.F.);
#24846=ORIENTED_EDGE('',*,*,#18192,.F.);
#24847=ORIENTED_EDGE('',*,*,#18262,.T.);
#24848=ORIENTED_EDGE('',*,*,#18265,.T.);
#24849=ORIENTED_EDGE('',*,*,#18266,.F.);
#24850=ORIENTED_EDGE('',*,*,#18198,.F.);
#24851=ORIENTED_EDGE('',*,*,#18267,.T.);
#24852=ORIENTED_EDGE('',*,*,#18268,.T.);
#24853=ORIENTED_EDGE('',*,*,#18269,.T.);
#24854=ORIENTED_EDGE('',*,*,#18270,.T.);
#24855=ORIENTED_EDGE('',*,*,#18271,.F.);
#24856=ORIENTED_EDGE('',*,*,#18206,.F.);
#24857=ORIENTED_EDGE('',*,*,#18272,.F.);
#24858=ORIENTED_EDGE('',*,*,#18207,.T.);
#24859=ORIENTED_EDGE('',*,*,#18271,.T.);
#24860=ORIENTED_EDGE('',*,*,#18273,.F.);
#24861=ORIENTED_EDGE('',*,*,#18208,.F.);
#24862=ORIENTED_EDGE('',*,*,#18272,.T.);
#24863=ORIENTED_EDGE('',*,*,#18274,.T.);
#24864=ORIENTED_EDGE('',*,*,#18275,.T.);
#24865=ORIENTED_EDGE('',*,*,#18276,.F.);
#24866=ORIENTED_EDGE('',*,*,#18277,.T.);
#24867=ORIENTED_EDGE('',*,*,#18209,.T.);
#24868=ORIENTED_EDGE('',*,*,#18275,.F.);
#24869=ORIENTED_EDGE('',*,*,#18210,.T.);
#24870=ORIENTED_EDGE('',*,*,#18277,.F.);
#24871=ORIENTED_EDGE('',*,*,#18278,.F.);
#24872=ORIENTED_EDGE('',*,*,#18279,.F.);
#24873=ORIENTED_EDGE('',*,*,#18280,.F.);
#24874=ORIENTED_EDGE('',*,*,#18281,.T.);
#24875=ORIENTED_EDGE('',*,*,#18218,.F.);
#24876=ORIENTED_EDGE('',*,*,#18281,.F.);
#24877=ORIENTED_EDGE('',*,*,#18236,.F.);
#24878=ORIENTED_EDGE('',*,*,#18234,.F.);
#24879=ORIENTED_EDGE('',*,*,#18232,.T.);
#24880=ORIENTED_EDGE('',*,*,#18230,.T.);
#24881=ORIENTED_EDGE('',*,*,#18228,.F.);
#24882=ORIENTED_EDGE('',*,*,#18227,.T.);
#24883=ORIENTED_EDGE('',*,*,#18224,.F.);
#24884=ORIENTED_EDGE('',*,*,#18222,.F.);
#24885=ORIENTED_EDGE('',*,*,#18220,.F.);
#24886=ORIENTED_EDGE('',*,*,#18282,.T.);
#24887=ORIENTED_EDGE('',*,*,#17758,.F.);
#24888=ORIENTED_EDGE('',*,*,#18283,.F.);
#24889=ORIENTED_EDGE('',*,*,#18284,.F.);
#24890=ORIENTED_EDGE('',*,*,#18285,.T.);
#24891=ORIENTED_EDGE('',*,*,#18286,.T.);
#24892=ORIENTED_EDGE('',*,*,#18238,.F.);
#24893=ORIENTED_EDGE('',*,*,#18287,.T.);
#24894=ORIENTED_EDGE('',*,*,#18239,.T.);
#24895=ORIENTED_EDGE('',*,*,#18288,.F.);
#24896=ORIENTED_EDGE('',*,*,#18241,.T.);
#24897=ORIENTED_EDGE('',*,*,#18289,.T.);
#24898=ORIENTED_EDGE('',*,*,#18290,.T.);
#24899=ORIENTED_EDGE('',*,*,#18289,.F.);
#24900=ORIENTED_EDGE('',*,*,#18280,.T.);
#24901=ORIENTED_EDGE('',*,*,#18291,.T.);
#24902=ORIENTED_EDGE('',*,*,#18292,.T.);
#24903=ORIENTED_EDGE('',*,*,#18293,.T.);
#24904=ORIENTED_EDGE('',*,*,#17759,.F.);
#24905=ORIENTED_EDGE('',*,*,#18282,.F.);
#24906=ORIENTED_EDGE('',*,*,#18283,.T.);
#24907=ORIENTED_EDGE('',*,*,#17762,.T.);
#24908=ORIENTED_EDGE('',*,*,#18294,.F.);
#24909=ORIENTED_EDGE('',*,*,#18295,.F.);
#24910=ORIENTED_EDGE('',*,*,#18296,.F.);
#24911=ORIENTED_EDGE('',*,*,#18297,.F.);
#24912=ORIENTED_EDGE('',*,*,#18284,.T.);
#24913=ORIENTED_EDGE('',*,*,#18297,.T.);
#24914=ORIENTED_EDGE('',*,*,#18298,.F.);
#24915=ORIENTED_EDGE('',*,*,#18299,.F.);
#24916=ORIENTED_EDGE('',*,*,#18300,.F.);
#24917=ORIENTED_EDGE('',*,*,#18300,.T.);
#24918=ORIENTED_EDGE('',*,*,#18301,.T.);
#24919=ORIENTED_EDGE('',*,*,#18302,.T.);
#24920=ORIENTED_EDGE('',*,*,#18303,.F.);
#24921=ORIENTED_EDGE('',*,*,#18285,.F.);
#24922=ORIENTED_EDGE('',*,*,#18303,.T.);
#24923=ORIENTED_EDGE('',*,*,#18304,.T.);
#24924=ORIENTED_EDGE('',*,*,#18305,.T.);
#24925=ORIENTED_EDGE('',*,*,#18306,.T.);
#24926=ORIENTED_EDGE('',*,*,#18291,.F.);
#24927=ORIENTED_EDGE('',*,*,#18286,.F.);
#24928=ORIENTED_EDGE('',*,*,#18287,.F.);
#24929=ORIENTED_EDGE('',*,*,#18307,.T.);
#24930=ORIENTED_EDGE('',*,*,#18308,.F.);
#24931=ORIENTED_EDGE('',*,*,#18309,.F.);
#24932=ORIENTED_EDGE('',*,*,#18310,.F.);
#24933=ORIENTED_EDGE('',*,*,#18311,.F.);
#24934=ORIENTED_EDGE('',*,*,#18312,.F.);
#24935=ORIENTED_EDGE('',*,*,#18313,.F.);
#24936=ORIENTED_EDGE('',*,*,#18314,.F.);
#24937=ORIENTED_EDGE('',*,*,#18307,.F.);
#24938=ORIENTED_EDGE('',*,*,#18315,.T.);
#24939=ORIENTED_EDGE('',*,*,#18316,.T.);
#24940=ORIENTED_EDGE('',*,*,#18288,.T.);
#24941=ORIENTED_EDGE('',*,*,#18316,.F.);
#24942=ORIENTED_EDGE('',*,*,#18317,.T.);
#24943=ORIENTED_EDGE('',*,*,#18318,.T.);
#24944=ORIENTED_EDGE('',*,*,#18319,.T.);
#24945=ORIENTED_EDGE('',*,*,#18320,.T.);
#24946=ORIENTED_EDGE('',*,*,#18321,.T.);
#24947=ORIENTED_EDGE('',*,*,#18322,.T.);
#24948=ORIENTED_EDGE('',*,*,#18290,.F.);
#24949=ORIENTED_EDGE('',*,*,#18323,.F.);
#24950=ORIENTED_EDGE('',*,*,#18324,.F.);
#24951=ORIENTED_EDGE('',*,*,#18325,.T.);
#24952=ORIENTED_EDGE('',*,*,#18326,.F.);
#24953=ORIENTED_EDGE('',*,*,#18327,.F.);
#24954=ORIENTED_EDGE('',*,*,#18328,.T.);
#24955=ORIENTED_EDGE('',*,*,#18326,.T.);
#24956=ORIENTED_EDGE('',*,*,#18329,.F.);
#24957=ORIENTED_EDGE('',*,*,#18330,.F.);
#24958=ORIENTED_EDGE('',*,*,#18331,.T.);
#24959=ORIENTED_EDGE('',*,*,#18332,.T.);
#24960=ORIENTED_EDGE('',*,*,#18327,.T.);
#24961=ORIENTED_EDGE('',*,*,#18333,.T.);
#24962=ORIENTED_EDGE('',*,*,#18334,.F.);
#24963=ORIENTED_EDGE('',*,*,#18331,.F.);
#24964=ORIENTED_EDGE('',*,*,#18335,.T.);
#24965=ORIENTED_EDGE('',*,*,#18336,.T.);
#24966=ORIENTED_EDGE('',*,*,#18333,.F.);
#24967=ORIENTED_EDGE('',*,*,#18337,.F.);
#24968=ORIENTED_EDGE('',*,*,#18338,.F.);
#24969=ORIENTED_EDGE('',*,*,#18339,.F.);
#24970=ORIENTED_EDGE('',*,*,#18338,.T.);
#24971=ORIENTED_EDGE('',*,*,#18340,.T.);
#24972=ORIENTED_EDGE('',*,*,#18341,.F.);
#24973=ORIENTED_EDGE('',*,*,#18342,.T.);
#24974=ORIENTED_EDGE('',*,*,#18343,.F.);
#24975=ORIENTED_EDGE('',*,*,#18341,.T.);
#24976=ORIENTED_EDGE('',*,*,#18344,.T.);
#24977=ORIENTED_EDGE('',*,*,#18345,.T.);
#24978=ORIENTED_EDGE('',*,*,#18342,.F.);
#24979=ORIENTED_EDGE('',*,*,#18346,.F.);
#24980=ORIENTED_EDGE('',*,*,#18347,.T.);
#24981=ORIENTED_EDGE('',*,*,#18348,.T.);
#24982=ORIENTED_EDGE('',*,*,#18349,.F.);
#24983=ORIENTED_EDGE('',*,*,#18347,.F.);
#24984=ORIENTED_EDGE('',*,*,#18350,.T.);
#24985=ORIENTED_EDGE('',*,*,#18351,.T.);
#24986=ORIENTED_EDGE('',*,*,#18352,.T.);
#24987=ORIENTED_EDGE('',*,*,#18348,.F.);
#24988=ORIENTED_EDGE('',*,*,#18353,.T.);
#24989=ORIENTED_EDGE('',*,*,#18354,.T.);
#24990=ORIENTED_EDGE('',*,*,#18351,.F.);
#24991=ORIENTED_EDGE('',*,*,#18355,.F.);
#24992=ORIENTED_EDGE('',*,*,#18324,.T.);
#24993=ORIENTED_EDGE('',*,*,#17760,.T.);
#24994=ORIENTED_EDGE('',*,*,#18293,.F.);
#24995=ORIENTED_EDGE('',*,*,#18356,.F.);
#24996=ORIENTED_EDGE('',*,*,#18357,.T.);
#24997=ORIENTED_EDGE('',*,*,#18292,.F.);
#24998=ORIENTED_EDGE('',*,*,#18306,.F.);
#24999=ORIENTED_EDGE('',*,*,#18358,.F.);
#25000=ORIENTED_EDGE('',*,*,#18359,.F.);
#25001=ORIENTED_EDGE('',*,*,#18360,.T.);
#25002=ORIENTED_EDGE('',*,*,#18361,.T.);
#25003=ORIENTED_EDGE('',*,*,#18294,.T.);
#25004=ORIENTED_EDGE('',*,*,#17761,.T.);
#25005=ORIENTED_EDGE('',*,*,#18357,.F.);
#25006=ORIENTED_EDGE('',*,*,#18356,.T.);
#25007=ORIENTED_EDGE('',*,*,#18298,.T.);
#25008=ORIENTED_EDGE('',*,*,#18296,.T.);
#25009=ORIENTED_EDGE('',*,*,#18362,.T.);
#25010=ORIENTED_EDGE('',*,*,#18363,.T.);
#25011=ORIENTED_EDGE('',*,*,#18364,.T.);
#25012=ORIENTED_EDGE('',*,*,#18365,.F.);
#25013=ORIENTED_EDGE('',*,*,#18362,.F.);
#25014=ORIENTED_EDGE('',*,*,#18295,.T.);
#25015=ORIENTED_EDGE('',*,*,#18361,.F.);
#25016=ORIENTED_EDGE('',*,*,#18366,.F.);
#25017=ORIENTED_EDGE('',*,*,#18301,.F.);
#25018=ORIENTED_EDGE('',*,*,#18299,.T.);
#25019=ORIENTED_EDGE('',*,*,#18365,.T.);
#25020=ORIENTED_EDGE('',*,*,#18367,.F.);
#25021=ORIENTED_EDGE('',*,*,#18368,.F.);
#25022=ORIENTED_EDGE('',*,*,#18369,.T.);
#25023=ORIENTED_EDGE('',*,*,#18370,.F.);
#25024=ORIENTED_EDGE('',*,*,#18304,.F.);
#25025=ORIENTED_EDGE('',*,*,#18302,.F.);
#25026=ORIENTED_EDGE('',*,*,#18371,.F.);
#25027=ORIENTED_EDGE('',*,*,#18372,.T.);
#25028=ORIENTED_EDGE('',*,*,#18358,.T.);
#25029=ORIENTED_EDGE('',*,*,#18305,.F.);
#25030=ORIENTED_EDGE('',*,*,#18371,.T.);
#25031=ORIENTED_EDGE('',*,*,#18370,.T.);
#25032=ORIENTED_EDGE('',*,*,#18373,.F.);
#25033=ORIENTED_EDGE('',*,*,#18374,.F.);
#25034=ORIENTED_EDGE('',*,*,#18375,.F.);
#25035=ORIENTED_EDGE('',*,*,#18376,.T.);
#25036=ORIENTED_EDGE('',*,*,#18377,.F.);
#25037=ORIENTED_EDGE('',*,*,#18312,.T.);
#25038=ORIENTED_EDGE('',*,*,#18378,.T.);
#25039=ORIENTED_EDGE('',*,*,#18379,.F.);
#25040=ORIENTED_EDGE('',*,*,#18380,.T.);
#25041=ORIENTED_EDGE('',*,*,#18310,.T.);
#25042=ORIENTED_EDGE('',*,*,#18378,.F.);
#25043=ORIENTED_EDGE('',*,*,#18311,.T.);
#25044=ORIENTED_EDGE('',*,*,#18380,.F.);
#25045=ORIENTED_EDGE('',*,*,#18379,.T.);
#25046=ORIENTED_EDGE('',*,*,#18313,.T.);
#25047=ORIENTED_EDGE('',*,*,#18381,.F.);
#25048=ORIENTED_EDGE('',*,*,#18382,.F.);
#25049=ORIENTED_EDGE('',*,*,#18383,.F.);
#25050=ORIENTED_EDGE('',*,*,#18384,.T.);
#25051=ORIENTED_EDGE('',*,*,#18385,.F.);
#25052=ORIENTED_EDGE('',*,*,#18308,.T.);
#25053=ORIENTED_EDGE('',*,*,#18314,.T.);
#25054=ORIENTED_EDGE('',*,*,#18386,.F.);
#25055=ORIENTED_EDGE('',*,*,#18309,.T.);
#25056=ORIENTED_EDGE('',*,*,#18387,.F.);
#25057=ORIENTED_EDGE('',*,*,#18388,.T.);
#25058=ORIENTED_EDGE('',*,*,#18389,.F.);
#25059=ORIENTED_EDGE('',*,*,#18390,.T.);
#25060=ORIENTED_EDGE('',*,*,#18391,.F.);
#25061=ORIENTED_EDGE('',*,*,#18315,.F.);
#25062=ORIENTED_EDGE('',*,*,#18392,.T.);
#25063=ORIENTED_EDGE('',*,*,#18317,.F.);
#25064=ORIENTED_EDGE('',*,*,#18322,.F.);
#25065=ORIENTED_EDGE('',*,*,#18393,.T.);
#25066=ORIENTED_EDGE('',*,*,#18394,.F.);
#25067=ORIENTED_EDGE('',*,*,#18395,.T.);
#25068=ORIENTED_EDGE('',*,*,#18396,.F.);
#25069=ORIENTED_EDGE('',*,*,#18397,.T.);
#25070=ORIENTED_EDGE('',*,*,#18398,.T.);
#25071=ORIENTED_EDGE('',*,*,#18399,.F.);
#25072=ORIENTED_EDGE('',*,*,#18400,.T.);
#25073=ORIENTED_EDGE('',*,*,#18321,.F.);
#25074=ORIENTED_EDGE('',*,*,#18401,.F.);
#25075=ORIENTED_EDGE('',*,*,#18402,.T.);
#25076=ORIENTED_EDGE('',*,*,#18403,.F.);
#25077=ORIENTED_EDGE('',*,*,#18319,.F.);
#25078=ORIENTED_EDGE('',*,*,#18401,.T.);
#25079=ORIENTED_EDGE('',*,*,#18320,.F.);
#25080=ORIENTED_EDGE('',*,*,#18403,.T.);
#25081=ORIENTED_EDGE('',*,*,#18402,.F.);
#25082=ORIENTED_EDGE('',*,*,#18318,.F.);
#25083=ORIENTED_EDGE('',*,*,#18404,.T.);
#25084=ORIENTED_EDGE('',*,*,#18405,.F.);
#25085=ORIENTED_EDGE('',*,*,#18406,.T.);
#25086=ORIENTED_EDGE('',*,*,#18407,.T.);
#25087=ORIENTED_EDGE('',*,*,#18408,.T.);
#25088=ORIENTED_EDGE('',*,*,#18350,.F.);
#25089=ORIENTED_EDGE('',*,*,#18346,.T.);
#25090=ORIENTED_EDGE('',*,*,#18344,.F.);
#25091=ORIENTED_EDGE('',*,*,#18340,.F.);
#25092=ORIENTED_EDGE('',*,*,#18337,.T.);
#25093=ORIENTED_EDGE('',*,*,#18335,.F.);
#25094=ORIENTED_EDGE('',*,*,#18330,.T.);
#25095=ORIENTED_EDGE('',*,*,#18329,.T.);
#25096=ORIENTED_EDGE('',*,*,#18325,.F.);
#25097=ORIENTED_EDGE('',*,*,#18355,.T.);
#25098=ORIENTED_EDGE('',*,*,#18353,.F.);
#25099=ORIENTED_EDGE('',*,*,#18409,.T.);
#25100=ORIENTED_EDGE('',*,*,#18410,.T.);
#25101=ORIENTED_EDGE('',*,*,#18411,.T.);
#25102=ORIENTED_EDGE('',*,*,#18412,.T.);
#25103=ORIENTED_EDGE('',*,*,#18413,.T.);
#25104=ORIENTED_EDGE('',*,*,#18414,.F.);
#25105=ORIENTED_EDGE('',*,*,#18415,.F.);
#25106=ORIENTED_EDGE('',*,*,#18416,.T.);
#25107=ORIENTED_EDGE('',*,*,#18417,.F.);
#25108=ORIENTED_EDGE('',*,*,#18418,.T.);
#25109=ORIENTED_EDGE('',*,*,#18419,.F.);
#25110=ORIENTED_EDGE('',*,*,#18420,.F.);
#25111=ORIENTED_EDGE('',*,*,#18421,.T.);
#25112=ORIENTED_EDGE('',*,*,#18422,.F.);
#25113=ORIENTED_EDGE('',*,*,#18423,.F.);
#25114=ORIENTED_EDGE('',*,*,#18424,.T.);
#25115=ORIENTED_EDGE('',*,*,#18425,.T.);
#25116=ORIENTED_EDGE('',*,*,#18426,.T.);
#25117=ORIENTED_EDGE('',*,*,#18427,.F.);
#25118=ORIENTED_EDGE('',*,*,#18428,.F.);
#25119=ORIENTED_EDGE('',*,*,#18429,.F.);
#25120=ORIENTED_EDGE('',*,*,#18430,.F.);
#25121=ORIENTED_EDGE('',*,*,#18431,.F.);
#25122=ORIENTED_EDGE('',*,*,#18432,.T.);
#25123=ORIENTED_EDGE('',*,*,#18433,.F.);
#25124=ORIENTED_EDGE('',*,*,#18434,.T.);
#25125=ORIENTED_EDGE('',*,*,#18366,.T.);
#25126=ORIENTED_EDGE('',*,*,#18360,.F.);
#25127=ORIENTED_EDGE('',*,*,#18435,.F.);
#25128=ORIENTED_EDGE('',*,*,#18436,.F.);
#25129=ORIENTED_EDGE('',*,*,#18435,.T.);
#25130=ORIENTED_EDGE('',*,*,#18359,.T.);
#25131=ORIENTED_EDGE('',*,*,#18372,.F.);
#25132=ORIENTED_EDGE('',*,*,#18364,.F.);
#25133=ORIENTED_EDGE('',*,*,#18437,.F.);
#25134=ORIENTED_EDGE('',*,*,#18438,.T.);
#25135=ORIENTED_EDGE('',*,*,#18367,.T.);
#25136=ORIENTED_EDGE('',*,*,#18439,.T.);
#25137=ORIENTED_EDGE('',*,*,#18440,.F.);
#25138=ORIENTED_EDGE('',*,*,#18441,.F.);
#25139=ORIENTED_EDGE('',*,*,#18442,.T.);
#25140=ORIENTED_EDGE('',*,*,#18443,.T.);
#25141=ORIENTED_EDGE('',*,*,#18444,.F.);
#25142=ORIENTED_EDGE('',*,*,#18445,.F.);
#25143=ORIENTED_EDGE('',*,*,#18446,.T.);
#25144=ORIENTED_EDGE('',*,*,#18437,.T.);
#25145=ORIENTED_EDGE('',*,*,#18363,.F.);
#25146=ORIENTED_EDGE('',*,*,#18434,.F.);
#25147=ORIENTED_EDGE('',*,*,#18436,.T.);
#25148=ORIENTED_EDGE('',*,*,#18374,.T.);
#25149=ORIENTED_EDGE('',*,*,#18447,.F.);
#25150=ORIENTED_EDGE('',*,*,#18446,.F.);
#25151=ORIENTED_EDGE('',*,*,#18448,.T.);
#25152=ORIENTED_EDGE('',*,*,#18368,.T.);
#25153=ORIENTED_EDGE('',*,*,#18438,.F.);
#25154=ORIENTED_EDGE('',*,*,#18369,.F.);
#25155=ORIENTED_EDGE('',*,*,#18448,.F.);
#25156=ORIENTED_EDGE('',*,*,#18447,.T.);
#25157=ORIENTED_EDGE('',*,*,#18373,.T.);
#25158=ORIENTED_EDGE('',*,*,#18449,.F.);
#25159=ORIENTED_EDGE('',*,*,#18450,.F.);
#25160=ORIENTED_EDGE('',*,*,#18451,.T.);
#25161=ORIENTED_EDGE('',*,*,#18381,.T.);
#25162=ORIENTED_EDGE('',*,*,#18377,.T.);
#25163=ORIENTED_EDGE('',*,*,#18452,.T.);
#25164=ORIENTED_EDGE('',*,*,#18449,.T.);
#25165=ORIENTED_EDGE('',*,*,#18376,.F.);
#25166=ORIENTED_EDGE('',*,*,#18453,.F.);
#25167=ORIENTED_EDGE('',*,*,#18454,.F.);
#25168=ORIENTED_EDGE('',*,*,#18455,.F.);
#25169=ORIENTED_EDGE('',*,*,#18453,.T.);
#25170=ORIENTED_EDGE('',*,*,#18375,.T.);
#25171=ORIENTED_EDGE('',*,*,#18391,.T.);
#25172=ORIENTED_EDGE('',*,*,#18456,.T.);
#25173=ORIENTED_EDGE('',*,*,#18382,.T.);
#25174=ORIENTED_EDGE('',*,*,#18451,.F.);
#25175=ORIENTED_EDGE('',*,*,#18457,.F.);
#25176=ORIENTED_EDGE('',*,*,#18458,.T.);
#25177=ORIENTED_EDGE('',*,*,#18383,.T.);
#25178=ORIENTED_EDGE('',*,*,#18456,.F.);
#25179=ORIENTED_EDGE('',*,*,#18459,.F.);
#25180=ORIENTED_EDGE('',*,*,#18460,.T.);
#25181=ORIENTED_EDGE('',*,*,#18461,.T.);
#25182=ORIENTED_EDGE('',*,*,#18384,.F.);
#25183=ORIENTED_EDGE('',*,*,#18458,.F.);
#25184=ORIENTED_EDGE('',*,*,#18461,.F.);
#25185=ORIENTED_EDGE('',*,*,#18462,.F.);
#25186=ORIENTED_EDGE('',*,*,#18463,.T.);
#25187=ORIENTED_EDGE('',*,*,#18387,.T.);
#25188=ORIENTED_EDGE('',*,*,#18386,.T.);
#25189=ORIENTED_EDGE('',*,*,#18385,.T.);
#25190=ORIENTED_EDGE('',*,*,#18464,.T.);
#25191=ORIENTED_EDGE('',*,*,#18465,.T.);
#25192=ORIENTED_EDGE('',*,*,#18388,.F.);
#25193=ORIENTED_EDGE('',*,*,#18463,.F.);
#25194=ORIENTED_EDGE('',*,*,#18465,.F.);
#25195=ORIENTED_EDGE('',*,*,#18466,.F.);
#25196=ORIENTED_EDGE('',*,*,#18467,.T.);
#25197=ORIENTED_EDGE('',*,*,#18389,.T.);
#25198=ORIENTED_EDGE('',*,*,#18468,.T.);
#25199=ORIENTED_EDGE('',*,*,#18454,.T.);
#25200=ORIENTED_EDGE('',*,*,#18390,.F.);
#25201=ORIENTED_EDGE('',*,*,#18467,.F.);
#25202=ORIENTED_EDGE('',*,*,#18469,.T.);
#25203=ORIENTED_EDGE('',*,*,#18470,.T.);
#25204=ORIENTED_EDGE('',*,*,#18404,.F.);
#25205=ORIENTED_EDGE('',*,*,#18392,.F.);
#25206=ORIENTED_EDGE('',*,*,#18397,.F.);
#25207=ORIENTED_EDGE('',*,*,#18471,.F.);
#25208=ORIENTED_EDGE('',*,*,#18472,.T.);
#25209=ORIENTED_EDGE('',*,*,#18473,.T.);
#25210=ORIENTED_EDGE('',*,*,#18393,.F.);
#25211=ORIENTED_EDGE('',*,*,#18400,.F.);
#25212=ORIENTED_EDGE('',*,*,#18474,.F.);
#25213=ORIENTED_EDGE('',*,*,#18475,.F.);
#25214=ORIENTED_EDGE('',*,*,#18476,.T.);
#25215=ORIENTED_EDGE('',*,*,#18394,.T.);
#25216=ORIENTED_EDGE('',*,*,#18473,.F.);
#25217=ORIENTED_EDGE('',*,*,#18477,.T.);
#25218=ORIENTED_EDGE('',*,*,#18478,.T.);
#25219=ORIENTED_EDGE('',*,*,#18395,.F.);
#25220=ORIENTED_EDGE('',*,*,#18476,.F.);
#25221=ORIENTED_EDGE('',*,*,#18479,.F.);
#25222=ORIENTED_EDGE('',*,*,#18471,.T.);
#25223=ORIENTED_EDGE('',*,*,#18396,.T.);
#25224=ORIENTED_EDGE('',*,*,#18478,.F.);
#25225=ORIENTED_EDGE('',*,*,#18480,.F.);
#25226=ORIENTED_EDGE('',*,*,#18474,.T.);
#25227=ORIENTED_EDGE('',*,*,#18399,.T.);
#25228=ORIENTED_EDGE('',*,*,#18481,.F.);
#25229=ORIENTED_EDGE('',*,*,#18482,.T.);
#25230=ORIENTED_EDGE('',*,*,#18481,.T.);
#25231=ORIENTED_EDGE('',*,*,#18398,.F.);
#25232=ORIENTED_EDGE('',*,*,#18408,.F.);
#25233=ORIENTED_EDGE('',*,*,#18483,.F.);
#25234=ORIENTED_EDGE('',*,*,#18470,.F.);
#25235=ORIENTED_EDGE('',*,*,#18484,.F.);
#25236=ORIENTED_EDGE('',*,*,#18485,.T.);
#25237=ORIENTED_EDGE('',*,*,#18405,.T.);
#25238=ORIENTED_EDGE('',*,*,#18406,.F.);
#25239=ORIENTED_EDGE('',*,*,#18485,.F.);
#25240=ORIENTED_EDGE('',*,*,#18486,.T.);
#25241=ORIENTED_EDGE('',*,*,#18487,.T.);
#25242=ORIENTED_EDGE('',*,*,#18407,.F.);
#25243=ORIENTED_EDGE('',*,*,#18487,.F.);
#25244=ORIENTED_EDGE('',*,*,#18488,.T.);
#25245=ORIENTED_EDGE('',*,*,#18483,.T.);
#25246=ORIENTED_EDGE('',*,*,#18409,.F.);
#25247=ORIENTED_EDGE('',*,*,#18489,.T.);
#25248=ORIENTED_EDGE('',*,*,#18490,.T.);
#25249=ORIENTED_EDGE('',*,*,#18491,.F.);
#25250=ORIENTED_EDGE('',*,*,#18410,.F.);
#25251=ORIENTED_EDGE('',*,*,#18491,.T.);
#25252=ORIENTED_EDGE('',*,*,#18492,.T.);
#25253=ORIENTED_EDGE('',*,*,#18493,.F.);
#25254=ORIENTED_EDGE('',*,*,#18411,.F.);
#25255=ORIENTED_EDGE('',*,*,#18493,.T.);
#25256=ORIENTED_EDGE('',*,*,#18494,.T.);
#25257=ORIENTED_EDGE('',*,*,#18495,.T.);
#25258=ORIENTED_EDGE('',*,*,#18496,.T.);
#25259=ORIENTED_EDGE('',*,*,#18412,.F.);
#25260=ORIENTED_EDGE('',*,*,#18495,.F.);
#25261=ORIENTED_EDGE('',*,*,#18497,.T.);
#25262=ORIENTED_EDGE('',*,*,#18413,.F.);
#25263=ORIENTED_EDGE('',*,*,#18496,.F.);
#25264=ORIENTED_EDGE('',*,*,#18498,.T.);
#25265=ORIENTED_EDGE('',*,*,#18499,.F.);
#25266=ORIENTED_EDGE('',*,*,#18500,.T.);
#25267=ORIENTED_EDGE('',*,*,#18414,.T.);
#25268=ORIENTED_EDGE('',*,*,#18499,.T.);
#25269=ORIENTED_EDGE('',*,*,#18501,.F.);
#25270=ORIENTED_EDGE('',*,*,#18415,.T.);
#25271=ORIENTED_EDGE('',*,*,#18500,.F.);
#25272=ORIENTED_EDGE('',*,*,#18502,.F.);
#25273=ORIENTED_EDGE('',*,*,#18503,.T.);
#25274=ORIENTED_EDGE('',*,*,#18416,.F.);
#25275=ORIENTED_EDGE('',*,*,#18503,.F.);
#25276=ORIENTED_EDGE('',*,*,#18504,.T.);
#25277=ORIENTED_EDGE('',*,*,#18505,.F.);
#25278=ORIENTED_EDGE('',*,*,#18505,.T.);
#25279=ORIENTED_EDGE('',*,*,#18506,.F.);
#25280=ORIENTED_EDGE('',*,*,#18489,.F.);
#25281=ORIENTED_EDGE('',*,*,#18417,.T.);
#25282=ORIENTED_EDGE('',*,*,#18440,.T.);
#25283=ORIENTED_EDGE('',*,*,#18507,.F.);
#25284=ORIENTED_EDGE('',*,*,#18418,.F.);
#25285=ORIENTED_EDGE('',*,*,#18508,.T.);
#25286=ORIENTED_EDGE('',*,*,#18507,.T.);
#25287=ORIENTED_EDGE('',*,*,#18439,.F.);
#25288=ORIENTED_EDGE('',*,*,#18509,.F.);
#25289=ORIENTED_EDGE('',*,*,#18419,.T.);
#25290=ORIENTED_EDGE('',*,*,#18509,.T.);
#25291=ORIENTED_EDGE('',*,*,#18445,.T.);
#25292=ORIENTED_EDGE('',*,*,#18510,.F.);
#25293=ORIENTED_EDGE('',*,*,#18420,.T.);
#25294=ORIENTED_EDGE('',*,*,#18421,.F.);
#25295=ORIENTED_EDGE('',*,*,#18510,.T.);
#25296=ORIENTED_EDGE('',*,*,#18444,.T.);
#25297=ORIENTED_EDGE('',*,*,#18511,.F.);
#25298=ORIENTED_EDGE('',*,*,#18512,.F.);
#25299=ORIENTED_EDGE('',*,*,#18422,.T.);
#25300=ORIENTED_EDGE('',*,*,#18511,.T.);
#25301=ORIENTED_EDGE('',*,*,#18443,.F.);
#25302=ORIENTED_EDGE('',*,*,#18513,.F.);
#25303=ORIENTED_EDGE('',*,*,#18423,.T.);
#25304=ORIENTED_EDGE('',*,*,#18512,.T.);
#25305=ORIENTED_EDGE('',*,*,#18442,.F.);
#25306=ORIENTED_EDGE('',*,*,#18508,.F.);
#25307=ORIENTED_EDGE('',*,*,#18424,.F.);
#25308=ORIENTED_EDGE('',*,*,#18513,.T.);
#25309=ORIENTED_EDGE('',*,*,#18441,.T.);
#25310=ORIENTED_EDGE('',*,*,#18514,.F.);
#25311=ORIENTED_EDGE('',*,*,#18515,.F.);
#25312=ORIENTED_EDGE('',*,*,#18425,.F.);
#25313=ORIENTED_EDGE('',*,*,#18516,.T.);
#25314=ORIENTED_EDGE('',*,*,#18515,.T.);
#25315=ORIENTED_EDGE('',*,*,#18517,.T.);
#25316=ORIENTED_EDGE('',*,*,#18518,.F.);
#25317=ORIENTED_EDGE('',*,*,#18426,.F.);
#25318=ORIENTED_EDGE('',*,*,#18518,.T.);
#25319=ORIENTED_EDGE('',*,*,#18519,.F.);
#25320=ORIENTED_EDGE('',*,*,#18520,.F.);
#25321=ORIENTED_EDGE('',*,*,#18427,.T.);
#25322=ORIENTED_EDGE('',*,*,#18520,.T.);
#25323=ORIENTED_EDGE('',*,*,#18521,.T.);
#25324=ORIENTED_EDGE('',*,*,#18522,.F.);
#25325=ORIENTED_EDGE('',*,*,#18428,.T.);
#25326=ORIENTED_EDGE('',*,*,#18523,.F.);
#25327=ORIENTED_EDGE('',*,*,#18524,.F.);
#25328=ORIENTED_EDGE('',*,*,#18429,.T.);
#25329=ORIENTED_EDGE('',*,*,#18522,.T.);
#25330=ORIENTED_EDGE('',*,*,#18524,.T.);
#25331=ORIENTED_EDGE('',*,*,#18525,.F.);
#25332=ORIENTED_EDGE('',*,*,#18526,.F.);
#25333=ORIENTED_EDGE('',*,*,#18430,.T.);
#25334=ORIENTED_EDGE('',*,*,#18526,.T.);
#25335=ORIENTED_EDGE('',*,*,#18527,.F.);
#25336=ORIENTED_EDGE('',*,*,#18528,.F.);
#25337=ORIENTED_EDGE('',*,*,#18431,.T.);
#25338=ORIENTED_EDGE('',*,*,#18432,.F.);
#25339=ORIENTED_EDGE('',*,*,#18528,.T.);
#25340=ORIENTED_EDGE('',*,*,#18529,.T.);
#25341=ORIENTED_EDGE('',*,*,#18530,.F.);
#25342=ORIENTED_EDGE('',*,*,#18530,.T.);
#25343=ORIENTED_EDGE('',*,*,#18531,.F.);
#25344=ORIENTED_EDGE('',*,*,#18516,.F.);
#25345=ORIENTED_EDGE('',*,*,#18433,.T.);
#25346=ORIENTED_EDGE('',*,*,#18494,.F.);
#25347=ORIENTED_EDGE('',*,*,#18492,.F.);
#25348=ORIENTED_EDGE('',*,*,#18490,.F.);
#25349=ORIENTED_EDGE('',*,*,#18506,.T.);
#25350=ORIENTED_EDGE('',*,*,#18504,.F.);
#25351=ORIENTED_EDGE('',*,*,#18502,.T.);
#25352=ORIENTED_EDGE('',*,*,#18501,.T.);
#25353=ORIENTED_EDGE('',*,*,#18498,.F.);
#25354=ORIENTED_EDGE('',*,*,#18497,.F.);
#25355=ORIENTED_EDGE('',*,*,#18457,.T.);
#25356=ORIENTED_EDGE('',*,*,#18450,.T.);
#25357=ORIENTED_EDGE('',*,*,#18452,.F.);
#25358=ORIENTED_EDGE('',*,*,#18455,.T.);
#25359=ORIENTED_EDGE('',*,*,#18468,.F.);
#25360=ORIENTED_EDGE('',*,*,#18466,.T.);
#25361=ORIENTED_EDGE('',*,*,#18464,.F.);
#25362=ORIENTED_EDGE('',*,*,#18462,.T.);
#25363=ORIENTED_EDGE('',*,*,#18460,.F.);
#25364=ORIENTED_EDGE('',*,*,#18459,.T.);
#25365=ORIENTED_EDGE('',*,*,#18519,.T.);
#25366=ORIENTED_EDGE('',*,*,#18517,.F.);
#25367=ORIENTED_EDGE('',*,*,#18514,.T.);
#25368=ORIENTED_EDGE('',*,*,#18531,.T.);
#25369=ORIENTED_EDGE('',*,*,#18529,.F.);
#25370=ORIENTED_EDGE('',*,*,#18527,.T.);
#25371=ORIENTED_EDGE('',*,*,#18525,.T.);
#25372=ORIENTED_EDGE('',*,*,#18523,.T.);
#25373=ORIENTED_EDGE('',*,*,#18521,.F.);
#25374=ORIENTED_EDGE('',*,*,#18486,.F.);
#25375=ORIENTED_EDGE('',*,*,#18484,.T.);
#25376=ORIENTED_EDGE('',*,*,#18469,.F.);
#25377=ORIENTED_EDGE('',*,*,#18479,.T.);
#25378=ORIENTED_EDGE('',*,*,#18477,.F.);
#25379=ORIENTED_EDGE('',*,*,#18475,.T.);
#25380=ORIENTED_EDGE('',*,*,#18472,.F.);
#25381=ORIENTED_EDGE('',*,*,#18480,.T.);
#25382=ORIENTED_EDGE('',*,*,#18482,.F.);
#25383=ORIENTED_EDGE('',*,*,#18488,.F.);
#25384=ORIENTED_EDGE('',*,*,#18211,.T.);
#25385=ORIENTED_EDGE('',*,*,#18279,.T.);
#25386=ORIENTED_EDGE('',*,*,#18532,.T.);
#25387=ORIENTED_EDGE('',*,*,#18123,.F.);
#25388=ORIENTED_EDGE('',*,*,#18119,.T.);
#25389=ORIENTED_EDGE('',*,*,#18533,.F.);
#25390=ORIENTED_EDGE('',*,*,#18244,.F.);
#25391=ORIENTED_EDGE('',*,*,#18160,.F.);
#25392=ORIENTED_EDGE('',*,*,#18190,.T.);
#25393=ORIENTED_EDGE('',*,*,#18176,.T.);
#25394=ORIENTED_EDGE('',*,*,#18534,.T.);
#25395=ORIENTED_EDGE('',*,*,#18263,.F.);
#25396=ORIENTED_EDGE('',*,*,#18260,.T.);
#25397=ORIENTED_EDGE('',*,*,#18535,.F.);
#25398=ORIENTED_EDGE('',*,*,#18172,.F.);
#25399=ORIENTED_EDGE('',*,*,#18138,.F.);
#25400=ORIENTED_EDGE('',*,*,#18253,.F.);
#25401=ORIENTED_EDGE('',*,*,#18142,.F.);
#25402=ORIENTED_EDGE('',*,*,#18536,.F.);
#25403=ORIENTED_EDGE('',*,*,#18537,.T.);
#25404=ORIENTED_EDGE('',*,*,#18538,.F.);
#25405=ORIENTED_EDGE('',*,*,#18539,.T.);
#25406=ORIENTED_EDGE('',*,*,#18540,.F.);
#25407=ORIENTED_EDGE('',*,*,#18541,.T.);
#25408=ORIENTED_EDGE('',*,*,#18542,.T.);
#25409=ORIENTED_EDGE('',*,*,#18543,.F.);
#25410=ORIENTED_EDGE('',*,*,#18544,.F.);
#25411=ORIENTED_EDGE('',*,*,#18166,.F.);
#25412=ORIENTED_EDGE('',*,*,#18146,.T.);
#25413=ORIENTED_EDGE('',*,*,#18252,.T.);
#25414=ORIENTED_EDGE('',*,*,#18258,.F.);
#25415=ORIENTED_EDGE('',*,*,#18135,.F.);
#25416=ORIENTED_EDGE('',*,*,#18171,.T.);
#25417=ORIENTED_EDGE('',*,*,#18545,.T.);
#25418=ORIENTED_EDGE('',*,*,#18546,.T.);
#25419=ORIENTED_EDGE('',*,*,#18547,.T.);
#25420=ORIENTED_EDGE('',*,*,#18548,.F.);
#25421=ORIENTED_EDGE('',*,*,#18549,.T.);
#25422=ORIENTED_EDGE('',*,*,#18550,.F.);
#25423=ORIENTED_EDGE('',*,*,#18551,.T.);
#25424=ORIENTED_EDGE('',*,*,#18552,.T.);
#25425=ORIENTED_EDGE('',*,*,#18553,.T.);
#25426=ORIENTED_EDGE('',*,*,#18144,.T.);
#25427=ORIENTED_EDGE('',*,*,#18255,.T.);
#25428=ORIENTED_EDGE('',*,*,#18267,.F.);
#25429=ORIENTED_EDGE('',*,*,#18197,.F.);
#25430=ORIENTED_EDGE('',*,*,#18554,.F.);
#25431=ORIENTED_EDGE('',*,*,#18555,.F.);
#25432=ORIENTED_EDGE('',*,*,#18556,.F.);
#25433=ORIENTED_EDGE('',*,*,#18557,.T.);
#25434=ORIENTED_EDGE('',*,*,#18558,.F.);
#25435=ORIENTED_EDGE('',*,*,#18559,.T.);
#25436=ORIENTED_EDGE('',*,*,#18560,.F.);
#25437=ORIENTED_EDGE('',*,*,#18561,.F.);
#25438=ORIENTED_EDGE('',*,*,#18562,.F.);
#25439=ORIENTED_EDGE('',*,*,#18174,.F.);
#25440=ORIENTED_EDGE('',*,*,#18193,.T.);
#25441=ORIENTED_EDGE('',*,*,#18264,.T.);
#25442=ORIENTED_EDGE('',*,*,#18269,.F.);
#25443=ORIENTED_EDGE('',*,*,#18205,.F.);
#25444=ORIENTED_EDGE('',*,*,#18182,.T.);
#25445=ORIENTED_EDGE('',*,*,#18563,.T.);
#25446=ORIENTED_EDGE('',*,*,#18564,.T.);
#25447=ORIENTED_EDGE('',*,*,#18565,.F.);
#25448=ORIENTED_EDGE('',*,*,#18566,.F.);
#25449=ORIENTED_EDGE('',*,*,#18567,.T.);
#25450=ORIENTED_EDGE('',*,*,#18568,.F.);
#25451=ORIENTED_EDGE('',*,*,#18569,.T.);
#25452=ORIENTED_EDGE('',*,*,#18570,.F.);
#25453=ORIENTED_EDGE('',*,*,#18571,.T.);
#25454=ORIENTED_EDGE('',*,*,#18194,.T.);
#25455=ORIENTED_EDGE('',*,*,#18266,.T.);
#25456=ORIENTED_EDGE('',*,*,#18184,.F.);
#25457=ORIENTED_EDGE('',*,*,#18050,.F.);
#25458=ORIENTED_EDGE('',*,*,#17884,.F.);
#25459=ORIENTED_EDGE('',*,*,#18572,.F.);
#25460=ORIENTED_EDGE('',*,*,#18563,.F.);
#25461=ORIENTED_EDGE('',*,*,#17888,.F.);
#25462=ORIENTED_EDGE('',*,*,#18064,.T.);
#25463=ORIENTED_EDGE('',*,*,#18130,.F.);
#25464=ORIENTED_EDGE('',*,*,#18573,.T.);
#25465=ORIENTED_EDGE('',*,*,#18574,.F.);
#25466=ORIENTED_EDGE('',*,*,#18568,.T.);
#25467=ORIENTED_EDGE('',*,*,#18268,.F.);
#25468=ORIENTED_EDGE('',*,*,#18557,.F.);
#25469=ORIENTED_EDGE('',*,*,#18575,.F.);
#25470=ORIENTED_EDGE('',*,*,#18576,.T.);
#25471=ORIENTED_EDGE('',*,*,#18577,.F.);
#25472=ORIENTED_EDGE('',*,*,#18558,.T.);
#25473=ORIENTED_EDGE('',*,*,#18265,.F.);
#25474=ORIENTED_EDGE('',*,*,#18261,.F.);
#25475=ORIENTED_EDGE('',*,*,#18534,.F.);
#25476=ORIENTED_EDGE('',*,*,#18175,.F.);
#25477=ORIENTED_EDGE('',*,*,#18562,.T.);
#25478=ORIENTED_EDGE('',*,*,#18578,.F.);
#25479=ORIENTED_EDGE('',*,*,#17898,.F.);
#25480=ORIENTED_EDGE('',*,*,#18185,.F.);
#25481=ORIENTED_EDGE('',*,*,#17853,.F.);
#25482=ORIENTED_EDGE('',*,*,#18579,.F.);
#25483=ORIENTED_EDGE('',*,*,#18545,.F.);
#25484=ORIENTED_EDGE('',*,*,#18173,.F.);
#25485=ORIENTED_EDGE('',*,*,#18535,.T.);
#25486=ORIENTED_EDGE('',*,*,#18259,.F.);
#25487=ORIENTED_EDGE('',*,*,#18256,.T.);
#25488=ORIENTED_EDGE('',*,*,#18549,.F.);
#25489=ORIENTED_EDGE('',*,*,#18580,.F.);
#25490=ORIENTED_EDGE('',*,*,#18581,.F.);
#25491=ORIENTED_EDGE('',*,*,#18582,.F.);
#25492=ORIENTED_EDGE('',*,*,#18550,.T.);
#25493=ORIENTED_EDGE('',*,*,#18254,.T.);
#25494=ORIENTED_EDGE('',*,*,#18539,.F.);
#25495=ORIENTED_EDGE('',*,*,#18583,.F.);
#25496=ORIENTED_EDGE('',*,*,#18584,.F.);
#25497=ORIENTED_EDGE('',*,*,#18585,.F.);
#25498=ORIENTED_EDGE('',*,*,#18540,.T.);
#25499=ORIENTED_EDGE('',*,*,#18251,.T.);
#25500=ORIENTED_EDGE('',*,*,#18249,.F.);
#25501=ORIENTED_EDGE('',*,*,#18248,.T.);
#25502=ORIENTED_EDGE('',*,*,#18245,.T.);
#25503=ORIENTED_EDGE('',*,*,#18242,.F.);
#25504=ORIENTED_EDGE('',*,*,#18533,.T.);
#25505=ORIENTED_EDGE('',*,*,#18118,.F.);
#25506=ORIENTED_EDGE('',*,*,#18586,.T.);
#25507=ORIENTED_EDGE('',*,*,#18587,.F.);
#25508=ORIENTED_EDGE('',*,*,#17860,.F.);
#25509=ORIENTED_EDGE('',*,*,#18109,.F.);
#25510=ORIENTED_EDGE('',*,*,#17892,.F.);
#25511=ORIENTED_EDGE('',*,*,#18588,.F.);
#25512=ORIENTED_EDGE('',*,*,#18589,.F.);
#25513=ORIENTED_EDGE('',*,*,#18124,.F.);
#25514=ORIENTED_EDGE('',*,*,#18532,.F.);
#25515=ORIENTED_EDGE('',*,*,#18278,.T.);
#25516=ORIENTED_EDGE('',*,*,#18276,.T.);
#25517=ORIENTED_EDGE('',*,*,#18274,.F.);
#25518=ORIENTED_EDGE('',*,*,#18273,.T.);
#25519=ORIENTED_EDGE('',*,*,#18270,.F.);
#25520=ORIENTED_EDGE('',*,*,#18567,.F.);
#25521=ORIENTED_EDGE('',*,*,#18590,.F.);
#25522=ORIENTED_EDGE('',*,*,#18591,.T.);
#25523=ORIENTED_EDGE('',*,*,#18592,.F.);
#25524=ORIENTED_EDGE('',*,*,#18328,.F.);
#25525=ORIENTED_EDGE('',*,*,#18332,.F.);
#25526=ORIENTED_EDGE('',*,*,#18334,.T.);
#25527=ORIENTED_EDGE('',*,*,#18336,.F.);
#25528=ORIENTED_EDGE('',*,*,#18339,.T.);
#25529=ORIENTED_EDGE('',*,*,#18343,.T.);
#25530=ORIENTED_EDGE('',*,*,#18345,.F.);
#25531=ORIENTED_EDGE('',*,*,#18349,.T.);
#25532=ORIENTED_EDGE('',*,*,#18352,.F.);
#25533=ORIENTED_EDGE('',*,*,#18354,.F.);
#25534=ORIENTED_EDGE('',*,*,#18323,.T.);
#25535=ORIENTED_EDGE('',*,*,#17849,.F.);
#25536=ORIENTED_EDGE('',*,*,#18037,.F.);
#25537=ORIENTED_EDGE('',*,*,#18167,.F.);
#25538=ORIENTED_EDGE('',*,*,#18544,.T.);
#25539=ORIENTED_EDGE('',*,*,#18593,.F.);
#25540=ORIENTED_EDGE('',*,*,#18112,.F.);
#25541=ORIENTED_EDGE('',*,*,#18030,.T.);
#25542=ORIENTED_EDGE('',*,*,#17845,.F.);
#25543=ORIENTED_EDGE('',*,*,#18594,.F.);
#25544=ORIENTED_EDGE('',*,*,#18595,.F.);
#25545=ORIENTED_EDGE('',*,*,#18596,.T.);
#25546=ORIENTED_EDGE('',*,*,#18565,.T.);
#25547=ORIENTED_EDGE('',*,*,#18597,.F.);
#25548=ORIENTED_EDGE('',*,*,#18598,.F.);
#25549=ORIENTED_EDGE('',*,*,#17883,.T.);
#25550=ORIENTED_EDGE('',*,*,#18599,.F.);
#25551=ORIENTED_EDGE('',*,*,#18564,.F.);
#25552=ORIENTED_EDGE('',*,*,#18572,.T.);
#25553=ORIENTED_EDGE('',*,*,#18597,.T.);
#25554=ORIENTED_EDGE('',*,*,#18599,.T.);
#25555=ORIENTED_EDGE('',*,*,#18600,.F.);
#25556=ORIENTED_EDGE('',*,*,#18566,.T.);
#25557=ORIENTED_EDGE('',*,*,#18601,.F.);
#25558=ORIENTED_EDGE('',*,*,#18602,.F.);
#25559=ORIENTED_EDGE('',*,*,#18590,.T.);
#25560=ORIENTED_EDGE('',*,*,#18603,.T.);
#25561=ORIENTED_EDGE('',*,*,#18601,.T.);
#25562=ORIENTED_EDGE('',*,*,#18596,.F.);
#25563=ORIENTED_EDGE('',*,*,#18600,.T.);
#25564=ORIENTED_EDGE('',*,*,#17882,.T.);
#25565=ORIENTED_EDGE('',*,*,#18604,.F.);
#25566=ORIENTED_EDGE('',*,*,#18605,.F.);
#25567=ORIENTED_EDGE('',*,*,#18561,.T.);
#25568=ORIENTED_EDGE('',*,*,#18606,.F.);
#25569=ORIENTED_EDGE('',*,*,#17881,.F.);
#25570=ORIENTED_EDGE('',*,*,#18578,.T.);
#25571=ORIENTED_EDGE('',*,*,#18604,.T.);
#25572=ORIENTED_EDGE('',*,*,#18606,.T.);
#25573=ORIENTED_EDGE('',*,*,#18607,.F.);
#25574=ORIENTED_EDGE('',*,*,#18605,.T.);
#25575=ORIENTED_EDGE('',*,*,#18608,.T.);
#25576=ORIENTED_EDGE('',*,*,#18609,.T.);
#25577=ORIENTED_EDGE('',*,*,#18610,.T.);
#25578=ORIENTED_EDGE('',*,*,#18611,.T.);
#25579=ORIENTED_EDGE('',*,*,#18612,.T.);
#25580=ORIENTED_EDGE('',*,*,#18613,.T.);
#25581=ORIENTED_EDGE('',*,*,#18614,.T.);
#25582=ORIENTED_EDGE('',*,*,#18615,.T.);
#25583=ORIENTED_EDGE('',*,*,#18598,.T.);
#25584=ORIENTED_EDGE('',*,*,#18616,.T.);
#25585=ORIENTED_EDGE('',*,*,#18617,.T.);
#25586=ORIENTED_EDGE('',*,*,#18603,.F.);
#25587=ORIENTED_EDGE('',*,*,#18615,.F.);
#25588=ORIENTED_EDGE('',*,*,#18618,.T.);
#25589=ORIENTED_EDGE('',*,*,#18619,.T.);
#25590=ORIENTED_EDGE('',*,*,#18616,.F.);
#25591=ORIENTED_EDGE('',*,*,#18607,.T.);
#25592=ORIENTED_EDGE('',*,*,#18560,.T.);
#25593=ORIENTED_EDGE('',*,*,#18620,.F.);
#25594=ORIENTED_EDGE('',*,*,#18608,.F.);
#25595=ORIENTED_EDGE('',*,*,#18620,.T.);
#25596=ORIENTED_EDGE('',*,*,#18621,.T.);
#25597=ORIENTED_EDGE('',*,*,#18622,.F.);
#25598=ORIENTED_EDGE('',*,*,#18622,.T.);
#25599=ORIENTED_EDGE('',*,*,#18623,.T.);
#25600=ORIENTED_EDGE('',*,*,#18624,.F.);
#25601=ORIENTED_EDGE('',*,*,#18609,.F.);
#25602=ORIENTED_EDGE('',*,*,#18624,.T.);
#25603=ORIENTED_EDGE('',*,*,#18625,.T.);
#25604=ORIENTED_EDGE('',*,*,#18626,.F.);
#25605=ORIENTED_EDGE('',*,*,#18626,.T.);
#25606=ORIENTED_EDGE('',*,*,#18555,.T.);
#25607=ORIENTED_EDGE('',*,*,#18627,.F.);
#25608=ORIENTED_EDGE('',*,*,#18610,.F.);
#25609=ORIENTED_EDGE('',*,*,#18627,.T.);
#25610=ORIENTED_EDGE('',*,*,#18628,.T.);
#25611=ORIENTED_EDGE('',*,*,#18629,.F.);
#25612=ORIENTED_EDGE('',*,*,#18611,.F.);
#25613=ORIENTED_EDGE('',*,*,#18629,.T.);
#25614=ORIENTED_EDGE('',*,*,#18180,.T.);
#25615=ORIENTED_EDGE('',*,*,#18630,.F.);
#25616=ORIENTED_EDGE('',*,*,#18612,.F.);
#25617=ORIENTED_EDGE('',*,*,#18630,.T.);
#25618=ORIENTED_EDGE('',*,*,#18631,.T.);
#25619=ORIENTED_EDGE('',*,*,#18632,.F.);
#25620=ORIENTED_EDGE('',*,*,#18613,.F.);
#25621=ORIENTED_EDGE('',*,*,#18632,.T.);
#25622=ORIENTED_EDGE('',*,*,#18570,.T.);
#25623=ORIENTED_EDGE('',*,*,#18618,.F.);
#25624=ORIENTED_EDGE('',*,*,#18614,.F.);
#25625=ORIENTED_EDGE('',*,*,#18591,.F.);
#25626=ORIENTED_EDGE('',*,*,#18602,.T.);
#25627=ORIENTED_EDGE('',*,*,#18617,.F.);
#25628=ORIENTED_EDGE('',*,*,#18633,.F.);
#25629=ORIENTED_EDGE('',*,*,#18633,.T.);
#25630=ORIENTED_EDGE('',*,*,#18619,.F.);
#25631=ORIENTED_EDGE('',*,*,#18569,.F.);
#25632=ORIENTED_EDGE('',*,*,#18592,.T.);
#25633=ORIENTED_EDGE('',*,*,#18634,.T.);
#25634=ORIENTED_EDGE('',*,*,#18621,.F.);
#25635=ORIENTED_EDGE('',*,*,#18559,.F.);
#25636=ORIENTED_EDGE('',*,*,#18577,.T.);
#25637=ORIENTED_EDGE('',*,*,#18576,.F.);
#25638=ORIENTED_EDGE('',*,*,#18635,.T.);
#25639=ORIENTED_EDGE('',*,*,#18623,.F.);
#25640=ORIENTED_EDGE('',*,*,#18634,.F.);
#25641=ORIENTED_EDGE('',*,*,#18556,.T.);
#25642=ORIENTED_EDGE('',*,*,#18625,.F.);
#25643=ORIENTED_EDGE('',*,*,#18635,.F.);
#25644=ORIENTED_EDGE('',*,*,#18575,.T.);
#25645=ORIENTED_EDGE('',*,*,#18628,.F.);
#25646=ORIENTED_EDGE('',*,*,#18554,.T.);
#25647=ORIENTED_EDGE('',*,*,#18196,.F.);
#25648=ORIENTED_EDGE('',*,*,#18181,.F.);
#25649=ORIENTED_EDGE('',*,*,#18631,.F.);
#25650=ORIENTED_EDGE('',*,*,#18179,.T.);
#25651=ORIENTED_EDGE('',*,*,#18195,.F.);
#25652=ORIENTED_EDGE('',*,*,#18571,.F.);
#25653=ORIENTED_EDGE('',*,*,#18636,.T.);
#25654=ORIENTED_EDGE('',*,*,#18637,.F.);
#25655=ORIENTED_EDGE('',*,*,#18638,.F.);
#25656=ORIENTED_EDGE('',*,*,#18212,.T.);
#25657=ORIENTED_EDGE('',*,*,#18121,.T.);
#25658=ORIENTED_EDGE('',*,*,#18589,.T.);
#25659=ORIENTED_EDGE('',*,*,#18639,.T.);
#25660=ORIENTED_EDGE('',*,*,#18637,.T.);
#25661=ORIENTED_EDGE('',*,*,#18640,.F.);
#25662=ORIENTED_EDGE('',*,*,#18641,.F.);
#25663=ORIENTED_EDGE('',*,*,#17891,.T.);
#25664=ORIENTED_EDGE('',*,*,#18642,.F.);
#25665=ORIENTED_EDGE('',*,*,#18636,.F.);
#25666=ORIENTED_EDGE('',*,*,#18588,.T.);
#25667=ORIENTED_EDGE('',*,*,#18640,.T.);
#25668=ORIENTED_EDGE('',*,*,#18642,.T.);
#25669=ORIENTED_EDGE('',*,*,#18643,.F.);
#25670=ORIENTED_EDGE('',*,*,#18644,.F.);
#25671=ORIENTED_EDGE('',*,*,#18213,.T.);
#25672=ORIENTED_EDGE('',*,*,#18638,.T.);
#25673=ORIENTED_EDGE('',*,*,#18645,.F.);
#25674=ORIENTED_EDGE('',*,*,#18646,.T.);
#25675=ORIENTED_EDGE('',*,*,#18645,.T.);
#25676=ORIENTED_EDGE('',*,*,#18639,.F.);
#25677=ORIENTED_EDGE('',*,*,#18643,.T.);
#25678=ORIENTED_EDGE('',*,*,#17890,.T.);
#25679=ORIENTED_EDGE('',*,*,#18647,.F.);
#25680=ORIENTED_EDGE('',*,*,#18648,.F.);
#25681=ORIENTED_EDGE('',*,*,#18649,.T.);
#25682=ORIENTED_EDGE('',*,*,#18650,.F.);
#25683=ORIENTED_EDGE('',*,*,#17889,.F.);
#25684=ORIENTED_EDGE('',*,*,#18574,.T.);
#25685=ORIENTED_EDGE('',*,*,#18647,.T.);
#25686=ORIENTED_EDGE('',*,*,#18650,.T.);
#25687=ORIENTED_EDGE('',*,*,#18651,.F.);
#25688=ORIENTED_EDGE('',*,*,#18648,.T.);
#25689=ORIENTED_EDGE('',*,*,#18652,.T.);
#25690=ORIENTED_EDGE('',*,*,#18653,.T.);
#25691=ORIENTED_EDGE('',*,*,#18654,.T.);
#25692=ORIENTED_EDGE('',*,*,#18655,.T.);
#25693=ORIENTED_EDGE('',*,*,#18656,.T.);
#25694=ORIENTED_EDGE('',*,*,#18657,.T.);
#25695=ORIENTED_EDGE('',*,*,#18658,.T.);
#25696=ORIENTED_EDGE('',*,*,#18659,.T.);
#25697=ORIENTED_EDGE('',*,*,#18641,.T.);
#25698=ORIENTED_EDGE('',*,*,#18660,.T.);
#25699=ORIENTED_EDGE('',*,*,#18661,.T.);
#25700=ORIENTED_EDGE('',*,*,#18646,.F.);
#25701=ORIENTED_EDGE('',*,*,#18659,.F.);
#25702=ORIENTED_EDGE('',*,*,#18662,.T.);
#25703=ORIENTED_EDGE('',*,*,#18663,.T.);
#25704=ORIENTED_EDGE('',*,*,#18660,.F.);
#25705=ORIENTED_EDGE('',*,*,#18651,.T.);
#25706=ORIENTED_EDGE('',*,*,#18664,.T.);
#25707=ORIENTED_EDGE('',*,*,#18665,.F.);
#25708=ORIENTED_EDGE('',*,*,#18652,.F.);
#25709=ORIENTED_EDGE('',*,*,#18665,.T.);
#25710=ORIENTED_EDGE('',*,*,#18666,.T.);
#25711=ORIENTED_EDGE('',*,*,#18667,.F.);
#25712=ORIENTED_EDGE('',*,*,#18667,.T.);
#25713=ORIENTED_EDGE('',*,*,#18668,.T.);
#25714=ORIENTED_EDGE('',*,*,#18669,.F.);
#25715=ORIENTED_EDGE('',*,*,#18653,.F.);
#25716=ORIENTED_EDGE('',*,*,#18669,.T.);
#25717=ORIENTED_EDGE('',*,*,#18670,.T.);
#25718=ORIENTED_EDGE('',*,*,#18671,.F.);
#25719=ORIENTED_EDGE('',*,*,#18671,.T.);
#25720=ORIENTED_EDGE('',*,*,#18672,.T.);
#25721=ORIENTED_EDGE('',*,*,#18673,.F.);
#25722=ORIENTED_EDGE('',*,*,#18654,.F.);
#25723=ORIENTED_EDGE('',*,*,#18673,.T.);
#25724=ORIENTED_EDGE('',*,*,#18674,.T.);
#25725=ORIENTED_EDGE('',*,*,#18675,.F.);
#25726=ORIENTED_EDGE('',*,*,#18655,.F.);
#25727=ORIENTED_EDGE('',*,*,#18675,.T.);
#25728=ORIENTED_EDGE('',*,*,#18127,.T.);
#25729=ORIENTED_EDGE('',*,*,#18676,.F.);
#25730=ORIENTED_EDGE('',*,*,#18656,.F.);
#25731=ORIENTED_EDGE('',*,*,#18676,.T.);
#25732=ORIENTED_EDGE('',*,*,#18677,.T.);
#25733=ORIENTED_EDGE('',*,*,#18678,.F.);
#25734=ORIENTED_EDGE('',*,*,#18657,.F.);
#25735=ORIENTED_EDGE('',*,*,#18678,.T.);
#25736=ORIENTED_EDGE('',*,*,#18679,.T.);
#25737=ORIENTED_EDGE('',*,*,#18662,.F.);
#25738=ORIENTED_EDGE('',*,*,#18658,.F.);
#25739=ORIENTED_EDGE('',*,*,#18680,.F.);
#25740=ORIENTED_EDGE('',*,*,#18214,.T.);
#25741=ORIENTED_EDGE('',*,*,#18644,.T.);
#25742=ORIENTED_EDGE('',*,*,#18661,.F.);
#25743=ORIENTED_EDGE('',*,*,#18681,.F.);
#25744=ORIENTED_EDGE('',*,*,#18215,.T.);
#25745=ORIENTED_EDGE('',*,*,#18680,.T.);
#25746=ORIENTED_EDGE('',*,*,#18663,.F.);
#25747=ORIENTED_EDGE('',*,*,#18573,.F.);
#25748=ORIENTED_EDGE('',*,*,#18129,.F.);
#25749=ORIENTED_EDGE('',*,*,#18204,.F.);
#25750=ORIENTED_EDGE('',*,*,#18682,.T.);
#25751=ORIENTED_EDGE('',*,*,#18664,.F.);
#25752=ORIENTED_EDGE('',*,*,#18649,.F.);
#25753=ORIENTED_EDGE('',*,*,#18682,.F.);
#25754=ORIENTED_EDGE('',*,*,#18203,.T.);
#25755=ORIENTED_EDGE('',*,*,#18683,.T.);
#25756=ORIENTED_EDGE('',*,*,#18666,.F.);
#25757=ORIENTED_EDGE('',*,*,#18683,.F.);
#25758=ORIENTED_EDGE('',*,*,#18202,.T.);
#25759=ORIENTED_EDGE('',*,*,#18684,.T.);
#25760=ORIENTED_EDGE('',*,*,#18668,.F.);
#25761=ORIENTED_EDGE('',*,*,#18684,.F.);
#25762=ORIENTED_EDGE('',*,*,#18201,.T.);
#25763=ORIENTED_EDGE('',*,*,#18685,.T.);
#25764=ORIENTED_EDGE('',*,*,#18670,.F.);
#25765=ORIENTED_EDGE('',*,*,#18685,.F.);
#25766=ORIENTED_EDGE('',*,*,#18200,.T.);
#25767=ORIENTED_EDGE('',*,*,#18686,.F.);
#25768=ORIENTED_EDGE('',*,*,#18672,.F.);
#25769=ORIENTED_EDGE('',*,*,#18674,.F.);
#25770=ORIENTED_EDGE('',*,*,#18686,.T.);
#25771=ORIENTED_EDGE('',*,*,#18199,.F.);
#25772=ORIENTED_EDGE('',*,*,#18128,.F.);
#25773=ORIENTED_EDGE('',*,*,#18677,.F.);
#25774=ORIENTED_EDGE('',*,*,#18126,.T.);
#25775=ORIENTED_EDGE('',*,*,#18217,.F.);
#25776=ORIENTED_EDGE('',*,*,#18687,.F.);
#25777=ORIENTED_EDGE('',*,*,#18679,.F.);
#25778=ORIENTED_EDGE('',*,*,#18687,.T.);
#25779=ORIENTED_EDGE('',*,*,#18216,.F.);
#25780=ORIENTED_EDGE('',*,*,#18681,.T.);
#25781=ORIENTED_EDGE('',*,*,#18688,.T.);
#25782=ORIENTED_EDGE('',*,*,#18689,.T.);
#25783=ORIENTED_EDGE('',*,*,#18690,.F.);
#25784=ORIENTED_EDGE('',*,*,#18542,.F.);
#25785=ORIENTED_EDGE('',*,*,#18543,.T.);
#25786=ORIENTED_EDGE('',*,*,#18691,.T.);
#25787=ORIENTED_EDGE('',*,*,#17850,.F.);
#25788=ORIENTED_EDGE('',*,*,#18593,.T.);
#25789=ORIENTED_EDGE('',*,*,#18690,.T.);
#25790=ORIENTED_EDGE('',*,*,#18692,.F.);
#25791=ORIENTED_EDGE('',*,*,#18691,.F.);
#25792=ORIENTED_EDGE('',*,*,#18693,.T.);
#25793=ORIENTED_EDGE('',*,*,#18694,.T.);
#25794=ORIENTED_EDGE('',*,*,#18541,.F.);
#25795=ORIENTED_EDGE('',*,*,#18585,.T.);
#25796=ORIENTED_EDGE('',*,*,#18695,.T.);
#25797=ORIENTED_EDGE('',*,*,#18688,.F.);
#25798=ORIENTED_EDGE('',*,*,#18694,.F.);
#25799=ORIENTED_EDGE('',*,*,#18692,.T.);
#25800=ORIENTED_EDGE('',*,*,#18696,.T.);
#25801=ORIENTED_EDGE('',*,*,#18697,.F.);
#25802=ORIENTED_EDGE('',*,*,#17851,.F.);
#25803=ORIENTED_EDGE('',*,*,#17852,.T.);
#25804=ORIENTED_EDGE('',*,*,#18698,.T.);
#25805=ORIENTED_EDGE('',*,*,#18546,.F.);
#25806=ORIENTED_EDGE('',*,*,#18579,.T.);
#25807=ORIENTED_EDGE('',*,*,#18697,.T.);
#25808=ORIENTED_EDGE('',*,*,#18699,.F.);
#25809=ORIENTED_EDGE('',*,*,#18698,.F.);
#25810=ORIENTED_EDGE('',*,*,#18689,.F.);
#25811=ORIENTED_EDGE('',*,*,#18700,.F.);
#25812=ORIENTED_EDGE('',*,*,#18701,.F.);
#25813=ORIENTED_EDGE('',*,*,#18702,.F.);
#25814=ORIENTED_EDGE('',*,*,#18703,.F.);
#25815=ORIENTED_EDGE('',*,*,#18704,.F.);
#25816=ORIENTED_EDGE('',*,*,#18705,.F.);
#25817=ORIENTED_EDGE('',*,*,#18706,.F.);
#25818=ORIENTED_EDGE('',*,*,#18707,.F.);
#25819=ORIENTED_EDGE('',*,*,#18696,.F.);
#25820=ORIENTED_EDGE('',*,*,#18708,.T.);
#25821=ORIENTED_EDGE('',*,*,#18700,.T.);
#25822=ORIENTED_EDGE('',*,*,#18695,.F.);
#25823=ORIENTED_EDGE('',*,*,#18709,.F.);
#25824=ORIENTED_EDGE('',*,*,#18710,.T.);
#25825=ORIENTED_EDGE('',*,*,#18708,.F.);
#25826=ORIENTED_EDGE('',*,*,#18711,.F.);
#25827=ORIENTED_EDGE('',*,*,#18699,.T.);
#25828=ORIENTED_EDGE('',*,*,#18707,.T.);
#25829=ORIENTED_EDGE('',*,*,#18712,.F.);
#25830=ORIENTED_EDGE('',*,*,#18547,.F.);
#25831=ORIENTED_EDGE('',*,*,#18712,.T.);
#25832=ORIENTED_EDGE('',*,*,#18713,.F.);
#25833=ORIENTED_EDGE('',*,*,#18714,.F.);
#25834=ORIENTED_EDGE('',*,*,#18713,.T.);
#25835=ORIENTED_EDGE('',*,*,#18706,.T.);
#25836=ORIENTED_EDGE('',*,*,#18715,.F.);
#25837=ORIENTED_EDGE('',*,*,#18716,.F.);
#25838=ORIENTED_EDGE('',*,*,#18715,.T.);
#25839=ORIENTED_EDGE('',*,*,#18717,.F.);
#25840=ORIENTED_EDGE('',*,*,#18718,.F.);
#25841=ORIENTED_EDGE('',*,*,#18717,.T.);
#25842=ORIENTED_EDGE('',*,*,#18705,.T.);
#25843=ORIENTED_EDGE('',*,*,#18719,.F.);
#25844=ORIENTED_EDGE('',*,*,#18552,.F.);
#25845=ORIENTED_EDGE('',*,*,#18719,.T.);
#25846=ORIENTED_EDGE('',*,*,#18704,.T.);
#25847=ORIENTED_EDGE('',*,*,#18720,.F.);
#25848=ORIENTED_EDGE('',*,*,#18721,.F.);
#25849=ORIENTED_EDGE('',*,*,#18720,.T.);
#25850=ORIENTED_EDGE('',*,*,#18703,.T.);
#25851=ORIENTED_EDGE('',*,*,#18722,.F.);
#25852=ORIENTED_EDGE('',*,*,#18169,.F.);
#25853=ORIENTED_EDGE('',*,*,#18722,.T.);
#25854=ORIENTED_EDGE('',*,*,#18702,.T.);
#25855=ORIENTED_EDGE('',*,*,#18723,.F.);
#25856=ORIENTED_EDGE('',*,*,#18724,.F.);
#25857=ORIENTED_EDGE('',*,*,#18723,.T.);
#25858=ORIENTED_EDGE('',*,*,#18701,.T.);
#25859=ORIENTED_EDGE('',*,*,#18710,.F.);
#25860=ORIENTED_EDGE('',*,*,#18537,.F.);
#25861=ORIENTED_EDGE('',*,*,#18725,.T.);
#25862=ORIENTED_EDGE('',*,*,#18709,.T.);
#25863=ORIENTED_EDGE('',*,*,#18693,.F.);
#25864=ORIENTED_EDGE('',*,*,#18584,.T.);
#25865=ORIENTED_EDGE('',*,*,#18538,.T.);
#25866=ORIENTED_EDGE('',*,*,#18711,.T.);
#25867=ORIENTED_EDGE('',*,*,#18725,.F.);
#25868=ORIENTED_EDGE('',*,*,#18583,.T.);
#25869=ORIENTED_EDGE('',*,*,#18548,.T.);
#25870=ORIENTED_EDGE('',*,*,#18714,.T.);
#25871=ORIENTED_EDGE('',*,*,#18726,.F.);
#25872=ORIENTED_EDGE('',*,*,#18580,.T.);
#25873=ORIENTED_EDGE('',*,*,#18726,.T.);
#25874=ORIENTED_EDGE('',*,*,#18716,.T.);
#25875=ORIENTED_EDGE('',*,*,#18727,.F.);
#25876=ORIENTED_EDGE('',*,*,#18581,.T.);
#25877=ORIENTED_EDGE('',*,*,#18727,.T.);
#25878=ORIENTED_EDGE('',*,*,#18718,.T.);
#25879=ORIENTED_EDGE('',*,*,#18551,.F.);
#25880=ORIENTED_EDGE('',*,*,#18582,.T.);
#25881=ORIENTED_EDGE('',*,*,#18721,.T.);
#25882=ORIENTED_EDGE('',*,*,#18168,.T.);
#25883=ORIENTED_EDGE('',*,*,#18145,.F.);
#25884=ORIENTED_EDGE('',*,*,#18553,.F.);
#25885=ORIENTED_EDGE('',*,*,#18724,.T.);
#25886=ORIENTED_EDGE('',*,*,#18536,.T.);
#25887=ORIENTED_EDGE('',*,*,#18141,.F.);
#25888=ORIENTED_EDGE('',*,*,#18170,.F.);
#25889=ORIENTED_EDGE('',*,*,#18586,.F.);
#25890=ORIENTED_EDGE('',*,*,#18117,.F.);
#25891=ORIENTED_EDGE('',*,*,#18159,.F.);
#25892=ORIENTED_EDGE('',*,*,#18728,.T.);
#25893=ORIENTED_EDGE('',*,*,#18729,.T.);
#25894=ORIENTED_EDGE('',*,*,#18730,.F.);
#25895=ORIENTED_EDGE('',*,*,#18731,.T.);
#25896=ORIENTED_EDGE('',*,*,#18732,.T.);
#25897=ORIENTED_EDGE('',*,*,#18733,.F.);
#25898=ORIENTED_EDGE('',*,*,#18729,.F.);
#25899=ORIENTED_EDGE('',*,*,#18728,.F.);
#25900=ORIENTED_EDGE('',*,*,#18158,.T.);
#25901=ORIENTED_EDGE('',*,*,#18734,.T.);
#25902=ORIENTED_EDGE('',*,*,#18735,.T.);
#25903=ORIENTED_EDGE('',*,*,#18736,.T.);
#25904=ORIENTED_EDGE('',*,*,#18731,.F.);
#25905=ORIENTED_EDGE('',*,*,#18735,.F.);
#25906=ORIENTED_EDGE('',*,*,#18730,.T.);
#25907=ORIENTED_EDGE('',*,*,#18737,.T.);
#25908=ORIENTED_EDGE('',*,*,#17842,.F.);
#25909=ORIENTED_EDGE('',*,*,#18587,.T.);
#25910=ORIENTED_EDGE('',*,*,#18733,.T.);
#25911=ORIENTED_EDGE('',*,*,#18738,.F.);
#25912=ORIENTED_EDGE('',*,*,#18737,.F.);
#25913=ORIENTED_EDGE('',*,*,#18732,.F.);
#25914=ORIENTED_EDGE('',*,*,#18739,.F.);
#25915=ORIENTED_EDGE('',*,*,#18740,.F.);
#25916=ORIENTED_EDGE('',*,*,#18741,.F.);
#25917=ORIENTED_EDGE('',*,*,#18742,.F.);
#25918=ORIENTED_EDGE('',*,*,#18743,.F.);
#25919=ORIENTED_EDGE('',*,*,#18744,.F.);
#25920=ORIENTED_EDGE('',*,*,#18745,.F.);
#25921=ORIENTED_EDGE('',*,*,#18746,.F.);
#25922=ORIENTED_EDGE('',*,*,#18747,.F.);
#25923=ORIENTED_EDGE('',*,*,#18748,.T.);
#25924=ORIENTED_EDGE('',*,*,#18739,.T.);
#25925=ORIENTED_EDGE('',*,*,#18736,.F.);
#25926=ORIENTED_EDGE('',*,*,#18749,.F.);
#25927=ORIENTED_EDGE('',*,*,#18750,.T.);
#25928=ORIENTED_EDGE('',*,*,#18748,.F.);
#25929=ORIENTED_EDGE('',*,*,#18751,.F.);
#25930=ORIENTED_EDGE('',*,*,#18738,.T.);
#25931=ORIENTED_EDGE('',*,*,#18747,.T.);
#25932=ORIENTED_EDGE('',*,*,#18752,.F.);
#25933=ORIENTED_EDGE('',*,*,#17843,.F.);
#25934=ORIENTED_EDGE('',*,*,#18752,.T.);
#25935=ORIENTED_EDGE('',*,*,#18753,.F.);
#25936=ORIENTED_EDGE('',*,*,#18754,.F.);
#25937=ORIENTED_EDGE('',*,*,#18755,.T.);
#25938=ORIENTED_EDGE('',*,*,#18745,.T.);
#25939=ORIENTED_EDGE('',*,*,#18756,.F.);
#25940=ORIENTED_EDGE('',*,*,#18757,.F.);
#25941=ORIENTED_EDGE('',*,*,#18758,.T.);
#25942=ORIENTED_EDGE('',*,*,#18755,.F.);
#25943=ORIENTED_EDGE('',*,*,#18759,.F.);
#25944=ORIENTED_EDGE('',*,*,#18756,.T.);
#25945=ORIENTED_EDGE('',*,*,#18760,.F.);
#25946=ORIENTED_EDGE('',*,*,#18761,.F.);
#25947=ORIENTED_EDGE('',*,*,#18753,.T.);
#25948=ORIENTED_EDGE('',*,*,#18746,.T.);
#25949=ORIENTED_EDGE('',*,*,#18758,.F.);
#25950=ORIENTED_EDGE('',*,*,#18762,.F.);
#25951=ORIENTED_EDGE('',*,*,#18760,.T.);
#25952=ORIENTED_EDGE('',*,*,#18744,.T.);
#25953=ORIENTED_EDGE('',*,*,#18763,.F.);
#25954=ORIENTED_EDGE('',*,*,#18764,.F.);
#25955=ORIENTED_EDGE('',*,*,#18763,.T.);
#25956=ORIENTED_EDGE('',*,*,#18743,.T.);
#25957=ORIENTED_EDGE('',*,*,#18765,.F.);
#25958=ORIENTED_EDGE('',*,*,#18766,.F.);
#25959=ORIENTED_EDGE('',*,*,#18765,.T.);
#25960=ORIENTED_EDGE('',*,*,#18742,.T.);
#25961=ORIENTED_EDGE('',*,*,#18767,.F.);
#25962=ORIENTED_EDGE('',*,*,#18115,.F.);
#25963=ORIENTED_EDGE('',*,*,#18767,.T.);
#25964=ORIENTED_EDGE('',*,*,#18741,.T.);
#25965=ORIENTED_EDGE('',*,*,#18768,.F.);
#25966=ORIENTED_EDGE('',*,*,#18769,.F.);
#25967=ORIENTED_EDGE('',*,*,#18768,.T.);
#25968=ORIENTED_EDGE('',*,*,#18740,.T.);
#25969=ORIENTED_EDGE('',*,*,#18750,.F.);
#25970=ORIENTED_EDGE('',*,*,#18770,.F.);
#25971=ORIENTED_EDGE('',*,*,#18749,.T.);
#25972=ORIENTED_EDGE('',*,*,#18734,.F.);
#25973=ORIENTED_EDGE('',*,*,#18157,.F.);
#25974=ORIENTED_EDGE('',*,*,#18771,.T.);
#25975=ORIENTED_EDGE('',*,*,#18771,.F.);
#25976=ORIENTED_EDGE('',*,*,#18156,.T.);
#25977=ORIENTED_EDGE('',*,*,#18772,.T.);
#25978=ORIENTED_EDGE('',*,*,#18751,.T.);
#25979=ORIENTED_EDGE('',*,*,#17844,.T.);
#25980=ORIENTED_EDGE('',*,*,#18754,.T.);
#25981=ORIENTED_EDGE('',*,*,#18773,.F.);
#25982=ORIENTED_EDGE('',*,*,#18594,.T.);
#25983=ORIENTED_EDGE('',*,*,#18757,.T.);
#25984=ORIENTED_EDGE('',*,*,#18774,.F.);
#25985=ORIENTED_EDGE('',*,*,#18150,.F.);
#25986=ORIENTED_EDGE('',*,*,#18775,.T.);
#25987=ORIENTED_EDGE('',*,*,#18775,.F.);
#25988=ORIENTED_EDGE('',*,*,#18149,.T.);
#25989=ORIENTED_EDGE('',*,*,#18776,.T.);
#25990=ORIENTED_EDGE('',*,*,#18759,.T.);
#25991=ORIENTED_EDGE('',*,*,#18777,.F.);
#25992=ORIENTED_EDGE('',*,*,#18151,.T.);
#25993=ORIENTED_EDGE('',*,*,#18774,.T.);
#25994=ORIENTED_EDGE('',*,*,#18761,.T.);
#25995=ORIENTED_EDGE('',*,*,#18773,.T.);
#25996=ORIENTED_EDGE('',*,*,#18762,.T.);
#25997=ORIENTED_EDGE('',*,*,#18776,.F.);
#25998=ORIENTED_EDGE('',*,*,#18148,.T.);
#25999=ORIENTED_EDGE('',*,*,#18110,.T.);
#26000=ORIENTED_EDGE('',*,*,#18595,.T.);
#26001=ORIENTED_EDGE('',*,*,#18764,.T.);
#26002=ORIENTED_EDGE('',*,*,#18778,.T.);
#26003=ORIENTED_EDGE('',*,*,#18152,.F.);
#26004=ORIENTED_EDGE('',*,*,#18777,.T.);
#26005=ORIENTED_EDGE('',*,*,#18766,.T.);
#26006=ORIENTED_EDGE('',*,*,#18114,.T.);
#26007=ORIENTED_EDGE('',*,*,#18153,.F.);
#26008=ORIENTED_EDGE('',*,*,#18778,.F.);
#26009=ORIENTED_EDGE('',*,*,#18769,.T.);
#26010=ORIENTED_EDGE('',*,*,#18779,.T.);
#26011=ORIENTED_EDGE('',*,*,#18154,.F.);
#26012=ORIENTED_EDGE('',*,*,#18116,.F.);
#26013=ORIENTED_EDGE('',*,*,#18772,.F.);
#26014=ORIENTED_EDGE('',*,*,#18155,.T.);
#26015=ORIENTED_EDGE('',*,*,#18779,.F.);
#26016=ORIENTED_EDGE('',*,*,#18770,.T.);
#32477=ADVANCED_FACE('',(#3729),#2131,.F.);
#32478=ADVANCED_FACE('',(#3730),#2620,.T.);
#32479=ADVANCED_FACE('',(#3731),#2132,.F.);
#32480=ADVANCED_FACE('',(#3732),#1106,.T.);
#32481=ADVANCED_FACE('',(#3733),#2133,.T.);
#32482=ADVANCED_FACE('',(#3734),#2134,.F.);
#32483=ADVANCED_FACE('',(#3735),#2135,.T.);
#32484=ADVANCED_FACE('',(#3736),#2621,.T.);
#32485=ADVANCED_FACE('',(#3737),#1107,.F.);
#32486=ADVANCED_FACE('',(#3738),#2136,.T.);
#32487=ADVANCED_FACE('',(#3739),#2622,.F.);
#32488=ADVANCED_FACE('',(#3740),#2623,.F.);
#32489=ADVANCED_FACE('',(#3741),#2137,.F.);
#32490=ADVANCED_FACE('',(#3742,#1274,#1275,#1276,#1277,#1278,#1279),#2138,
 .F.);
#32491=ADVANCED_FACE('',(#3743),#2624,.F.);
#32492=ADVANCED_FACE('',(#3744),#2139,.F.);
#32493=ADVANCED_FACE('',(#3745),#2140,.F.);
#32494=ADVANCED_FACE('',(#3746),#2141,.T.);
#32495=ADVANCED_FACE('',(#3747),#2625,.T.);
#32496=ADVANCED_FACE('',(#3748),#2142,.F.);
#32497=ADVANCED_FACE('',(#3749),#1108,.T.);
#32498=ADVANCED_FACE('',(#3750),#2143,.T.);
#32499=ADVANCED_FACE('',(#3751),#2626,.T.);
#32500=ADVANCED_FACE('',(#3752),#2144,.T.);
#32501=ADVANCED_FACE('',(#3753),#1109,.F.);
#32502=ADVANCED_FACE('',(#3754),#2145,.F.);
#32503=ADVANCED_FACE('',(#3755),#2627,.T.);
#32504=ADVANCED_FACE('',(#3756),#2146,.F.);
#32505=ADVANCED_FACE('',(#3757),#1110,.F.);
#32506=ADVANCED_FACE('',(#3758),#2147,.T.);
#32507=ADVANCED_FACE('',(#3759),#2628,.T.);
#32508=ADVANCED_FACE('',(#3760),#2148,.T.);
#32509=ADVANCED_FACE('',(#3761),#1111,.T.);
#32510=ADVANCED_FACE('',(#3762),#2149,.F.);
#32511=ADVANCED_FACE('',(#3763),#2629,.F.);
#32512=ADVANCED_FACE('',(#3764),#2150,.T.);
#32513=ADVANCED_FACE('',(#3765),#2630,.T.);
#32514=ADVANCED_FACE('',(#3766),#2631,.F.);
#32515=ADVANCED_FACE('',(#3767),#2632,.T.);
#32516=ADVANCED_FACE('',(#3768),#2151,.T.);
#32517=ADVANCED_FACE('',(#3769),#2152,.F.);
#32518=ADVANCED_FACE('',(#3770),#2153,.T.);
#32519=ADVANCED_FACE('',(#3771),#2633,.F.);
#32520=ADVANCED_FACE('',(#3772),#2154,.T.);
#32521=ADVANCED_FACE('',(#3773),#2155,.T.);
#32522=ADVANCED_FACE('',(#3774),#2634,.T.);
#32523=ADVANCED_FACE('',(#3775),#2635,.F.);
#32524=ADVANCED_FACE('',(#3776),#2636,.F.);
#32525=ADVANCED_FACE('',(#3777),#2637,.T.);
#32526=ADVANCED_FACE('',(#3778),#2156,.F.);
#32527=ADVANCED_FACE('',(#3779),#2157,.T.);
#32528=ADVANCED_FACE('',(#3780),#2638,.T.);
#32529=ADVANCED_FACE('',(#3781),#2158,.T.);
#32530=ADVANCED_FACE('',(#3782),#2639,.F.);
#32531=ADVANCED_FACE('',(#3783),#2159,.F.);
#32532=ADVANCED_FACE('',(#3784),#2160,.F.);
#32533=ADVANCED_FACE('',(#3785),#2640,.T.);
#32534=ADVANCED_FACE('',(#3786),#2641,.T.);
#32535=ADVANCED_FACE('',(#3787),#2642,.F.);
#32536=ADVANCED_FACE('',(#3788),#2161,.T.);
#32537=ADVANCED_FACE('',(#3789),#2643,.T.);
#32538=ADVANCED_FACE('',(#3790),#2644,.F.);
#32539=ADVANCED_FACE('',(#3791),#2645,.T.);
#32540=ADVANCED_FACE('',(#3792),#2646,.T.);
#32541=ADVANCED_FACE('',(#3793),#2647,.F.);
#32542=ADVANCED_FACE('',(#3794),#2648,.T.);
#32543=ADVANCED_FACE('',(#3795),#2162,.F.);
#32544=ADVANCED_FACE('',(#3796),#2649,.T.);
#32545=ADVANCED_FACE('',(#3797),#2163,.T.);
#32546=ADVANCED_FACE('',(#3798),#2164,.T.);
#32547=ADVANCED_FACE('',(#3799),#2650,.F.);
#32548=ADVANCED_FACE('',(#3800),#2165,.F.);
#32549=ADVANCED_FACE('',(#3801),#2651,.T.);
#32550=ADVANCED_FACE('',(#3802),#2652,.T.);
#32551=ADVANCED_FACE('',(#3803),#2166,.F.);
#32552=ADVANCED_FACE('',(#3804),#2167,.T.);
#32553=ADVANCED_FACE('',(#3805),#2168,.T.);
#32554=ADVANCED_FACE('',(#3806),#2169,.T.);
#32555=ADVANCED_FACE('',(#3807),#2170,.F.);
#32556=ADVANCED_FACE('',(#3808),#2171,.F.);
#32557=ADVANCED_FACE('',(#3809),#2172,.T.);
#32558=ADVANCED_FACE('',(#3810),#2173,.T.);
#32559=ADVANCED_FACE('',(#3811),#2174,.T.);
#32560=ADVANCED_FACE('',(#3812),#2175,.F.);
#32561=ADVANCED_FACE('',(#3813),#2176,.T.);
#32562=ADVANCED_FACE('',(#3814),#2177,.F.);
#32563=ADVANCED_FACE('',(#3815),#2178,.F.);
#32564=ADVANCED_FACE('',(#3816),#2179,.F.);
#32565=ADVANCED_FACE('',(#3817),#2180,.T.);
#32566=ADVANCED_FACE('',(#3818),#2181,.T.);
#32567=ADVANCED_FACE('',(#3819),#2653,.T.);
#32568=ADVANCED_FACE('',(#3820),#2654,.T.);
#32569=ADVANCED_FACE('',(#3821),#2182,.F.);
#32570=ADVANCED_FACE('',(#3822),#2183,.F.);
#32571=ADVANCED_FACE('',(#3823),#2184,.F.);
#32572=ADVANCED_FACE('',(#3824),#2185,.F.);
#32573=ADVANCED_FACE('',(#3825),#2186,.F.);
#32574=ADVANCED_FACE('',(#3826),#2187,.F.);
#32575=ADVANCED_FACE('',(#3827),#2188,.F.);
#32576=ADVANCED_FACE('',(#3828),#2189,.F.);
#32577=ADVANCED_FACE('',(#3829),#2190,.F.);
#32578=ADVANCED_FACE('',(#3830),#2191,.F.);
#32579=ADVANCED_FACE('',(#3831),#2192,.F.);
#32580=ADVANCED_FACE('',(#3832),#2193,.F.);
#32581=ADVANCED_FACE('',(#3833),#120,.T.);
#32582=ADVANCED_FACE('',(#3834,#1280,#1281,#1282),#2194,.T.);
#32583=ADVANCED_FACE('',(#3835),#2195,.F.);
#32584=ADVANCED_FACE('',(#3836),#2196,.F.);
#32585=ADVANCED_FACE('',(#3837),#2197,.F.);
#32586=ADVANCED_FACE('',(#3838),#121,.T.);
#32587=ADVANCED_FACE('',(#3839),#2655,.T.);
#32588=ADVANCED_FACE('',(#3840),#2656,.F.);
#32589=ADVANCED_FACE('',(#3841),#2657,.F.);
#32590=ADVANCED_FACE('',(#3842),#2658,.F.);
#32591=ADVANCED_FACE('',(#3843),#2659,.F.);
#32592=ADVANCED_FACE('',(#3844),#2660,.F.);
#32593=ADVANCED_FACE('',(#3845),#2661,.F.);
#32594=ADVANCED_FACE('',(#3846),#2662,.F.);
#32595=ADVANCED_FACE('',(#3847),#2198,.T.);
#32596=ADVANCED_FACE('',(#3848),#2199,.T.);
#32597=ADVANCED_FACE('',(#3849),#2663,.T.);
#32598=ADVANCED_FACE('',(#3850),#2200,.T.);
#32599=ADVANCED_FACE('',(#3851),#2201,.T.);
#32600=ADVANCED_FACE('',(#3852),#2202,.T.);
#32601=ADVANCED_FACE('',(#3853),#2664,.F.);
#32602=ADVANCED_FACE('',(#3854),#2665,.F.);
#32603=ADVANCED_FACE('',(#3855),#2666,.F.);
#32604=ADVANCED_FACE('',(#3856),#2667,.F.);
#32605=ADVANCED_FACE('',(#3857),#2668,.F.);
#32606=ADVANCED_FACE('',(#3858),#2669,.F.);
#32607=ADVANCED_FACE('',(#3859),#2670,.F.);
#32608=ADVANCED_FACE('',(#3860),#2203,.T.);
#32609=ADVANCED_FACE('',(#3861),#2671,.T.);
#32610=ADVANCED_FACE('',(#3862),#2672,.T.);
#32611=ADVANCED_FACE('',(#3863),#2204,.T.);
#32612=ADVANCED_FACE('',(#3864),#2205,.F.);
#32613=ADVANCED_FACE('',(#3865),#2206,.T.);
#32614=ADVANCED_FACE('',(#3866),#2207,.T.);
#32615=ADVANCED_FACE('',(#3867),#2208,.T.);
#32616=ADVANCED_FACE('',(#3868,#1283),#2209,.F.);
#32617=ADVANCED_FACE('',(#3869),#2673,.T.);
#32618=ADVANCED_FACE('',(#3870),#2674,.F.);
#32619=ADVANCED_FACE('',(#3871),#2675,.T.);
#32620=ADVANCED_FACE('',(#3872),#2676,.F.);
#32621=ADVANCED_FACE('',(#3873),#2677,.T.);
#32622=ADVANCED_FACE('',(#3874),#2210,.F.);
#32623=ADVANCED_FACE('',(#3875),#2678,.T.);
#32624=ADVANCED_FACE('',(#3876),#2679,.T.);
#32625=ADVANCED_FACE('',(#3877),#2211,.T.);
#32626=ADVANCED_FACE('',(#3878),#2680,.T.);
#32627=ADVANCED_FACE('',(#3879),#2681,.T.);
#32628=ADVANCED_FACE('',(#3880,#1284),#2212,.F.);
#32629=ADVANCED_FACE('',(#3881),#2682,.T.);
#32630=ADVANCED_FACE('',(#3882),#2683,.F.);
#32631=ADVANCED_FACE('',(#3883),#1112,.T.);
#32632=ADVANCED_FACE('',(#3884),#1113,.F.);
#32633=ADVANCED_FACE('',(#3885),#1114,.T.);
#32634=ADVANCED_FACE('',(#3886),#1115,.T.);
#32635=ADVANCED_FACE('',(#3887),#1116,.T.);
#32636=ADVANCED_FACE('',(#3888),#2684,.T.);
#32637=ADVANCED_FACE('',(#3889),#2685,.T.);
#32638=ADVANCED_FACE('',(#3890),#1117,.F.);
#32639=ADVANCED_FACE('',(#3891),#1118,.F.);
#32640=ADVANCED_FACE('',(#3892),#1119,.F.);
#32641=ADVANCED_FACE('',(#3893),#1120,.T.);
#32642=ADVANCED_FACE('',(#3894),#1121,.F.);
#32643=ADVANCED_FACE('',(#3895),#2686,.F.);
#32644=ADVANCED_FACE('',(#3896),#2687,.T.);
#32645=ADVANCED_FACE('',(#3897),#2688,.F.);
#32646=ADVANCED_FACE('',(#3898,#1285),#2213,.F.);
#32647=ADVANCED_FACE('',(#3899,#1286),#2214,.F.);
#32648=ADVANCED_FACE('',(#3900,#1287),#2215,.F.);
#32649=ADVANCED_FACE('',(#3901),#2689,.F.);
#32650=ADVANCED_FACE('',(#3902),#2216,.T.);
#32651=ADVANCED_FACE('',(#3903),#2690,.F.);
#32652=ADVANCED_FACE('',(#3904),#2217,.F.);
#32653=ADVANCED_FACE('',(#3905),#2691,.T.);
#32654=ADVANCED_FACE('',(#3906),#2692,.T.);
#32655=ADVANCED_FACE('',(#3907),#2218,.T.);
#32656=ADVANCED_FACE('',(#3908),#2693,.F.);
#32657=ADVANCED_FACE('',(#3909),#2694,.F.);
#32658=ADVANCED_FACE('',(#3910),#2219,.T.);
#32659=ADVANCED_FACE('',(#3911),#2695,.F.);
#32660=ADVANCED_FACE('',(#3912),#2696,.T.);
#32661=ADVANCED_FACE('',(#3913),#1122,.F.);
#32662=ADVANCED_FACE('',(#3914),#1123,.T.);
#32663=ADVANCED_FACE('',(#3915),#1124,.F.);
#32664=ADVANCED_FACE('',(#3916),#2697,.F.);
#32665=ADVANCED_FACE('',(#3917),#1125,.T.);
#32666=ADVANCED_FACE('',(#3918),#1126,.F.);
#32667=ADVANCED_FACE('',(#3919),#1127,.T.);
#32668=ADVANCED_FACE('',(#3920),#2698,.T.);
#32669=ADVANCED_FACE('',(#3921),#2699,.F.);
#32670=ADVANCED_FACE('',(#3922),#2220,.F.);
#32671=ADVANCED_FACE('',(#3923),#2221,.F.);
#32672=ADVANCED_FACE('',(#3924),#2222,.F.);
#32673=ADVANCED_FACE('',(#3925),#1128,.F.);
#32674=ADVANCED_FACE('',(#3926),#2223,.T.);
#32675=ADVANCED_FACE('',(#3927),#2224,.F.);
#32676=ADVANCED_FACE('',(#3928),#1129,.T.);
#32677=ADVANCED_FACE('',(#3929),#2225,.F.);
#32678=ADVANCED_FACE('',(#3930),#2226,.F.);
#32679=ADVANCED_FACE('',(#3931),#2227,.T.);
#32680=ADVANCED_FACE('',(#3932),#2228,.F.);
#32681=ADVANCED_FACE('',(#3933),#2229,.T.);
#32682=ADVANCED_FACE('',(#3934),#2230,.F.);
#32683=ADVANCED_FACE('',(#3935),#2231,.T.);
#32684=ADVANCED_FACE('',(#3936),#2232,.F.);
#32685=ADVANCED_FACE('',(#3937),#2233,.F.);
#32686=ADVANCED_FACE('',(#3938),#2234,.T.);
#32687=ADVANCED_FACE('',(#3939,#1288,#1289,#1290),#2235,.T.);
#32688=ADVANCED_FACE('',(#3940),#2700,.F.);
#32689=ADVANCED_FACE('',(#3941),#2701,.F.);
#32690=ADVANCED_FACE('',(#3942),#1130,.T.);
#32691=ADVANCED_FACE('',(#3943,#1291),#2236,.T.);
#32692=ADVANCED_FACE('',(#3944),#2702,.F.);
#32693=ADVANCED_FACE('',(#3945),#1131,.F.);
#32694=ADVANCED_FACE('',(#3946),#1132,.T.);
#32695=ADVANCED_FACE('',(#3947),#2703,.F.);
#32696=ADVANCED_FACE('',(#3948),#1133,.T.);
#32697=ADVANCED_FACE('',(#3949),#1134,.T.);
#32698=ADVANCED_FACE('',(#3950),#1135,.T.);
#32699=ADVANCED_FACE('',(#3951),#1136,.F.);
#32700=ADVANCED_FACE('',(#3952),#1137,.T.);
#32701=ADVANCED_FACE('',(#3953),#2704,.F.);
#32702=ADVANCED_FACE('',(#3954),#2237,.T.);
#32703=ADVANCED_FACE('',(#3955),#2705,.F.);
#32704=ADVANCED_FACE('',(#3956),#1138,.F.);
#32705=ADVANCED_FACE('',(#3957),#1139,.F.);
#32706=ADVANCED_FACE('',(#3958),#2706,.F.);
#32707=ADVANCED_FACE('',(#3959),#2238,.F.);
#32708=ADVANCED_FACE('',(#3960),#2707,.F.);
#32709=ADVANCED_FACE('',(#3961),#2708,.F.);
#32710=ADVANCED_FACE('',(#3962),#1140,.F.);
#32711=ADVANCED_FACE('',(#3963),#1141,.T.);
#32712=ADVANCED_FACE('',(#3964),#1142,.F.);
#32713=ADVANCED_FACE('',(#3965),#1143,.F.);
#32714=ADVANCED_FACE('',(#3966),#1144,.F.);
#32715=ADVANCED_FACE('',(#3967),#1145,.F.);
#32716=ADVANCED_FACE('',(#3968),#2709,.F.);
#32717=ADVANCED_FACE('',(#3969),#2710,.T.);
#32718=ADVANCED_FACE('',(#3970),#2239,.F.);
#32719=ADVANCED_FACE('',(#3971),#2711,.T.);
#32720=ADVANCED_FACE('',(#3972),#2712,.F.);
#32721=ADVANCED_FACE('',(#3973),#1146,.F.);
#32722=ADVANCED_FACE('',(#3974),#1147,.T.);
#32723=ADVANCED_FACE('',(#3975),#1148,.F.);
#32724=ADVANCED_FACE('',(#3976),#1149,.T.);
#32725=ADVANCED_FACE('',(#3977),#2713,.T.);
#32726=ADVANCED_FACE('',(#3978),#1150,.F.);
#32727=ADVANCED_FACE('',(#3979),#1151,.T.);
#32728=ADVANCED_FACE('',(#3980),#2714,.T.);
#32729=ADVANCED_FACE('',(#3981),#2715,.T.);
#32730=ADVANCED_FACE('',(#3982),#2716,.F.);
#32731=ADVANCED_FACE('',(#3983),#2717,.T.);
#32732=ADVANCED_FACE('',(#3984),#2240,.T.);
#32733=ADVANCED_FACE('',(#3985),#2718,.T.);
#32734=ADVANCED_FACE('',(#3986),#2719,.F.);
#32735=ADVANCED_FACE('',(#3987),#1152,.T.);
#32736=ADVANCED_FACE('',(#3988),#1153,.T.);
#32737=ADVANCED_FACE('',(#3989),#1154,.F.);
#32738=ADVANCED_FACE('',(#3990),#1155,.T.);
#32739=ADVANCED_FACE('',(#3991,#1292),#2241,.T.);
#32740=ADVANCED_FACE('',(#3992,#1293),#2242,.T.);
#32741=ADVANCED_FACE('',(#3993),#2243,.F.);
#32742=ADVANCED_FACE('',(#3994),#2244,.T.);
#32743=ADVANCED_FACE('',(#3995),#2245,.F.);
#32744=ADVANCED_FACE('',(#3996),#2246,.T.);
#32745=ADVANCED_FACE('',(#3997),#2247,.F.);
#32746=ADVANCED_FACE('',(#3998),#2248,.T.);
#32747=ADVANCED_FACE('',(#3999),#2249,.F.);
#32748=ADVANCED_FACE('',(#4000),#2250,.T.);
#32749=ADVANCED_FACE('',(#4001),#2251,.F.);
#32750=ADVANCED_FACE('',(#4002),#2252,.T.);
#32751=ADVANCED_FACE('',(#4003),#2253,.F.);
#32752=ADVANCED_FACE('',(#4004),#2254,.T.);
#32753=ADVANCED_FACE('',(#4005),#2255,.T.);
#32754=ADVANCED_FACE('',(#4006),#2256,.T.);
#32755=ADVANCED_FACE('',(#4007,#1294),#2257,.T.);
#32756=ADVANCED_FACE('',(#4008),#2258,.T.);
#32757=ADVANCED_FACE('',(#4009),#2259,.T.);
#32758=ADVANCED_FACE('',(#4010),#2720,.T.);
#32759=ADVANCED_FACE('',(#4011),#2721,.T.);
#32760=ADVANCED_FACE('',(#4012),#712,.T.);
#32761=ADVANCED_FACE('',(#4013),#2722,.T.);
#32762=ADVANCED_FACE('',(#4014),#713,.T.);
#32763=ADVANCED_FACE('',(#4015),#122,.T.);
#32764=ADVANCED_FACE('',(#4016),#2723,.T.);
#32765=ADVANCED_FACE('',(#4017),#714,.T.);
#32766=ADVANCED_FACE('',(#4018),#2260,.T.);
#32767=ADVANCED_FACE('',(#4019),#2724,.T.);
#32768=ADVANCED_FACE('',(#4020),#715,.T.);
#32769=ADVANCED_FACE('',(#4021),#2725,.T.);
#32770=ADVANCED_FACE('',(#4022),#716,.T.);
#32771=ADVANCED_FACE('',(#4023),#2726,.T.);
#32772=ADVANCED_FACE('',(#4024),#717,.T.);
#32773=ADVANCED_FACE('',(#4025),#2727,.T.);
#32774=ADVANCED_FACE('',(#4026),#123,.T.);
#32775=ADVANCED_FACE('',(#4027),#124,.T.);
#32776=ADVANCED_FACE('',(#4028),#125,.T.);
#32777=ADVANCED_FACE('',(#4029),#2728,.T.);
#32778=ADVANCED_FACE('',(#4030),#2261,.F.);
#32779=ADVANCED_FACE('',(#4031),#2729,.T.);
#32780=ADVANCED_FACE('',(#4032),#2730,.T.);
#32781=ADVANCED_FACE('',(#4033),#2262,.F.);
#32782=ADVANCED_FACE('',(#4034),#2731,.T.);
#32783=ADVANCED_FACE('',(#4035),#2732,.F.);
#32784=ADVANCED_FACE('',(#4036),#2733,.F.);
#32785=ADVANCED_FACE('',(#4037),#2263,.T.);
#32786=ADVANCED_FACE('',(#4038),#2734,.T.);
#32787=ADVANCED_FACE('',(#4039),#2735,.T.);
#32788=ADVANCED_FACE('',(#4040),#718,.T.);
#32789=ADVANCED_FACE('',(#4041),#2736,.T.);
#32790=ADVANCED_FACE('',(#4042),#719,.T.);
#32791=ADVANCED_FACE('',(#4043),#126,.T.);
#32792=ADVANCED_FACE('',(#4044),#2737,.T.);
#32793=ADVANCED_FACE('',(#4045),#720,.T.);
#32794=ADVANCED_FACE('',(#4046),#2264,.T.);
#32795=ADVANCED_FACE('',(#4047),#2738,.T.);
#32796=ADVANCED_FACE('',(#4048),#721,.T.);
#32797=ADVANCED_FACE('',(#4049),#2739,.T.);
#32798=ADVANCED_FACE('',(#4050),#722,.T.);
#32799=ADVANCED_FACE('',(#4051),#2740,.T.);
#32800=ADVANCED_FACE('',(#4052),#723,.T.);
#32801=ADVANCED_FACE('',(#4053),#2741,.T.);
#32802=ADVANCED_FACE('',(#4054),#127,.T.);
#32803=ADVANCED_FACE('',(#4055),#128,.T.);
#32804=ADVANCED_FACE('',(#4056),#129,.T.);
#32805=ADVANCED_FACE('',(#4057),#2742,.T.);
#32806=ADVANCED_FACE('',(#4058),#2265,.T.);
#32807=ADVANCED_FACE('',(#4059),#2743,.T.);
#32808=ADVANCED_FACE('',(#4060),#2266,.F.);
#32809=ADVANCED_FACE('',(#4061),#2744,.T.);
#32810=ADVANCED_FACE('',(#4062),#2267,.T.);
#32811=ADVANCED_FACE('',(#4063),#2745,.T.);
#32812=ADVANCED_FACE('',(#4064),#2268,.T.);
#32813=ADVANCED_FACE('',(#4065),#2746,.F.);
#32814=ADVANCED_FACE('',(#4066),#2747,.F.);
#32815=ADVANCED_FACE('',(#4067),#2269,.F.);
#32816=ADVANCED_FACE('',(#4068),#2748,.T.);
#32817=ADVANCED_FACE('',(#4069),#2749,.T.);
#32818=ADVANCED_FACE('',(#4070),#724,.T.);
#32819=ADVANCED_FACE('',(#4071),#2750,.T.);
#32820=ADVANCED_FACE('',(#4072),#725,.T.);
#32821=ADVANCED_FACE('',(#4073),#130,.T.);
#32822=ADVANCED_FACE('',(#4074),#2751,.T.);
#32823=ADVANCED_FACE('',(#4075),#726,.T.);
#32824=ADVANCED_FACE('',(#4076),#2270,.T.);
#32825=ADVANCED_FACE('',(#4077),#2752,.T.);
#32826=ADVANCED_FACE('',(#4078),#727,.T.);
#32827=ADVANCED_FACE('',(#4079),#2753,.T.);
#32828=ADVANCED_FACE('',(#4080),#728,.T.);
#32829=ADVANCED_FACE('',(#4081),#2754,.T.);
#32830=ADVANCED_FACE('',(#4082),#729,.T.);
#32831=ADVANCED_FACE('',(#4083),#2755,.T.);
#32832=ADVANCED_FACE('',(#4084),#131,.T.);
#32833=ADVANCED_FACE('',(#4085),#132,.T.);
#32834=ADVANCED_FACE('',(#4086),#133,.T.);
#32835=ADVANCED_FACE('',(#4087),#2756,.T.);
#32836=ADVANCED_FACE('',(#4088),#2271,.T.);
#32837=ADVANCED_FACE('',(#4089),#2757,.T.);
#32838=ADVANCED_FACE('',(#4090),#2758,.T.);
#32839=ADVANCED_FACE('',(#4091),#2272,.T.);
#32840=ADVANCED_FACE('',(#4092),#2759,.T.);
#32841=ADVANCED_FACE('',(#4093),#2760,.F.);
#32842=ADVANCED_FACE('',(#4094),#2761,.F.);
#32843=ADVANCED_FACE('',(#4095),#2273,.F.);
#32844=ADVANCED_FACE('',(#4096),#2762,.T.);
#32845=ADVANCED_FACE('',(#4097),#2763,.T.);
#32846=ADVANCED_FACE('',(#4098),#730,.T.);
#32847=ADVANCED_FACE('',(#4099),#2764,.T.);
#32848=ADVANCED_FACE('',(#4100),#731,.T.);
#32849=ADVANCED_FACE('',(#4101),#2274,.T.);
#32850=ADVANCED_FACE('',(#4102),#2765,.T.);
#32851=ADVANCED_FACE('',(#4103),#732,.T.);
#32852=ADVANCED_FACE('',(#4104),#134,.T.);
#32853=ADVANCED_FACE('',(#4105),#733,.T.);
#32854=ADVANCED_FACE('',(#4106),#2766,.T.);
#32855=ADVANCED_FACE('',(#4107),#734,.T.);
#32856=ADVANCED_FACE('',(#4108),#735,.T.);
#32857=ADVANCED_FACE('',(#4109),#2767,.T.);
#32858=ADVANCED_FACE('',(#4110),#2768,.T.);
#32859=ADVANCED_FACE('',(#4111),#135,.T.);
#32860=ADVANCED_FACE('',(#4112),#136,.T.);
#32861=ADVANCED_FACE('',(#4113),#137,.T.);
#32862=ADVANCED_FACE('',(#4114),#2769,.T.);
#32863=ADVANCED_FACE('',(#4115),#2275,.F.);
#32864=ADVANCED_FACE('',(#4116),#2770,.T.);
#32865=ADVANCED_FACE('',(#4117),#2771,.T.);
#32866=ADVANCED_FACE('',(#4118),#2276,.F.);
#32867=ADVANCED_FACE('',(#4119),#2772,.T.);
#32868=ADVANCED_FACE('',(#4120),#2773,.T.);
#32869=ADVANCED_FACE('',(#4121),#2277,.T.);
#32870=ADVANCED_FACE('',(#4122),#2278,.F.);
#32871=ADVANCED_FACE('',(#4123),#2774,.F.);
#32872=ADVANCED_FACE('',(#4124),#2775,.F.);
#32873=ADVANCED_FACE('',(#4125),#2279,.T.);
#34171=CLOSED_SHELL('',(#32477,#32478,#32479,#32480,#32481));
#34172=CLOSED_SHELL('',(#32482,#32483,#32484,#32485,#32486));
#34173=CLOSED_SHELL('',(#32487,#32488,#32489,#32490,#32491,#32492,#32493,
#32494,#32495,#32496,#32497,#32498,#32499,#32500,#32501,#32502,#32503,#32504,
#32505,#32506,#32507,#32508,#32509,#32510,#32511,#32512,#32513,#32514,#32515,
#32516,#32517,#32518,#32519,#32520,#32521,#32522,#32523,#32524,#32525,#32526,
#32527,#32528,#32529,#32530,#32531,#32532,#32533,#32534,#32535,#32536,#32537,
#32538,#32539,#32540,#32541,#32542,#32543,#32544,#32545,#32546,#32547,#32548,
#32549,#32550,#32551,#32552,#32553,#32554,#32555,#32556,#32557,#32558,#32559,
#32560,#32561,#32562,#32563,#32564,#32565,#32566,#32567,#32568,#32569,#32570,
#32571,#32572,#32573,#32574,#32575,#32576,#32577,#32578,#32579,#32580,#32581,
#32582,#32583,#32584,#32585,#32586,#32587,#32588,#32589,#32590,#32591,#32592,
#32593,#32594,#32595,#32596,#32597,#32598,#32599,#32600,#32601,#32602,#32603,
#32604,#32605,#32606,#32607,#32608,#32609,#32610,#32611,#32612,#32613,#32614,
#32615,#32616,#32617,#32618,#32619,#32620,#32621,#32622,#32623,#32624,#32625,
#32626,#32627,#32628,#32629,#32630,#32631,#32632,#32633,#32634,#32635,#32636,
#32637,#32638,#32639,#32640,#32641,#32642,#32643,#32644,#32645,#32646,#32647,
#32648,#32649,#32650,#32651,#32652,#32653,#32654,#32655,#32656,#32657,#32658,
#32659,#32660,#32661,#32662,#32663,#32664,#32665,#32666,#32667,#32668,#32669,
#32670,#32671,#32672,#32673,#32674,#32675,#32676,#32677,#32678,#32679,#32680,
#32681,#32682,#32683,#32684,#32685,#32686,#32687,#32688,#32689,#32690,#32691,
#32692,#32693,#32694,#32695,#32696,#32697,#32698,#32699,#32700,#32701,#32702,
#32703,#32704,#32705,#32706,#32707,#32708,#32709,#32710,#32711,#32712,#32713,
#32714,#32715,#32716,#32717,#32718,#32719,#32720,#32721,#32722,#32723,#32724,
#32725,#32726,#32727,#32728,#32729,#32730,#32731,#32732,#32733,#32734,#32735,
#32736,#32737,#32738,#32739,#32740,#32741,#32742,#32743,#32744,#32745,#32746,
#32747,#32748,#32749,#32750,#32751,#32752,#32753,#32754,#32755,#32756,#32757,
#32758,#32759,#32760,#32761,#32762,#32763,#32764,#32765,#32766,#32767,#32768,
#32769,#32770,#32771,#32772,#32773,#32774,#32775,#32776,#32777,#32778,#32779,
#32780,#32781,#32782,#32783,#32784,#32785,#32786,#32787,#32788,#32789,#32790,
#32791,#32792,#32793,#32794,#32795,#32796,#32797,#32798,#32799,#32800,#32801,
#32802,#32803,#32804,#32805,#32806,#32807,#32808,#32809,#32810,#32811,#32812,
#32813,#32814,#32815,#32816,#32817,#32818,#32819,#32820,#32821,#32822,#32823,
#32824,#32825,#32826,#32827,#32828,#32829,#32830,#32831,#32832,#32833,#32834,
#32835,#32836,#32837,#32838,#32839,#32840,#32841,#32842,#32843,#32844,#32845,
#32846,#32847,#32848,#32849,#32850,#32851,#32852,#32853,#32854,#32855,#32856,
#32857,#32858,#32859,#32860,#32861,#32862,#32863,#32864,#32865,#32866,#32867,
#32868,#32869,#32870,#32871,#32872,#32873));
#34962=AXIS2_PLACEMENT_3D('',#74301,#40272,#40273);
#34963=AXIS2_PLACEMENT_3D('',#74302,#40274,#40275);
#34964=AXIS2_PLACEMENT_3D('',#74311,#40277,#40278);
#34965=AXIS2_PLACEMENT_3D('',#74312,#40279,#40280);
#34966=AXIS2_PLACEMENT_3D('',#74317,#40283,#40284);
#34967=AXIS2_PLACEMENT_3D('',#74318,#40285,#40286);
#34968=AXIS2_PLACEMENT_3D('',#74334,#40289,#40290);
#34969=AXIS2_PLACEMENT_3D('',#74335,#40291,#40292);
#34970=AXIS2_PLACEMENT_3D('',#74343,#40293,#40294);
#34971=AXIS2_PLACEMENT_3D('',#74345,#40296,#40297);
#34972=AXIS2_PLACEMENT_3D('',#74351,#40301,#40302);
#34973=AXIS2_PLACEMENT_3D('',#74354,#40304,#40305);
#34974=AXIS2_PLACEMENT_3D('',#74367,#40306,#40307);
#34975=AXIS2_PLACEMENT_3D('',#74368,#40308,#40309);
#34976=AXIS2_PLACEMENT_3D('',#74371,#40310,#40311);
#34977=AXIS2_PLACEMENT_3D('',#74375,#40313,#40314);
#34978=AXIS2_PLACEMENT_3D('',#74377,#40315,#40316);
#34979=AXIS2_PLACEMENT_3D('',#74379,#40318,#40319);
#34980=AXIS2_PLACEMENT_3D('',#74382,#40320,#40321);
#34981=AXIS2_PLACEMENT_3D('',#74386,#40323,#40324);
#34982=AXIS2_PLACEMENT_3D('',#74388,#40326,#40327);
#34983=AXIS2_PLACEMENT_3D('',#74399,#40333,#40334);
#34984=AXIS2_PLACEMENT_3D('',#74412,#40337,#40338);
#34985=AXIS2_PLACEMENT_3D('',#74424,#40341,#40342);
#34986=AXIS2_PLACEMENT_3D('',#74436,#40345,#40346);
#34987=AXIS2_PLACEMENT_3D('',#74447,#40349,#40350);
#34988=AXIS2_PLACEMENT_3D('',#74452,#40352,#40353);
#34989=AXIS2_PLACEMENT_3D('',#74454,#40354,#40355);
#34990=AXIS2_PLACEMENT_3D('',#74456,#40356,#40357);
#34991=AXIS2_PLACEMENT_3D('',#74459,#40359,#40360);
#34992=AXIS2_PLACEMENT_3D('',#74462,#40361,#40362);
#34993=AXIS2_PLACEMENT_3D('',#74464,#40363,#40364);
#34994=AXIS2_PLACEMENT_3D('',#74470,#40367,#40368);
#34995=AXIS2_PLACEMENT_3D('',#74480,#40373,#40374);
#34996=AXIS2_PLACEMENT_3D('',#74482,#40375,#40376);
#34997=AXIS2_PLACEMENT_3D('',#74484,#40378,#40379);
#34998=AXIS2_PLACEMENT_3D('',#74487,#40380,#40381);
#34999=AXIS2_PLACEMENT_3D('',#74489,#40382,#40383);
#35000=AXIS2_PLACEMENT_3D('',#74495,#40386,#40387);
#35001=AXIS2_PLACEMENT_3D('',#74498,#40389,#40390);
#35002=AXIS2_PLACEMENT_3D('',#74503,#40392,#40393);
#35003=AXIS2_PLACEMENT_3D('',#74505,#40394,#40395);
#35004=AXIS2_PLACEMENT_3D('',#74507,#40396,#40397);
#35005=AXIS2_PLACEMENT_3D('',#74509,#40398,#40399);
#35006=AXIS2_PLACEMENT_3D('',#74511,#40400,#40401);
#35007=AXIS2_PLACEMENT_3D('',#74513,#40402,#40403);
#35008=AXIS2_PLACEMENT_3D('',#74515,#40405,#40406);
#35009=AXIS2_PLACEMENT_3D('',#74518,#40407,#40408);
#35010=AXIS2_PLACEMENT_3D('',#74520,#40409,#40410);
#35011=AXIS2_PLACEMENT_3D('',#74524,#40412,#40413);
#35012=AXIS2_PLACEMENT_3D('',#74529,#40416,#40417);
#35013=AXIS2_PLACEMENT_3D('',#74530,#40418,#40419);
#35014=AXIS2_PLACEMENT_3D('',#74532,#40420,#40421);
#35015=AXIS2_PLACEMENT_3D('',#74534,#40423,#40424);
#35016=AXIS2_PLACEMENT_3D('',#74536,#40425,#40426);
#35017=AXIS2_PLACEMENT_3D('',#74538,#40428,#40429);
#35018=AXIS2_PLACEMENT_3D('',#74542,#40431,#40432);
#35019=AXIS2_PLACEMENT_3D('',#74551,#40433,#40434);
#35020=AXIS2_PLACEMENT_3D('',#74555,#40437,#40438);
#35021=AXIS2_PLACEMENT_3D('',#74559,#40441,#40442);
#35022=AXIS2_PLACEMENT_3D('',#74564,#40444,#40445);
#35023=AXIS2_PLACEMENT_3D('',#74568,#40447,#40448);
#35024=AXIS2_PLACEMENT_3D('',#74572,#40450,#40451);
#35025=AXIS2_PLACEMENT_3D('',#74576,#40453,#40454);
#35026=AXIS2_PLACEMENT_3D('',#74580,#40456,#40457);
#35027=AXIS2_PLACEMENT_3D('',#74584,#40459,#40460);
#35028=AXIS2_PLACEMENT_3D('',#74588,#40462,#40463);
#35029=AXIS2_PLACEMENT_3D('',#74593,#40466,#40467);
#35030=AXIS2_PLACEMENT_3D('',#74596,#40469,#40470);
#35031=AXIS2_PLACEMENT_3D('',#74597,#40471,#40472);
#35032=AXIS2_PLACEMENT_3D('',#74618,#40476,#40477);
#35033=AXIS2_PLACEMENT_3D('',#74622,#40480,#40481);
#35034=AXIS2_PLACEMENT_3D('',#74626,#40483,#40484);
#35035=AXIS2_PLACEMENT_3D('',#74641,#40486,#40487);
#35036=AXIS2_PLACEMENT_3D('',#74655,#40489,#40490);
#35037=AXIS2_PLACEMENT_3D('',#74656,#40491,#40492);
#35038=AXIS2_PLACEMENT_3D('',#74677,#40496,#40497);
#35039=AXIS2_PLACEMENT_3D('',#74681,#40500,#40501);
#35040=AXIS2_PLACEMENT_3D('',#74686,#40503,#40504);
#35041=AXIS2_PLACEMENT_3D('',#74690,#40506,#40507);
#35042=AXIS2_PLACEMENT_3D('',#74694,#40509,#40510);
#35043=AXIS2_PLACEMENT_3D('',#74698,#40512,#40513);
#35044=AXIS2_PLACEMENT_3D('',#74702,#40515,#40516);
#35045=AXIS2_PLACEMENT_3D('',#74706,#40518,#40519);
#35046=AXIS2_PLACEMENT_3D('',#74709,#40521,#40522);
#35047=AXIS2_PLACEMENT_3D('',#74713,#40524,#40525);
#35048=AXIS2_PLACEMENT_3D('',#74716,#40527,#40528);
#35049=AXIS2_PLACEMENT_3D('',#74717,#40529,#40530);
#35050=AXIS2_PLACEMENT_3D('',#74738,#40534,#40535);
#35051=AXIS2_PLACEMENT_3D('',#74742,#40538,#40539);
#35052=AXIS2_PLACEMENT_3D('',#74746,#40541,#40542);
#35053=AXIS2_PLACEMENT_3D('',#74761,#40544,#40545);
#35054=AXIS2_PLACEMENT_3D('',#74775,#40547,#40548);
#35055=AXIS2_PLACEMENT_3D('',#74776,#40549,#40550);
#35056=AXIS2_PLACEMENT_3D('',#74797,#40554,#40555);
#35057=AXIS2_PLACEMENT_3D('',#74799,#40557,#40558);
#35058=AXIS2_PLACEMENT_3D('',#74805,#40561,#40562);
#35059=AXIS2_PLACEMENT_3D('',#74807,#40563,#40564);
#35060=AXIS2_PLACEMENT_3D('',#74808,#40565,#40566);
#35061=AXIS2_PLACEMENT_3D('',#74809,#40567,#40568);
#35062=AXIS2_PLACEMENT_3D('',#74815,#40572,#40573);
#35063=AXIS2_PLACEMENT_3D('',#74819,#40575,#40576);
#35064=AXIS2_PLACEMENT_3D('',#74821,#40577,#40578);
#35065=AXIS2_PLACEMENT_3D('',#74823,#40579,#40580);
#35066=AXIS2_PLACEMENT_3D('',#74824,#40581,#40582);
#35067=AXIS2_PLACEMENT_3D('',#74825,#40583,#40584);
#35068=AXIS2_PLACEMENT_3D('',#74828,#40586,#40587);
#35069=AXIS2_PLACEMENT_3D('',#74829,#40588,#40589);
#35070=AXIS2_PLACEMENT_3D('',#74832,#40590,#40591);
#35071=AXIS2_PLACEMENT_3D('',#74834,#40592,#40593);
#35072=AXIS2_PLACEMENT_3D('',#74836,#40594,#40595);
#35073=AXIS2_PLACEMENT_3D('',#74837,#40596,#40597);
#35074=AXIS2_PLACEMENT_3D('',#74839,#40599,#40600);
#35075=AXIS2_PLACEMENT_3D('',#74843,#40603,#40604);
#35076=AXIS2_PLACEMENT_3D('',#74851,#40609,#40610);
#35077=AXIS2_PLACEMENT_3D('',#74857,#40614,#40615);
#35078=AXIS2_PLACEMENT_3D('',#74860,#40617,#40618);
#35079=AXIS2_PLACEMENT_3D('',#74861,#40619,#40620);
#35080=AXIS2_PLACEMENT_3D('',#74867,#40624,#40625);
#35081=AXIS2_PLACEMENT_3D('',#74871,#40628,#40629);
#35082=AXIS2_PLACEMENT_3D('',#74875,#40631,#40632);
#35083=AXIS2_PLACEMENT_3D('',#74876,#40633,#40634);
#35084=AXIS2_PLACEMENT_3D('',#74877,#40635,#40636);
#35085=AXIS2_PLACEMENT_3D('',#74878,#40637,#40638);
#35086=AXIS2_PLACEMENT_3D('',#74879,#40639,#40640);
#35087=AXIS2_PLACEMENT_3D('',#74882,#40642,#40643);
#35088=AXIS2_PLACEMENT_3D('',#74883,#40644,#40645);
#35089=AXIS2_PLACEMENT_3D('',#74884,#40646,#40647);
#35090=AXIS2_PLACEMENT_3D('',#74886,#40649,#40650);
#35091=AXIS2_PLACEMENT_3D('',#74888,#40652,#40653);
#35092=AXIS2_PLACEMENT_3D('',#74889,#40654,#40655);
#35093=AXIS2_PLACEMENT_3D('',#74893,#40657,#40658);
#35094=AXIS2_PLACEMENT_3D('',#74895,#40660,#40661);
#35095=AXIS2_PLACEMENT_3D('',#74899,#40664,#40665);
#35096=AXIS2_PLACEMENT_3D('',#74903,#40667,#40668);
#35097=AXIS2_PLACEMENT_3D('',#74904,#40669,#40670);
#35098=AXIS2_PLACEMENT_3D('',#74905,#40671,#40672);
#35099=AXIS2_PLACEMENT_3D('',#74911,#40676,#40677);
#35100=AXIS2_PLACEMENT_3D('',#74915,#40680,#40681);
#35101=AXIS2_PLACEMENT_3D('',#74917,#40682,#40683);
#35102=AXIS2_PLACEMENT_3D('',#74919,#40685,#40686);
#35103=AXIS2_PLACEMENT_3D('',#74921,#40687,#40688);
#35104=AXIS2_PLACEMENT_3D('',#74924,#40690,#40691);
#35105=AXIS2_PLACEMENT_3D('',#74926,#40692,#40693);
#35106=AXIS2_PLACEMENT_3D('',#74928,#40694,#40695);
#35107=AXIS2_PLACEMENT_3D('',#74929,#40696,#40697);
#35108=AXIS2_PLACEMENT_3D('',#74930,#40698,#40699);
#35109=AXIS2_PLACEMENT_3D('',#74933,#40701,#40702);
#35110=AXIS2_PLACEMENT_3D('',#74934,#40703,#40704);
#35111=AXIS2_PLACEMENT_3D('',#74938,#40707,#40708);
#35112=AXIS2_PLACEMENT_3D('',#74940,#40709,#40710);
#35113=AXIS2_PLACEMENT_3D('',#74942,#40712,#40713);
#35114=AXIS2_PLACEMENT_3D('',#74944,#40714,#40715);
#35115=AXIS2_PLACEMENT_3D('',#74946,#40717,#40718);
#35116=AXIS2_PLACEMENT_3D('',#74948,#40719,#40720);
#35117=AXIS2_PLACEMENT_3D('',#74950,#40722,#40723);
#35118=AXIS2_PLACEMENT_3D('',#74952,#40724,#40725);
#35119=AXIS2_PLACEMENT_3D('',#74954,#40727,#40728);
#35120=AXIS2_PLACEMENT_3D('',#74957,#40730,#40731);
#35121=AXIS2_PLACEMENT_3D('',#74958,#40732,#40733);
#35122=AXIS2_PLACEMENT_3D('',#74960,#40734,#40735);
#35123=AXIS2_PLACEMENT_3D('',#74962,#40737,#40738);
#35124=AXIS2_PLACEMENT_3D('',#74964,#40740,#40741);
#35125=AXIS2_PLACEMENT_3D('',#74968,#40743,#40744);
#35126=AXIS2_PLACEMENT_3D('',#74970,#40746,#40747);
#35127=AXIS2_PLACEMENT_3D('',#74974,#40750,#40751);
#35128=AXIS2_PLACEMENT_3D('',#74980,#40755,#40756);
#35129=AXIS2_PLACEMENT_3D('',#74984,#40758,#40759);
#35130=AXIS2_PLACEMENT_3D('',#74985,#40760,#40761);
#35131=AXIS2_PLACEMENT_3D('',#74986,#40762,#40763);
#35132=AXIS2_PLACEMENT_3D('',#74990,#40766,#40767);
#35133=AXIS2_PLACEMENT_3D('',#74992,#40768,#40769);
#35134=AXIS2_PLACEMENT_3D('',#74994,#40771,#40772);
#35135=AXIS2_PLACEMENT_3D('',#74997,#40773,#40774);
#35136=AXIS2_PLACEMENT_3D('',#74999,#40775,#40776);
#35137=AXIS2_PLACEMENT_3D('',#75000,#40777,#40778);
#35138=AXIS2_PLACEMENT_3D('',#75001,#40779,#40780);
#35139=AXIS2_PLACEMENT_3D('',#75005,#40782,#40783);
#35140=AXIS2_PLACEMENT_3D('',#75006,#40784,#40785);
#35141=AXIS2_PLACEMENT_3D('',#75007,#40786,#40787);
#35142=AXIS2_PLACEMENT_3D('',#75008,#40788,#40789);
#35143=AXIS2_PLACEMENT_3D('',#75010,#40791,#40792);
#35144=AXIS2_PLACEMENT_3D('',#75014,#40795,#40796);
#35145=AXIS2_PLACEMENT_3D('',#75028,#40804,#40805);
#35146=AXIS2_PLACEMENT_3D('',#75030,#40806,#40807);
#35147=AXIS2_PLACEMENT_3D('',#75032,#40809,#40810);
#35148=AXIS2_PLACEMENT_3D('',#75044,#40817,#40818);
#35149=AXIS2_PLACEMENT_3D('',#75049,#40822,#40823);
#35150=AXIS2_PLACEMENT_3D('',#75050,#40824,#40825);
#35151=AXIS2_PLACEMENT_3D('',#75052,#40827,#40828);
#35152=AXIS2_PLACEMENT_3D('',#75056,#40831,#40832);
#35153=AXIS2_PLACEMENT_3D('',#75058,#40834,#40835);
#35154=AXIS2_PLACEMENT_3D('',#75062,#40838,#40839);
#35155=AXIS2_PLACEMENT_3D('',#75076,#40847,#40848);
#35156=AXIS2_PLACEMENT_3D('',#75078,#40849,#40850);
#35157=AXIS2_PLACEMENT_3D('',#75080,#40852,#40853);
#35158=AXIS2_PLACEMENT_3D('',#75092,#40860,#40861);
#35159=AXIS2_PLACEMENT_3D('',#75097,#40864,#40865);
#35160=AXIS2_PLACEMENT_3D('',#75098,#40866,#40867);
#35161=AXIS2_PLACEMENT_3D('',#75109,#40868,#40869);
#35162=AXIS2_PLACEMENT_3D('',#75120,#40870,#40871);
#35163=AXIS2_PLACEMENT_3D('',#75129,#40873,#40874);
#35164=AXIS2_PLACEMENT_3D('',#75138,#40875,#40876);
#35165=AXIS2_PLACEMENT_3D('',#75153,#40878,#40879);
#35166=AXIS2_PLACEMENT_3D('',#75154,#40880,#40881);
#35167=AXIS2_PLACEMENT_3D('',#75169,#40884,#40885);
#35168=AXIS2_PLACEMENT_3D('',#75170,#40886,#40887);
#35169=AXIS2_PLACEMENT_3D('',#75171,#40888,#40889);
#35170=AXIS2_PLACEMENT_3D('',#75179,#40890,#40891);
#35171=AXIS2_PLACEMENT_3D('',#75180,#40892,#40893);
#35172=AXIS2_PLACEMENT_3D('',#75181,#40894,#40895);
#35173=AXIS2_PLACEMENT_3D('',#75182,#40896,#40897);
#35174=AXIS2_PLACEMENT_3D('',#75183,#40898,#40899);
#35175=AXIS2_PLACEMENT_3D('',#75186,#40901,#40902);
#35176=AXIS2_PLACEMENT_3D('',#75187,#40903,#40904);
#35177=AXIS2_PLACEMENT_3D('',#75188,#40905,#40906);
#35178=AXIS2_PLACEMENT_3D('',#75189,#40907,#40908);
#35179=AXIS2_PLACEMENT_3D('',#75190,#40909,#40910);
#35180=AXIS2_PLACEMENT_3D('',#75192,#40911,#40912);
#35181=AXIS2_PLACEMENT_3D('',#75193,#40913,#40914);
#35182=AXIS2_PLACEMENT_3D('',#75194,#40915,#40916);
#35183=AXIS2_PLACEMENT_3D('',#75197,#40917,#40918);
#35184=AXIS2_PLACEMENT_3D('',#75199,#40919,#40920);
#35185=AXIS2_PLACEMENT_3D('',#75201,#40921,#40922);
#35186=AXIS2_PLACEMENT_3D('',#75203,#40923,#40924);
#35187=AXIS2_PLACEMENT_3D('',#75205,#40925,#40926);
#35188=AXIS2_PLACEMENT_3D('',#75209,#40928,#40929);
#35189=AXIS2_PLACEMENT_3D('',#75211,#40930,#40931);
#35190=AXIS2_PLACEMENT_3D('',#75214,#40933,#40934);
#35191=AXIS2_PLACEMENT_3D('',#75216,#40935,#40936);
#35192=AXIS2_PLACEMENT_3D('',#75217,#40937,#40938);
#35193=AXIS2_PLACEMENT_3D('',#75218,#40939,#40940);
#35194=AXIS2_PLACEMENT_3D('',#75219,#40941,#40942);
#35195=AXIS2_PLACEMENT_3D('',#75222,#40944,#40945);
#35196=AXIS2_PLACEMENT_3D('',#75223,#40946,#40947);
#35197=AXIS2_PLACEMENT_3D('',#75224,#40948,#40949);
#35198=AXIS2_PLACEMENT_3D('',#75226,#40950,#40951);
#35199=AXIS2_PLACEMENT_3D('',#75227,#40952,#40953);
#35200=AXIS2_PLACEMENT_3D('',#75228,#40954,#40955);
#35201=AXIS2_PLACEMENT_3D('',#75241,#40957,#40958);
#35202=AXIS2_PLACEMENT_3D('',#75243,#40959,#40960);
#35203=AXIS2_PLACEMENT_3D('',#75254,#40961,#40962);
#35204=AXIS2_PLACEMENT_3D('',#75255,#40963,#40964);
#35205=AXIS2_PLACEMENT_3D('',#75259,#40966,#40967);
#35206=AXIS2_PLACEMENT_3D('',#75260,#40968,#40969);
#35207=AXIS2_PLACEMENT_3D('',#75261,#40970,#40971);
#35208=AXIS2_PLACEMENT_3D('',#75264,#40972,#40973);
#35209=AXIS2_PLACEMENT_3D('',#75268,#40975,#40976);
#35210=AXIS2_PLACEMENT_3D('',#75270,#40978,#40979);
#35211=AXIS2_PLACEMENT_3D('',#75275,#40981,#40982);
#35212=AXIS2_PLACEMENT_3D('',#75278,#40984,#40985);
#35213=AXIS2_PLACEMENT_3D('',#75279,#40986,#40987);
#35214=AXIS2_PLACEMENT_3D('',#75284,#40989,#40990);
#35215=AXIS2_PLACEMENT_3D('',#75287,#40992,#40993);
#35216=AXIS2_PLACEMENT_3D('',#75288,#40994,#40995);
#35217=AXIS2_PLACEMENT_3D('',#75291,#40996,#40997);
#35218=AXIS2_PLACEMENT_3D('',#75295,#40999,#41000);
#35219=AXIS2_PLACEMENT_3D('',#75297,#41002,#41003);
#35220=AXIS2_PLACEMENT_3D('',#75301,#41005,#41006);
#35221=AXIS2_PLACEMENT_3D('',#75302,#41007,#41008);
#35222=AXIS2_PLACEMENT_3D('',#75303,#41009,#41010);
#35223=AXIS2_PLACEMENT_3D('',#75306,#41013,#41014);
#35224=AXIS2_PLACEMENT_3D('',#75307,#41015,#41016);
#35225=AXIS2_PLACEMENT_3D('',#75308,#41017,#41018);
#35226=AXIS2_PLACEMENT_3D('',#75309,#41019,#41020);
#35227=AXIS2_PLACEMENT_3D('',#75324,#41022,#41023);
#35228=AXIS2_PLACEMENT_3D('',#75327,#41025,#41026);
#35229=AXIS2_PLACEMENT_3D('',#75328,#41027,#41028);
#35230=AXIS2_PLACEMENT_3D('',#75331,#41029,#41030);
#35231=AXIS2_PLACEMENT_3D('',#75333,#41031,#41032);
#35232=AXIS2_PLACEMENT_3D('',#75367,#41035,#41036);
#35233=AXIS2_PLACEMENT_3D('',#75368,#41037,#41038);
#35234=AXIS2_PLACEMENT_3D('',#75372,#41040,#41041);
#35235=AXIS2_PLACEMENT_3D('',#75376,#41043,#41044);
#35236=AXIS2_PLACEMENT_3D('',#75380,#41046,#41047);
#35237=AXIS2_PLACEMENT_3D('',#75383,#41049,#41050);
#35238=AXIS2_PLACEMENT_3D('',#75385,#41051,#41052);
#35239=AXIS2_PLACEMENT_3D('',#75389,#41054,#41055);
#35240=AXIS2_PLACEMENT_3D('',#75393,#41057,#41058);
#35241=AXIS2_PLACEMENT_3D('',#75398,#41061,#41062);
#35242=AXIS2_PLACEMENT_3D('',#75400,#41063,#41064);
#35243=AXIS2_PLACEMENT_3D('',#75439,#41065,#41066);
#35244=AXIS2_PLACEMENT_3D('',#75442,#41068,#41069);
#35245=AXIS2_PLACEMENT_3D('',#75443,#41070,#41071);
#35246=AXIS2_PLACEMENT_3D('',#75447,#41073,#41074);
#35247=AXIS2_PLACEMENT_3D('',#75449,#41076,#41077);
#35248=AXIS2_PLACEMENT_3D('',#75454,#41080,#41081);
#35249=AXIS2_PLACEMENT_3D('',#75455,#41082,#41083);
#35250=AXIS2_PLACEMENT_3D('',#75460,#41085,#41086);
#35251=AXIS2_PLACEMENT_3D('',#75463,#41088,#41089);
#35252=AXIS2_PLACEMENT_3D('',#75464,#41090,#41091);
#35253=AXIS2_PLACEMENT_3D('',#75467,#41092,#41093);
#35254=AXIS2_PLACEMENT_3D('',#75471,#41095,#41096);
#35255=AXIS2_PLACEMENT_3D('',#75473,#41098,#41099);
#35256=AXIS2_PLACEMENT_3D('',#75477,#41101,#41102);
#35257=AXIS2_PLACEMENT_3D('',#75478,#41103,#41104);
#35258=AXIS2_PLACEMENT_3D('',#75479,#41105,#41106);
#35259=AXIS2_PLACEMENT_3D('',#75480,#41107,#41108);
#35260=AXIS2_PLACEMENT_3D('',#75481,#41109,#41110);
#35261=AXIS2_PLACEMENT_3D('',#75483,#41112,#41113);
#35262=AXIS2_PLACEMENT_3D('',#75484,#41114,#41115);
#35263=AXIS2_PLACEMENT_3D('',#75485,#41116,#41117);
#35264=AXIS2_PLACEMENT_3D('',#75486,#41118,#41119);
#35265=AXIS2_PLACEMENT_3D('',#75488,#41121,#41122);
#35266=AXIS2_PLACEMENT_3D('',#75490,#41124,#41125);
#35267=AXIS2_PLACEMENT_3D('',#75494,#41127,#41128);
#35268=AXIS2_PLACEMENT_3D('',#75506,#41130,#41131);
#35269=AXIS2_PLACEMENT_3D('',#75510,#41133,#41134);
#35270=AXIS2_PLACEMENT_3D('',#75512,#41135,#41136);
#35271=AXIS2_PLACEMENT_3D('',#75543,#41138,#41139);
#35272=AXIS2_PLACEMENT_3D('',#75545,#41140,#41141);
#35273=AXIS2_PLACEMENT_3D('',#75549,#41143,#41144);
#35274=AXIS2_PLACEMENT_3D('',#75553,#41146,#41147);
#35275=AXIS2_PLACEMENT_3D('',#75597,#41150,#41151);
#35276=AXIS2_PLACEMENT_3D('',#75599,#41152,#41153);
#35277=AXIS2_PLACEMENT_3D('',#75604,#41156,#41157);
#35278=AXIS2_PLACEMENT_3D('',#75608,#41159,#41160);
#35279=AXIS2_PLACEMENT_3D('',#75611,#41162,#41163);
#35280=AXIS2_PLACEMENT_3D('',#75612,#41164,#41165);
#35281=AXIS2_PLACEMENT_3D('',#75614,#41166,#41167);
#35282=AXIS2_PLACEMENT_3D('',#75615,#41168,#41169);
#35283=AXIS2_PLACEMENT_3D('',#75619,#41171,#41172);
#35284=AXIS2_PLACEMENT_3D('',#75621,#41174,#41175);
#35285=AXIS2_PLACEMENT_3D('',#75623,#41176,#41177);
#35286=AXIS2_PLACEMENT_3D('',#75625,#41179,#41180);
#35287=AXIS2_PLACEMENT_3D('',#75627,#41181,#41182);
#35288=AXIS2_PLACEMENT_3D('',#75629,#41184,#41185);
#35289=AXIS2_PLACEMENT_3D('',#75632,#41187,#41188);
#35290=AXIS2_PLACEMENT_3D('',#75633,#41189,#41190);
#35291=AXIS2_PLACEMENT_3D('',#75635,#41191,#41192);
#35292=AXIS2_PLACEMENT_3D('',#75637,#41194,#41195);
#35293=AXIS2_PLACEMENT_3D('',#75641,#41198,#41199);
#35294=AXIS2_PLACEMENT_3D('',#75643,#41200,#41201);
#35295=AXIS2_PLACEMENT_3D('',#75645,#41203,#41204);
#35296=AXIS2_PLACEMENT_3D('',#75647,#41205,#41206);
#35297=AXIS2_PLACEMENT_3D('',#75649,#41208,#41209);
#35298=AXIS2_PLACEMENT_3D('',#75651,#41211,#41212);
#35299=AXIS2_PLACEMENT_3D('',#75654,#41214,#41215);
#35300=AXIS2_PLACEMENT_3D('',#75655,#41216,#41217);
#35301=AXIS2_PLACEMENT_3D('',#75657,#41218,#41219);
#35302=AXIS2_PLACEMENT_3D('',#75659,#41221,#41222);
#35303=AXIS2_PLACEMENT_3D('',#75661,#41223,#41224);
#35304=AXIS2_PLACEMENT_3D('',#75662,#41225,#41226);
#35305=AXIS2_PLACEMENT_3D('',#75665,#41227,#41228);
#35306=AXIS2_PLACEMENT_3D('',#75668,#41231,#41232);
#35307=AXIS2_PLACEMENT_3D('',#75670,#41233,#41234);
#35308=AXIS2_PLACEMENT_3D('',#75867,#41243,#41244);
#35309=AXIS2_PLACEMENT_3D('',#75869,#41245,#41246);
#35310=AXIS2_PLACEMENT_3D('',#75871,#41248,#41249);
#35311=AXIS2_PLACEMENT_3D('',#75874,#41250,#41251);
#35312=AXIS2_PLACEMENT_3D('',#76072,#41261,#41262);
#35313=AXIS2_PLACEMENT_3D('',#76074,#41263,#41264);
#35314=AXIS2_PLACEMENT_3D('',#76076,#41266,#41267);
#35315=AXIS2_PLACEMENT_3D('',#76078,#41268,#41269);
#35316=AXIS2_PLACEMENT_3D('',#76080,#41271,#41272);
#35317=AXIS2_PLACEMENT_3D('',#76082,#41273,#41274);
#35318=AXIS2_PLACEMENT_3D('',#76084,#41276,#41277);
#35319=AXIS2_PLACEMENT_3D('',#76086,#41278,#41279);
#35320=AXIS2_PLACEMENT_3D('',#76090,#41281,#41282);
#35321=AXIS2_PLACEMENT_3D('',#76092,#41283,#41284);
#35322=AXIS2_PLACEMENT_3D('',#76094,#41286,#41287);
#35323=AXIS2_PLACEMENT_3D('',#76096,#41288,#41289);
#35324=AXIS2_PLACEMENT_3D('',#76097,#41290,#41291);
#35325=AXIS2_PLACEMENT_3D('',#76099,#41292,#41293);
#35326=AXIS2_PLACEMENT_3D('',#76100,#41294,#41295);
#35327=AXIS2_PLACEMENT_3D('',#76103,#41297,#41298);
#35328=AXIS2_PLACEMENT_3D('',#76104,#41299,#41300);
#35329=AXIS2_PLACEMENT_3D('',#76105,#41301,#41302);
#35330=AXIS2_PLACEMENT_3D('',#76109,#41304,#41305);
#35331=AXIS2_PLACEMENT_3D('',#76110,#41306,#41307);
#35332=AXIS2_PLACEMENT_3D('',#76111,#41308,#41309);
#35333=AXIS2_PLACEMENT_3D('',#76124,#41313,#41314);
#35334=AXIS2_PLACEMENT_3D('',#76126,#41315,#41316);
#35335=AXIS2_PLACEMENT_3D('',#76128,#41317,#41318);
#35336=AXIS2_PLACEMENT_3D('',#76130,#41320,#41321);
#35337=AXIS2_PLACEMENT_3D('',#76132,#41322,#41323);
#35338=AXIS2_PLACEMENT_3D('',#76134,#41324,#41325);
#35339=AXIS2_PLACEMENT_3D('',#76136,#41327,#41328);
#35340=AXIS2_PLACEMENT_3D('',#76142,#41332,#41333);
#35341=AXIS2_PLACEMENT_3D('',#76146,#41335,#41336);
#35342=AXIS2_PLACEMENT_3D('',#76148,#41337,#41338);
#35343=AXIS2_PLACEMENT_3D('',#76150,#41339,#41340);
#35344=AXIS2_PLACEMENT_3D('',#76152,#41341,#41342);
#35345=AXIS2_PLACEMENT_3D('',#76154,#41343,#41344);
#35346=AXIS2_PLACEMENT_3D('',#76156,#41345,#41346);
#35347=AXIS2_PLACEMENT_3D('',#76157,#41347,#41348);
#35348=AXIS2_PLACEMENT_3D('',#76158,#41349,#41350);
#35349=AXIS2_PLACEMENT_3D('',#76161,#41351,#41352);
#35350=AXIS2_PLACEMENT_3D('',#76164,#41354,#41355);
#35351=AXIS2_PLACEMENT_3D('',#76166,#41356,#41357);
#35352=AXIS2_PLACEMENT_3D('',#76168,#41358,#41359);
#35353=AXIS2_PLACEMENT_3D('',#76170,#41360,#41361);
#35354=AXIS2_PLACEMENT_3D('',#76172,#41362,#41363);
#35355=AXIS2_PLACEMENT_3D('',#76173,#41364,#41365);
#35356=AXIS2_PLACEMENT_3D('',#76174,#41366,#41367);
#35357=AXIS2_PLACEMENT_3D('',#76175,#41368,#41369);
#35358=AXIS2_PLACEMENT_3D('',#76178,#41370,#41371);
#35359=AXIS2_PLACEMENT_3D('',#76182,#41373,#41374);
#35360=AXIS2_PLACEMENT_3D('',#76184,#41376,#41377);
#35361=AXIS2_PLACEMENT_3D('',#76188,#41379,#41380);
#35362=AXIS2_PLACEMENT_3D('',#76189,#41381,#41382);
#35363=AXIS2_PLACEMENT_3D('',#76367,#41386,#41387);
#35364=AXIS2_PLACEMENT_3D('',#76369,#41388,#41389);
#35365=AXIS2_PLACEMENT_3D('',#76371,#41390,#41391);
#35366=AXIS2_PLACEMENT_3D('',#76550,#41396,#41397);
#35367=AXIS2_PLACEMENT_3D('',#76554,#41399,#41400);
#35368=AXIS2_PLACEMENT_3D('',#76555,#41401,#41402);
#35369=AXIS2_PLACEMENT_3D('',#76556,#41403,#41404);
#35370=AXIS2_PLACEMENT_3D('',#76557,#41405,#41406);
#35371=AXIS2_PLACEMENT_3D('',#76558,#41407,#41408);
#35372=AXIS2_PLACEMENT_3D('',#76559,#41409,#41410);
#35373=AXIS2_PLACEMENT_3D('',#76561,#41411,#41412);
#35374=AXIS2_PLACEMENT_3D('',#76562,#41413,#41414);
#35375=AXIS2_PLACEMENT_3D('',#76563,#41415,#41416);
#35376=AXIS2_PLACEMENT_3D('',#76572,#41417,#41418);
#35377=AXIS2_PLACEMENT_3D('',#76574,#41419,#41420);
#35378=AXIS2_PLACEMENT_3D('',#76581,#41421,#41422);
#35379=AXIS2_PLACEMENT_3D('',#76617,#41425,#41426);
#35380=AXIS2_PLACEMENT_3D('',#76633,#41427,#41428);
#35381=AXIS2_PLACEMENT_3D('',#76659,#41429,#41430);
#35382=AXIS2_PLACEMENT_3D('',#76688,#41433,#41434);
#35383=AXIS2_PLACEMENT_3D('',#76690,#41435,#41436);
#35384=AXIS2_PLACEMENT_3D('',#76692,#41437,#41438);
#35385=AXIS2_PLACEMENT_3D('',#76713,#41439,#41440);
#35386=AXIS2_PLACEMENT_3D('',#76718,#41441,#41442);
#35387=AXIS2_PLACEMENT_3D('',#76719,#41443,#41444);
#35388=AXIS2_PLACEMENT_3D('',#76757,#41445,#41446);
#35389=AXIS2_PLACEMENT_3D('',#76758,#41447,#41448);
#35390=AXIS2_PLACEMENT_3D('',#76774,#41449,#41450);
#35391=AXIS2_PLACEMENT_3D('',#76783,#41451,#41452);
#35392=AXIS2_PLACEMENT_3D('',#76787,#41454,#41455);
#35393=AXIS2_PLACEMENT_3D('',#76788,#41456,#41457);
#35394=AXIS2_PLACEMENT_3D('',#76789,#41458,#41459);
#35395=AXIS2_PLACEMENT_3D('',#76805,#41460,#41461);
#35396=AXIS2_PLACEMENT_3D('',#76807,#41462,#41463);
#35397=AXIS2_PLACEMENT_3D('',#76809,#41464,#41465);
#35398=AXIS2_PLACEMENT_3D('',#76813,#41467,#41468);
#35399=AXIS2_PLACEMENT_3D('',#76820,#41469,#41470);
#35400=AXIS2_PLACEMENT_3D('',#76835,#41471,#41472);
#35401=AXIS2_PLACEMENT_3D('',#76836,#41473,#41474);
#35402=AXIS2_PLACEMENT_3D('',#76843,#41475,#41476);
#35403=AXIS2_PLACEMENT_3D('',#76850,#41477,#41478);
#35404=AXIS2_PLACEMENT_3D('',#76851,#41479,#41480);
#35405=AXIS2_PLACEMENT_3D('',#76853,#41481,#41482);
#35406=AXIS2_PLACEMENT_3D('',#76890,#41483,#41484);
#35407=AXIS2_PLACEMENT_3D('',#76916,#41485,#41486);
#35408=AXIS2_PLACEMENT_3D('',#76918,#41487,#41488);
#35409=AXIS2_PLACEMENT_3D('',#76922,#41490,#41491);
#35410=AXIS2_PLACEMENT_3D('',#76924,#41492,#41493);
#35411=AXIS2_PLACEMENT_3D('',#76980,#41494,#41495);
#35412=AXIS2_PLACEMENT_3D('',#77010,#41496,#41497);
#35413=AXIS2_PLACEMENT_3D('',#77011,#41498,#41499);
#35414=AXIS2_PLACEMENT_3D('',#77014,#41500,#41501);
#35415=AXIS2_PLACEMENT_3D('',#77016,#41502,#41503);
#35416=AXIS2_PLACEMENT_3D('',#77020,#41505,#41506);
#35417=AXIS2_PLACEMENT_3D('',#77022,#41507,#41508);
#35418=AXIS2_PLACEMENT_3D('',#77071,#41509,#41510);
#35419=AXIS2_PLACEMENT_3D('',#77073,#41511,#41512);
#35420=AXIS2_PLACEMENT_3D('',#77075,#41514,#41515);
#35421=AXIS2_PLACEMENT_3D('',#77076,#41516,#41517);
#35422=AXIS2_PLACEMENT_3D('',#77133,#41519,#41520);
#35423=AXIS2_PLACEMENT_3D('',#77164,#41521,#41522);
#35424=AXIS2_PLACEMENT_3D('',#77166,#41523,#41524);
#35425=AXIS2_PLACEMENT_3D('',#77195,#41525,#41526);
#35426=AXIS2_PLACEMENT_3D('',#77197,#41527,#41528);
#35427=AXIS2_PLACEMENT_3D('',#77216,#41529,#41530);
#35428=AXIS2_PLACEMENT_3D('',#77294,#41534,#41535);
#35429=AXIS2_PLACEMENT_3D('',#77296,#41536,#41537);
#35430=AXIS2_PLACEMENT_3D('',#77461,#41544,#41545);
#35431=AXIS2_PLACEMENT_3D('',#77463,#41546,#41547);
#35432=AXIS2_PLACEMENT_3D('',#77465,#41549,#41550);
#35433=AXIS2_PLACEMENT_3D('',#77469,#41553,#41554);
#35434=AXIS2_PLACEMENT_3D('',#77470,#41555,#41556);
#35435=AXIS2_PLACEMENT_3D('',#77551,#41561,#41562);
#35436=AXIS2_PLACEMENT_3D('',#77553,#41563,#41564);
#35437=AXIS2_PLACEMENT_3D('',#77555,#41566,#41567);
#35438=AXIS2_PLACEMENT_3D('',#77559,#41570,#41571);
#35439=AXIS2_PLACEMENT_3D('',#77560,#41572,#41573);
#35440=AXIS2_PLACEMENT_3D('',#77561,#41574,#41575);
#35441=AXIS2_PLACEMENT_3D('',#77563,#41576,#41577);
#35442=AXIS2_PLACEMENT_3D('',#77757,#41585,#41586);
#35443=AXIS2_PLACEMENT_3D('',#77759,#41587,#41588);
#35444=AXIS2_PLACEMENT_3D('',#77761,#41590,#41591);
#35445=AXIS2_PLACEMENT_3D('',#77764,#41593,#41594);
#35446=AXIS2_PLACEMENT_3D('',#77765,#41595,#41596);
#35447=AXIS2_PLACEMENT_3D('',#77769,#41599,#41600);
#35448=AXIS2_PLACEMENT_3D('',#77772,#41602,#41603);
#35449=AXIS2_PLACEMENT_3D('',#77773,#41604,#41605);
#35450=AXIS2_PLACEMENT_3D('',#77775,#41606,#41607);
#35451=AXIS2_PLACEMENT_3D('',#77906,#41613,#41614);
#35452=AXIS2_PLACEMENT_3D('',#77962,#41618,#41619);
#35453=AXIS2_PLACEMENT_3D('',#77964,#41621,#41622);
#35454=AXIS2_PLACEMENT_3D('',#77965,#41623,#41624);
#35455=AXIS2_PLACEMENT_3D('',#77968,#41625,#41626);
#35456=AXIS2_PLACEMENT_3D('',#77971,#41629,#41630);
#35457=AXIS2_PLACEMENT_3D('',#77973,#41631,#41632);
#35458=AXIS2_PLACEMENT_3D('',#77975,#41634,#41635);
#35459=AXIS2_PLACEMENT_3D('',#77979,#41638,#41639);
#35460=AXIS2_PLACEMENT_3D('',#77981,#41640,#41641);
#35461=AXIS2_PLACEMENT_3D('',#77983,#41643,#41644);
#35462=AXIS2_PLACEMENT_3D('',#77985,#41645,#41646);
#35463=AXIS2_PLACEMENT_3D('',#78128,#41651,#41652);
#35464=AXIS2_PLACEMENT_3D('',#78129,#41653,#41654);
#35465=AXIS2_PLACEMENT_3D('',#78130,#41655,#41656);
#35466=AXIS2_PLACEMENT_3D('',#78132,#41658,#41659);
#35467=AXIS2_PLACEMENT_3D('',#78134,#41661,#41662);
#35468=AXIS2_PLACEMENT_3D('',#78136,#41664,#41665);
#35469=AXIS2_PLACEMENT_3D('',#78138,#41667,#41668);
#35470=AXIS2_PLACEMENT_3D('',#78146,#41673,#41674);
#35471=AXIS2_PLACEMENT_3D('',#78156,#41680,#41681);
#35472=AXIS2_PLACEMENT_3D('',#78166,#41687,#41688);
#35473=AXIS2_PLACEMENT_3D('',#78174,#41693,#41694);
#35474=AXIS2_PLACEMENT_3D('',#78182,#41699,#41700);
#35475=AXIS2_PLACEMENT_3D('',#78192,#41706,#41707);
#35476=AXIS2_PLACEMENT_3D('',#78202,#41713,#41714);
#35477=AXIS2_PLACEMENT_3D('',#78210,#41719,#41720);
#35478=AXIS2_PLACEMENT_3D('',#78211,#41721,#41722);
#35479=AXIS2_PLACEMENT_3D('',#78212,#41723,#41724);
#35480=AXIS2_PLACEMENT_3D('',#78215,#41726,#41727);
#35481=AXIS2_PLACEMENT_3D('',#78216,#41728,#41729);
#35482=AXIS2_PLACEMENT_3D('',#78218,#41730,#41731);
#35483=AXIS2_PLACEMENT_3D('',#78221,#41733,#41734);
#35484=AXIS2_PLACEMENT_3D('',#78222,#41735,#41736);
#35485=AXIS2_PLACEMENT_3D('',#78223,#41737,#41738);
#35486=AXIS2_PLACEMENT_3D('',#78225,#41739,#41740);
#35487=AXIS2_PLACEMENT_3D('',#78228,#41742,#41743);
#35488=AXIS2_PLACEMENT_3D('',#78230,#41744,#41745);
#35489=AXIS2_PLACEMENT_3D('',#78233,#41747,#41748);
#35490=AXIS2_PLACEMENT_3D('',#78236,#41750,#41751);
#35491=AXIS2_PLACEMENT_3D('',#78238,#41752,#41753);
#35492=AXIS2_PLACEMENT_3D('',#78241,#41755,#41756);
#35493=AXIS2_PLACEMENT_3D('',#78244,#41758,#41759);
#35494=AXIS2_PLACEMENT_3D('',#78245,#41760,#41761);
#35495=AXIS2_PLACEMENT_3D('',#78246,#41762,#41763);
#35496=AXIS2_PLACEMENT_3D('',#78247,#41764,#41765);
#35497=AXIS2_PLACEMENT_3D('',#78249,#41766,#41767);
#35498=AXIS2_PLACEMENT_3D('',#78251,#41769,#41770);
#35499=AXIS2_PLACEMENT_3D('',#78253,#41771,#41772);
#35500=AXIS2_PLACEMENT_3D('',#78255,#41773,#41774);
#35501=AXIS2_PLACEMENT_3D('',#78257,#41776,#41777);
#35502=AXIS2_PLACEMENT_3D('',#78258,#41778,#41779);
#35503=AXIS2_PLACEMENT_3D('',#78259,#41780,#41781);
#35504=AXIS2_PLACEMENT_3D('',#78260,#41782,#41783);
#35505=AXIS2_PLACEMENT_3D('',#78261,#41784,#41785);
#35506=AXIS2_PLACEMENT_3D('',#78263,#41786,#41787);
#35507=AXIS2_PLACEMENT_3D('',#78265,#41789,#41790);
#35508=AXIS2_PLACEMENT_3D('',#78266,#41791,#41792);
#35509=AXIS2_PLACEMENT_3D('',#78267,#41793,#41794);
#35510=AXIS2_PLACEMENT_3D('',#78269,#41795,#41796);
#35511=AXIS2_PLACEMENT_3D('',#78270,#41797,#41798);
#35512=AXIS2_PLACEMENT_3D('',#78271,#41799,#41800);
#35513=AXIS2_PLACEMENT_3D('',#78272,#41801,#41802);
#35514=AXIS2_PLACEMENT_3D('',#78273,#41803,#41804);
#35515=AXIS2_PLACEMENT_3D('',#78274,#41805,#41806);
#35516=AXIS2_PLACEMENT_3D('',#78275,#41807,#41808);
#35517=AXIS2_PLACEMENT_3D('',#78283,#41812,#41813);
#35518=AXIS2_PLACEMENT_3D('',#78285,#41814,#41815);
#35519=AXIS2_PLACEMENT_3D('',#78287,#41816,#41817);
#35520=AXIS2_PLACEMENT_3D('',#78291,#41820,#41821);
#35521=AXIS2_PLACEMENT_3D('',#78293,#41822,#41823);
#35522=AXIS2_PLACEMENT_3D('',#78295,#41825,#41826);
#35523=AXIS2_PLACEMENT_3D('',#78296,#41827,#41828);
#35524=AXIS2_PLACEMENT_3D('',#78297,#41829,#41830);
#35525=AXIS2_PLACEMENT_3D('',#78298,#41831,#41832);
#35526=AXIS2_PLACEMENT_3D('',#78299,#41833,#41834);
#35527=AXIS2_PLACEMENT_3D('',#78300,#41835,#41836);
#35528=AXIS2_PLACEMENT_3D('',#78302,#41837,#41838);
#35529=AXIS2_PLACEMENT_3D('',#78303,#41839,#41840);
#35530=AXIS2_PLACEMENT_3D('',#78304,#41841,#41842);
#35531=AXIS2_PLACEMENT_3D('',#78307,#41844,#41845);
#35532=AXIS2_PLACEMENT_3D('',#78308,#41846,#41847);
#35533=AXIS2_PLACEMENT_3D('',#78309,#41848,#41849);
#35534=AXIS2_PLACEMENT_3D('',#78310,#41850,#41851);
#35535=AXIS2_PLACEMENT_3D('',#78311,#41852,#41853);
#35536=AXIS2_PLACEMENT_3D('',#78312,#41854,#41855);
#35537=AXIS2_PLACEMENT_3D('',#78313,#41856,#41857);
#35538=AXIS2_PLACEMENT_3D('',#78314,#41858,#41859);
#35539=AXIS2_PLACEMENT_3D('',#78315,#41860,#41861);
#35540=AXIS2_PLACEMENT_3D('',#78316,#41862,#41863);
#35541=AXIS2_PLACEMENT_3D('',#78317,#41864,#41865);
#35542=AXIS2_PLACEMENT_3D('',#78318,#41866,#41867);
#35543=AXIS2_PLACEMENT_3D('',#78319,#41868,#41869);
#35544=AXIS2_PLACEMENT_3D('',#78320,#41870,#41871);
#35545=AXIS2_PLACEMENT_3D('',#78321,#41872,#41873);
#35546=AXIS2_PLACEMENT_3D('',#78322,#41874,#41875);
#35547=AXIS2_PLACEMENT_3D('',#78324,#41877,#41878);
#35548=AXIS2_PLACEMENT_3D('',#78325,#41879,#41880);
#35549=AXIS2_PLACEMENT_3D('',#78327,#41882,#41883);
#35550=AXIS2_PLACEMENT_3D('',#78329,#41885,#41886);
#35551=AXIS2_PLACEMENT_3D('',#78330,#41887,#41888);
#35552=AXIS2_PLACEMENT_3D('',#78331,#41889,#41890);
#35553=AXIS2_PLACEMENT_3D('',#78332,#41891,#41892);
#35554=AXIS2_PLACEMENT_3D('',#78338,#41896,#41897);
#35555=AXIS2_PLACEMENT_3D('',#78340,#41898,#41899);
#35556=AXIS2_PLACEMENT_3D('',#78342,#41900,#41901);
#35557=AXIS2_PLACEMENT_3D('',#78344,#41903,#41904);
#35558=AXIS2_PLACEMENT_3D('',#78345,#41905,#41906);
#35559=AXIS2_PLACEMENT_3D('',#78346,#41907,#41908);
#35560=AXIS2_PLACEMENT_3D('',#78347,#41909,#41910);
#35561=AXIS2_PLACEMENT_3D('',#78348,#41911,#41912);
#35562=AXIS2_PLACEMENT_3D('',#78351,#41914,#41915);
#35563=AXIS2_PLACEMENT_3D('',#78352,#41916,#41917);
#35564=AXIS2_PLACEMENT_3D('',#78353,#41918,#41919);
#35565=AXIS2_PLACEMENT_3D('',#78354,#41920,#41921);
#35566=AXIS2_PLACEMENT_3D('',#78356,#41922,#41923);
#35567=AXIS2_PLACEMENT_3D('',#78357,#41924,#41925);
#35568=AXIS2_PLACEMENT_3D('',#78358,#41926,#41927);
#35569=AXIS2_PLACEMENT_3D('',#78361,#41929,#41930);
#35570=AXIS2_PLACEMENT_3D('',#78362,#41931,#41932);
#35571=AXIS2_PLACEMENT_3D('',#78363,#41933,#41934);
#35572=AXIS2_PLACEMENT_3D('',#78364,#41935,#41936);
#35573=AXIS2_PLACEMENT_3D('',#78372,#41940,#41941);
#35574=AXIS2_PLACEMENT_3D('',#78374,#41942,#41943);
#35575=AXIS2_PLACEMENT_3D('',#78376,#41944,#41945);
#35576=AXIS2_PLACEMENT_3D('',#78380,#41948,#41949);
#35577=AXIS2_PLACEMENT_3D('',#78382,#41950,#41951);
#35578=AXIS2_PLACEMENT_3D('',#78384,#41953,#41954);
#35579=AXIS2_PLACEMENT_3D('',#78386,#41955,#41956);
#35580=AXIS2_PLACEMENT_3D('',#78387,#41957,#41958);
#35581=AXIS2_PLACEMENT_3D('',#78388,#41959,#41960);
#35582=AXIS2_PLACEMENT_3D('',#78391,#41962,#41963);
#35583=AXIS2_PLACEMENT_3D('',#78392,#41964,#41965);
#35584=AXIS2_PLACEMENT_3D('',#78394,#41966,#41967);
#35585=AXIS2_PLACEMENT_3D('',#78395,#41968,#41969);
#35586=AXIS2_PLACEMENT_3D('',#78396,#41970,#41971);
#35587=AXIS2_PLACEMENT_3D('',#78399,#41973,#41974);
#35588=AXIS2_PLACEMENT_3D('',#78400,#41975,#41976);
#35589=AXIS2_PLACEMENT_3D('',#78402,#41977,#41978);
#35590=AXIS2_PLACEMENT_3D('',#78403,#41979,#41980);
#35591=AXIS2_PLACEMENT_3D('',#78404,#41981,#41982);
#35592=AXIS2_PLACEMENT_3D('',#78407,#41984,#41985);
#35593=AXIS2_PLACEMENT_3D('',#78408,#41986,#41987);
#35594=AXIS2_PLACEMENT_3D('',#78409,#41988,#41989);
#35595=AXIS2_PLACEMENT_3D('',#78410,#41990,#41991);
#35596=AXIS2_PLACEMENT_3D('',#78411,#41992,#41993);
#35597=AXIS2_PLACEMENT_3D('',#78412,#41994,#41995);
#35598=AXIS2_PLACEMENT_3D('',#78413,#41996,#41997);
#35599=AXIS2_PLACEMENT_3D('',#78415,#41998,#41999);
#35600=AXIS2_PLACEMENT_3D('',#78416,#42000,#42001);
#35601=AXIS2_PLACEMENT_3D('',#78417,#42002,#42003);
#35602=AXIS2_PLACEMENT_3D('',#78419,#42005,#42006);
#35603=AXIS2_PLACEMENT_3D('',#78421,#42008,#42009);
#35604=AXIS2_PLACEMENT_3D('',#78423,#42011,#42012);
#35605=AXIS2_PLACEMENT_3D('',#78425,#42014,#42015);
#35606=AXIS2_PLACEMENT_3D('',#78427,#42017,#42018);
#35607=AXIS2_PLACEMENT_3D('',#78429,#42020,#42021);
#35608=AXIS2_PLACEMENT_3D('',#78431,#42023,#42024);
#35609=AXIS2_PLACEMENT_3D('',#78433,#42026,#42027);
#35610=AXIS2_PLACEMENT_3D('',#78434,#42028,#42029);
#35611=AXIS2_PLACEMENT_3D('',#78436,#42031,#42032);
#35612=AXIS2_PLACEMENT_3D('',#78437,#42033,#42034);
#35613=AXIS2_PLACEMENT_3D('',#78439,#42035,#42036);
#35614=AXIS2_PLACEMENT_3D('',#78442,#42038,#42039);
#35615=AXIS2_PLACEMENT_3D('',#78443,#42040,#42041);
#35616=AXIS2_PLACEMENT_3D('',#78444,#42042,#42043);
#35617=AXIS2_PLACEMENT_3D('',#78445,#42044,#42045);
#35618=AXIS2_PLACEMENT_3D('',#78446,#42046,#42047);
#35619=AXIS2_PLACEMENT_3D('',#78447,#42048,#42049);
#35620=AXIS2_PLACEMENT_3D('',#78450,#42051,#42052);
#35621=AXIS2_PLACEMENT_3D('',#78451,#42053,#42054);
#35622=AXIS2_PLACEMENT_3D('',#78452,#42055,#42056);
#35623=AXIS2_PLACEMENT_3D('',#78453,#42057,#42058);
#35624=AXIS2_PLACEMENT_3D('',#78455,#42059,#42060);
#35625=AXIS2_PLACEMENT_3D('',#78456,#42061,#42062);
#35626=AXIS2_PLACEMENT_3D('',#78457,#42063,#42064);
#35627=AXIS2_PLACEMENT_3D('',#78458,#42065,#42066);
#35628=AXIS2_PLACEMENT_3D('',#78459,#42067,#42068);
#35629=AXIS2_PLACEMENT_3D('',#78460,#42069,#42070);
#35630=AXIS2_PLACEMENT_3D('',#78461,#42071,#42072);
#35631=AXIS2_PLACEMENT_3D('',#78467,#42075,#42076);
#35632=AXIS2_PLACEMENT_3D('',#78469,#42077,#42078);
#35633=AXIS2_PLACEMENT_3D('',#78471,#42079,#42080);
#35634=AXIS2_PLACEMENT_3D('',#78477,#42084,#42085);
#35635=AXIS2_PLACEMENT_3D('',#78479,#42086,#42087);
#35636=AXIS2_PLACEMENT_3D('',#78481,#42089,#42090);
#35637=AXIS2_PLACEMENT_3D('',#78482,#42091,#42092);
#35638=AXIS2_PLACEMENT_3D('',#78483,#42093,#42094);
#35639=AXIS2_PLACEMENT_3D('',#78484,#42095,#42096);
#35640=AXIS2_PLACEMENT_3D('',#78485,#42097,#42098);
#35641=AXIS2_PLACEMENT_3D('',#78486,#42099,#42100);
#35642=AXIS2_PLACEMENT_3D('',#78488,#42101,#42102);
#35643=AXIS2_PLACEMENT_3D('',#78489,#42103,#42104);
#35644=AXIS2_PLACEMENT_3D('',#78490,#42105,#42106);
#35645=AXIS2_PLACEMENT_3D('',#78492,#42107,#42108);
#35646=AXIS2_PLACEMENT_3D('',#78494,#42110,#42111);
#35647=AXIS2_PLACEMENT_3D('',#78495,#42112,#42113);
#35648=AXIS2_PLACEMENT_3D('',#78496,#42114,#42115);
#35649=AXIS2_PLACEMENT_3D('',#78497,#42116,#42117);
#35650=AXIS2_PLACEMENT_3D('',#78498,#42118,#42119);
#35651=AXIS2_PLACEMENT_3D('',#78499,#42120,#42121);
#35652=AXIS2_PLACEMENT_3D('',#78500,#42122,#42123);
#35653=AXIS2_PLACEMENT_3D('',#78501,#42124,#42125);
#35654=AXIS2_PLACEMENT_3D('',#78502,#42126,#42127);
#35655=AXIS2_PLACEMENT_3D('',#78503,#42128,#42129);
#35656=AXIS2_PLACEMENT_3D('',#78504,#42130,#42131);
#35657=AXIS2_PLACEMENT_3D('',#78505,#42132,#42133);
#35658=AXIS2_PLACEMENT_3D('',#78506,#42134,#42135);
#35659=AXIS2_PLACEMENT_3D('',#78507,#42136,#42137);
#35660=AXIS2_PLACEMENT_3D('',#78508,#42138,#42139);
#35661=AXIS2_PLACEMENT_3D('',#78510,#42141,#42142);
#35662=AXIS2_PLACEMENT_3D('',#78511,#42143,#42144);
#35663=AXIS2_PLACEMENT_3D('',#78513,#42146,#42147);
#35664=AXIS2_PLACEMENT_3D('',#78515,#42149,#42150);
#35665=AXIS2_PLACEMENT_3D('',#78516,#42151,#42152);
#35666=AXIS2_PLACEMENT_3D('',#78517,#42153,#42154);
#35667=AXIS2_PLACEMENT_3D('',#78518,#42155,#42156);
#35668=AXIS2_PLACEMENT_3D('',#78524,#42160,#42161);
#35669=AXIS2_PLACEMENT_3D('',#78526,#42162,#42163);
#35670=AXIS2_PLACEMENT_3D('',#78529,#42165,#42166);
#35671=AXIS2_PLACEMENT_3D('',#78530,#42167,#42168);
#35672=AXIS2_PLACEMENT_3D('',#78533,#42170,#42171);
#35673=AXIS2_PLACEMENT_3D('',#78534,#42172,#42173);
#35674=AXIS2_PLACEMENT_3D('',#78535,#42174,#42175);
#35675=AXIS2_PLACEMENT_3D('',#78536,#42176,#42177);
#35676=AXIS2_PLACEMENT_3D('',#78537,#42178,#42179);
#35677=AXIS2_PLACEMENT_3D('',#78538,#42180,#42181);
#35678=AXIS2_PLACEMENT_3D('',#78539,#42182,#42183);
#35679=AXIS2_PLACEMENT_3D('',#78540,#42184,#42185);
#35680=AXIS2_PLACEMENT_3D('',#78546,#42188,#42189);
#35681=AXIS2_PLACEMENT_3D('',#78548,#42190,#42191);
#35682=AXIS2_PLACEMENT_3D('',#78550,#42192,#42193);
#35683=AXIS2_PLACEMENT_3D('',#78557,#42197,#42198);
#35684=AXIS2_PLACEMENT_3D('',#78558,#42199,#42200);
#35685=AXIS2_PLACEMENT_3D('',#78560,#42201,#42202);
#35686=AXIS2_PLACEMENT_3D('',#78562,#42204,#42205);
#35687=AXIS2_PLACEMENT_3D('',#78564,#42206,#42207);
#35688=AXIS2_PLACEMENT_3D('',#78565,#42208,#42209);
#35689=AXIS2_PLACEMENT_3D('',#78566,#42210,#42211);
#35690=AXIS2_PLACEMENT_3D('',#78567,#42212,#42213);
#35691=AXIS2_PLACEMENT_3D('',#78568,#42214,#42215);
#35692=AXIS2_PLACEMENT_3D('',#78570,#42216,#42217);
#35693=AXIS2_PLACEMENT_3D('',#78571,#42218,#42219);
#35694=AXIS2_PLACEMENT_3D('',#78572,#42220,#42221);
#35695=AXIS2_PLACEMENT_3D('',#78574,#42222,#42223);
#35696=AXIS2_PLACEMENT_3D('',#78576,#42224,#42225);
#35697=AXIS2_PLACEMENT_3D('',#78578,#42227,#42228);
#35698=AXIS2_PLACEMENT_3D('',#78580,#42229,#42230);
#35699=AXIS2_PLACEMENT_3D('',#78581,#42231,#42232);
#35700=AXIS2_PLACEMENT_3D('',#78582,#42233,#42234);
#35701=AXIS2_PLACEMENT_3D('',#78584,#42235,#42236);
#35702=AXIS2_PLACEMENT_3D('',#78585,#42237,#42238);
#35703=AXIS2_PLACEMENT_3D('',#78586,#42239,#42240);
#35704=AXIS2_PLACEMENT_3D('',#78588,#42242,#42243);
#35705=AXIS2_PLACEMENT_3D('',#78590,#42244,#42245);
#35706=AXIS2_PLACEMENT_3D('',#78592,#42247,#42248);
#35707=AXIS2_PLACEMENT_3D('',#78593,#42249,#42250);
#35708=AXIS2_PLACEMENT_3D('',#78594,#42251,#42252);
#35709=AXIS2_PLACEMENT_3D('',#78595,#42253,#42254);
#35710=AXIS2_PLACEMENT_3D('',#78596,#42255,#42256);
#35711=AXIS2_PLACEMENT_3D('',#78597,#42257,#42258);
#35712=AXIS2_PLACEMENT_3D('',#78599,#42259,#42260);
#35713=AXIS2_PLACEMENT_3D('',#78600,#42261,#42262);
#35714=AXIS2_PLACEMENT_3D('',#78601,#42263,#42264);
#35715=AXIS2_PLACEMENT_3D('',#78603,#42266,#42267);
#35716=AXIS2_PLACEMENT_3D('',#78605,#42269,#42270);
#35717=AXIS2_PLACEMENT_3D('',#78607,#42272,#42273);
#35718=AXIS2_PLACEMENT_3D('',#78609,#42275,#42276);
#35719=AXIS2_PLACEMENT_3D('',#78612,#42279,#42280);
#35720=AXIS2_PLACEMENT_3D('',#78614,#42282,#42283);
#35721=AXIS2_PLACEMENT_3D('',#78616,#42285,#42286);
#35722=AXIS2_PLACEMENT_3D('',#78617,#42287,#42288);
#35723=AXIS2_PLACEMENT_3D('',#78619,#42290,#42291);
#35724=AXIS2_PLACEMENT_3D('',#78620,#42292,#42293);
#35725=AXIS2_PLACEMENT_3D('',#78622,#42295,#42296);
#40272=DIRECTION('axis',(0.,0.,1.));
#40273=DIRECTION('refdir',(1.,0.,0.));
#40274=DIRECTION('center_axis',(0.,1.,0.));
#40275=DIRECTION('ref_axis',(1.,0.,0.));
#40276=DIRECTION('',(0.,0.,-1.));
#40277=DIRECTION('center_axis',(0.,-1.,0.));
#40278=DIRECTION('ref_axis',(-0.256673183280288,0.,-0.966498255034516));
#40279=DIRECTION('center_axis',(0.,-1.,0.));
#40280=DIRECTION('ref_axis',(-0.280070575750354,0.,-0.959979412591158));
#40281=DIRECTION('',(0.,-1.,0.));
#40282=DIRECTION('',(0.,1.,0.));
#40283=DIRECTION('center_axis',(0.,-1.,0.));
#40284=DIRECTION('ref_axis',(1.,0.,0.));
#40285=DIRECTION('center_axis',(1.,0.,0.));
#40286=DIRECTION('ref_axis',(0.,1.,0.));
#40287=DIRECTION('',(0.,1.,0.));
#40288=DIRECTION('',(0.,0.,-1.));
#40289=DIRECTION('center_axis',(0.,1.,0.));
#40290=DIRECTION('ref_axis',(1.,0.,0.));
#40291=DIRECTION('center_axis',(0.,1.,0.));
#40292=DIRECTION('ref_axis',(1.,0.,0.));
#40293=DIRECTION('center_axis',(0.,1.,0.));
#40294=DIRECTION('ref_axis',(0.256673183280308,0.,-0.96649825503451));
#40295=DIRECTION('',(0.,0.,-1.));
#40296=DIRECTION('center_axis',(1.,0.,0.));
#40297=DIRECTION('ref_axis',(0.,1.,0.));
#40298=DIRECTION('',(0.,1.,0.));
#40299=DIRECTION('',(0.,0.,-1.));
#40300=DIRECTION('',(0.,1.,0.));
#40301=DIRECTION('center_axis',(0.,1.,0.));
#40302=DIRECTION('ref_axis',(0.280070575787534,0.,-0.959979412580311));
#40303=DIRECTION('',(0.,1.,0.));
#40304=DIRECTION('center_axis',(0.,1.,0.));
#40305=DIRECTION('ref_axis',(1.,0.,0.));
#40306=DIRECTION('center_axis',(0.,1.,0.));
#40307=DIRECTION('ref_axis',(1.,0.,0.));
#40308=DIRECTION('center_axis',(0.,1.,0.));
#40309=DIRECTION('ref_axis',(-6.12267139103014E-17,0.,1.));
#40310=DIRECTION('center_axis',(0.,-1.,0.));
#40311=DIRECTION('ref_axis',(1.,0.,0.));
#40312=DIRECTION('',(0.,1.,0.));
#40313=DIRECTION('center_axis',(0.,-1.,0.));
#40314=DIRECTION('ref_axis',(1.,0.,0.));
#40315=DIRECTION('center_axis',(0.,-1.,0.));
#40316=DIRECTION('ref_axis',(1.,0.,0.));
#40317=DIRECTION('',(0.,1.,0.));
#40318=DIRECTION('center_axis',(0.,-1.,0.));
#40319=DIRECTION('ref_axis',(2.83274710209661E-16,0.,1.));
#40320=DIRECTION('center_axis',(0.,-1.,0.));
#40321=DIRECTION('ref_axis',(1.,0.,0.));
#40322=DIRECTION('',(0.,1.,0.));
#40323=DIRECTION('center_axis',(0.,-1.,0.));
#40324=DIRECTION('ref_axis',(1.,0.,0.));
#40325=DIRECTION('',(0.,1.,0.));
#40326=DIRECTION('center_axis',(-0.341378619534878,0.,0.939925868419665));
#40327=DIRECTION('ref_axis',(0.,1.,0.));
#40328=DIRECTION('',(0.,1.,0.));
#40329=DIRECTION('',(0.939925868419665,0.,0.341378619534878));
#40330=DIRECTION('',(0.939925868419665,0.,0.341378619534878));
#40331=DIRECTION('',(0.,1.,0.));
#40332=DIRECTION('',(0.939925868419665,0.,0.341378619534878));
#40333=DIRECTION('center_axis',(0.,1.,0.));
#40334=DIRECTION('ref_axis',(1.,0.,0.));
#40335=DIRECTION('',(-1.,0.,0.));
#40336=DIRECTION('',(-1.,0.,0.));
#40337=DIRECTION('center_axis',(0.,1.,0.));
#40338=DIRECTION('ref_axis',(1.,0.,0.));
#40339=DIRECTION('',(1.,0.,0.));
#40340=DIRECTION('',(-1.,0.,0.));
#40341=DIRECTION('center_axis',(0.,-1.,0.));
#40342=DIRECTION('ref_axis',(1.,0.,0.));
#40343=DIRECTION('',(1.,0.,0.));
#40344=DIRECTION('',(-1.,0.,0.));
#40345=DIRECTION('center_axis',(0.,1.,0.));
#40346=DIRECTION('ref_axis',(1.,0.,0.));
#40347=DIRECTION('',(1.,0.,0.));
#40348=DIRECTION('',(1.,0.,0.));
#40349=DIRECTION('center_axis',(0.,1.,0.));
#40350=DIRECTION('ref_axis',(1.,0.,0.));
#40351=DIRECTION('',(-1.,0.,0.));
#40352=DIRECTION('center_axis',(0.,-1.,0.));
#40353=DIRECTION('ref_axis',(1.,0.,0.));
#40354=DIRECTION('center_axis',(0.,1.,0.));
#40355=DIRECTION('ref_axis',(1.,0.,0.));
#40356=DIRECTION('center_axis',(0.,1.,0.));
#40357=DIRECTION('ref_axis',(1.,0.,0.));
#40358=DIRECTION('',(1.,0.,0.));
#40359=DIRECTION('center_axis',(0.,1.,0.));
#40360=DIRECTION('ref_axis',(1.,0.,0.));
#40361=DIRECTION('center_axis',(0.,-1.,0.));
#40362=DIRECTION('ref_axis',(1.,0.,0.));
#40363=DIRECTION('center_axis',(0.,-1.,0.));
#40364=DIRECTION('ref_axis',(1.,0.,0.));
#40365=DIRECTION('',(0.,0.,-1.));
#40366=DIRECTION('',(1.,0.,0.));
#40367=DIRECTION('center_axis',(0.,1.,0.));
#40368=DIRECTION('ref_axis',(1.,0.,0.));
#40369=DIRECTION('',(-0.939925868419665,0.,0.341378619534878));
#40370=DIRECTION('',(0.,0.,-1.));
#40371=DIRECTION('',(-1.,0.,0.));
#40372=DIRECTION('',(0.,0.,-1.));
#40373=DIRECTION('center_axis',(0.,1.,0.));
#40374=DIRECTION('ref_axis',(1.,0.,0.));
#40375=DIRECTION('center_axis',(0.,1.,0.));
#40376=DIRECTION('ref_axis',(1.,0.,0.));
#40377=DIRECTION('',(0.,0.,-1.));
#40378=DIRECTION('center_axis',(0.,1.,0.));
#40379=DIRECTION('ref_axis',(1.,0.,0.));
#40380=DIRECTION('center_axis',(0.,1.,0.));
#40381=DIRECTION('ref_axis',(1.,0.,0.));
#40382=DIRECTION('center_axis',(0.,-1.,0.));
#40383=DIRECTION('ref_axis',(1.,0.,0.));
#40384=DIRECTION('',(0.,0.,-1.));
#40385=DIRECTION('',(-0.939925868419665,0.,0.341378619534878));
#40386=DIRECTION('center_axis',(0.,1.,0.));
#40387=DIRECTION('ref_axis',(1.,0.,0.));
#40388=DIRECTION('',(0.,0.,1.));
#40389=DIRECTION('center_axis',(0.,-1.,0.));
#40390=DIRECTION('ref_axis',(1.,0.,0.));
#40391=DIRECTION('',(0.,0.,-1.));
#40392=DIRECTION('center_axis',(0.,-1.,0.));
#40393=DIRECTION('ref_axis',(1.,0.,0.));
#40394=DIRECTION('center_axis',(0.,1.,0.));
#40395=DIRECTION('ref_axis',(1.,0.,0.));
#40396=DIRECTION('center_axis',(0.,-1.,0.));
#40397=DIRECTION('ref_axis',(1.,0.,0.));
#40398=DIRECTION('center_axis',(0.,-1.,0.));
#40399=DIRECTION('ref_axis',(1.,0.,0.));
#40400=DIRECTION('center_axis',(0.,-1.,0.));
#40401=DIRECTION('ref_axis',(1.,0.,0.));
#40402=DIRECTION('center_axis',(0.,-1.,0.));
#40403=DIRECTION('ref_axis',(1.,0.,0.));
#40404=DIRECTION('',(0.,0.,-1.));
#40405=DIRECTION('center_axis',(0.,1.,0.));
#40406=DIRECTION('ref_axis',(1.,0.,0.));
#40407=DIRECTION('center_axis',(0.,1.,0.));
#40408=DIRECTION('ref_axis',(1.,0.,0.));
#40409=DIRECTION('center_axis',(0.,1.,0.));
#40410=DIRECTION('ref_axis',(1.,0.,0.));
#40411=DIRECTION('',(0.,0.,1.));
#40412=DIRECTION('center_axis',(0.,1.,0.));
#40413=DIRECTION('ref_axis',(1.,0.,0.));
#40414=DIRECTION('',(0.939925868419665,0.,0.341378619534878));
#40415=DIRECTION('',(0.,0.,-1.));
#40416=DIRECTION('center_axis',(0.,1.,0.));
#40417=DIRECTION('ref_axis',(1.,0.,0.));
#40418=DIRECTION('center_axis',(0.,1.,0.));
#40419=DIRECTION('ref_axis',(0.,0.,1.));
#40420=DIRECTION('center_axis',(0.,1.,0.));
#40421=DIRECTION('ref_axis',(1.,0.,0.));
#40422=DIRECTION('',(0.,1.,0.));
#40423=DIRECTION('center_axis',(0.,1.,0.));
#40424=DIRECTION('ref_axis',(1.,0.,0.));
#40425=DIRECTION('center_axis',(0.,1.,0.));
#40426=DIRECTION('ref_axis',(-0.350308709236867,0.,0.936634298022873));
#40427=DIRECTION('',(-1.,0.,0.));
#40428=DIRECTION('center_axis',(0.,1.,0.));
#40429=DIRECTION('ref_axis',(1.,0.,0.));
#40430=DIRECTION('',(0.,0.,-1.));
#40431=DIRECTION('center_axis',(0.,1.,0.));
#40432=DIRECTION('ref_axis',(0.974839739501394,0.,0.222906891523915));
#40433=DIRECTION('center_axis',(-3.99809304065974E-15,1.,-3.3121011422878E-15));
#40434=DIRECTION('ref_axis',(0.977438775426633,4.67462326157961E-15,0.211218939237193));
#40435=DIRECTION('',(0.,0.,-1.));
#40436=DIRECTION('',(-1.,0.,0.));
#40437=DIRECTION('center_axis',(1.,0.,0.));
#40438=DIRECTION('ref_axis',(0.,1.,0.));
#40439=DIRECTION('',(0.,1.,0.));
#40440=DIRECTION('',(0.,0.,-1.));
#40441=DIRECTION('center_axis',(0.,1.,0.));
#40442=DIRECTION('ref_axis',(-5.05321549807E-16,0.,1.));
#40443=DIRECTION('',(0.,1.,0.));
#40444=DIRECTION('center_axis',(0.,-1.,0.));
#40445=DIRECTION('ref_axis',(1.,0.,0.));
#40446=DIRECTION('',(0.,1.,0.));
#40447=DIRECTION('center_axis',(0.,-1.,0.));
#40448=DIRECTION('ref_axis',(1.,0.,0.));
#40449=DIRECTION('',(0.,-1.,0.));
#40450=DIRECTION('center_axis',(0.,-1.,0.));
#40451=DIRECTION('ref_axis',(1.,0.,0.));
#40452=DIRECTION('',(0.,-1.,0.));
#40453=DIRECTION('center_axis',(0.,-1.,0.));
#40454=DIRECTION('ref_axis',(1.,0.,0.));
#40455=DIRECTION('',(0.,1.,0.));
#40456=DIRECTION('center_axis',(0.,-1.,0.));
#40457=DIRECTION('ref_axis',(1.,0.,0.));
#40458=DIRECTION('',(0.,1.,0.));
#40459=DIRECTION('center_axis',(0.,-1.,0.));
#40460=DIRECTION('ref_axis',(1.,0.,0.));
#40461=DIRECTION('',(0.,-1.,0.));
#40462=DIRECTION('center_axis',(0.,1.,0.));
#40463=DIRECTION('ref_axis',(1.,0.,0.));
#40464=DIRECTION('',(0.,-1.,0.));
#40465=DIRECTION('',(0.,-1.,0.));
#40466=DIRECTION('center_axis',(0.,1.,0.));
#40467=DIRECTION('ref_axis',(1.,0.,0.));
#40468=DIRECTION('',(0.,-1.,0.));
#40469=DIRECTION('center_axis',(0.,-1.,0.));
#40470=DIRECTION('ref_axis',(1.,0.,0.));
#40471=DIRECTION('center_axis',(0.,0.,1.));
#40472=DIRECTION('ref_axis',(1.,0.,0.));
#40473=DIRECTION('',(0.,1.,0.));
#40474=DIRECTION('',(1.,0.,0.));
#40475=DIRECTION('',(0.,1.,0.));
#40476=DIRECTION('center_axis',(0.,0.,1.));
#40477=DIRECTION('ref_axis',(1.,0.,0.));
#40478=DIRECTION('',(1.,0.,0.));
#40479=DIRECTION('',(0.,1.,0.));
#40480=DIRECTION('center_axis',(0.,1.,0.));
#40481=DIRECTION('ref_axis',(0.,0.,1.));
#40482=DIRECTION('',(0.,1.,0.));
#40483=DIRECTION('center_axis',(0.,-1.,0.));
#40484=DIRECTION('ref_axis',(1.,0.,0.));
#40485=DIRECTION('',(0.,-1.,0.));
#40486=DIRECTION('center_axis',(0.,-1.,0.));
#40487=DIRECTION('ref_axis',(1.,0.,0.));
#40488=DIRECTION('',(0.,-1.,0.));
#40489=DIRECTION('center_axis',(0.,-1.,0.));
#40490=DIRECTION('ref_axis',(1.,0.,0.));
#40491=DIRECTION('center_axis',(0.,0.,1.));
#40492=DIRECTION('ref_axis',(1.,0.,0.));
#40493=DIRECTION('',(0.,1.,0.));
#40494=DIRECTION('',(-1.,0.,0.));
#40495=DIRECTION('',(0.,1.,0.));
#40496=DIRECTION('center_axis',(0.,0.,1.));
#40497=DIRECTION('ref_axis',(1.,0.,0.));
#40498=DIRECTION('',(0.,-1.,0.));
#40499=DIRECTION('',(1.,0.,0.));
#40500=DIRECTION('center_axis',(0.,1.,0.));
#40501=DIRECTION('ref_axis',(-5.05321549807E-16,0.,1.));
#40502=DIRECTION('',(0.,1.,0.));
#40503=DIRECTION('center_axis',(0.,1.,0.));
#40504=DIRECTION('ref_axis',(1.,0.,0.));
#40505=DIRECTION('',(0.,1.,0.));
#40506=DIRECTION('center_axis',(0.,-1.,0.));
#40507=DIRECTION('ref_axis',(1.,0.,0.));
#40508=DIRECTION('',(0.,-1.,0.));
#40509=DIRECTION('center_axis',(0.,1.,0.));
#40510=DIRECTION('ref_axis',(1.,0.,0.));
#40511=DIRECTION('',(0.,-1.,0.));
#40512=DIRECTION('center_axis',(0.,-1.,0.));
#40513=DIRECTION('ref_axis',(1.,0.,0.));
#40514=DIRECTION('',(0.,1.,0.));
#40515=DIRECTION('center_axis',(0.,1.,0.));
#40516=DIRECTION('ref_axis',(1.,0.,0.));
#40517=DIRECTION('',(0.,1.,0.));
#40518=DIRECTION('center_axis',(0.,-1.,0.));
#40519=DIRECTION('ref_axis',(1.,0.,0.));
#40520=DIRECTION('',(0.,-1.,0.));
#40521=DIRECTION('center_axis',(0.,1.,0.));
#40522=DIRECTION('ref_axis',(1.,0.,0.));
#40523=DIRECTION('',(0.,-1.,0.));
#40524=DIRECTION('center_axis',(0.,1.,0.));
#40525=DIRECTION('ref_axis',(1.,0.,0.));
#40526=DIRECTION('',(0.,-1.,0.));
#40527=DIRECTION('center_axis',(0.,-1.,0.));
#40528=DIRECTION('ref_axis',(1.,0.,0.));
#40529=DIRECTION('center_axis',(4.93038065763E-32,0.,-1.));
#40530=DIRECTION('ref_axis',(0.,-1.,0.));
#40531=DIRECTION('',(0.,1.,0.));
#40532=DIRECTION('',(-1.,0.,0.));
#40533=DIRECTION('',(0.,1.,0.));
#40534=DIRECTION('center_axis',(4.93038065763E-32,0.,-1.));
#40535=DIRECTION('ref_axis',(0.,-1.,0.));
#40536=DIRECTION('',(1.,0.,0.));
#40537=DIRECTION('',(0.,1.,0.));
#40538=DIRECTION('center_axis',(0.,1.,0.));
#40539=DIRECTION('ref_axis',(1.22464679914735E-16,0.,-1.));
#40540=DIRECTION('',(0.,1.,0.));
#40541=DIRECTION('center_axis',(0.,-1.,0.));
#40542=DIRECTION('ref_axis',(1.,0.,0.));
#40543=DIRECTION('',(0.,-1.,0.));
#40544=DIRECTION('center_axis',(0.,-1.,0.));
#40545=DIRECTION('ref_axis',(1.,0.,0.));
#40546=DIRECTION('',(0.,-1.,0.));
#40547=DIRECTION('center_axis',(0.,-1.,0.));
#40548=DIRECTION('ref_axis',(1.,0.,0.));
#40549=DIRECTION('center_axis',(4.93038065763E-32,0.,-1.));
#40550=DIRECTION('ref_axis',(0.,-1.,0.));
#40551=DIRECTION('',(0.,1.,0.));
#40552=DIRECTION('',(-1.,0.,0.));
#40553=DIRECTION('',(0.,1.,0.));
#40554=DIRECTION('center_axis',(4.93038065763E-32,0.,-1.));
#40555=DIRECTION('ref_axis',(0.,-1.,0.));
#40556=DIRECTION('',(-1.,0.,0.));
#40557=DIRECTION('center_axis',(0.,1.,0.));
#40558=DIRECTION('ref_axis',(-1.22464679914735E-16,0.,-1.));
#40559=DIRECTION('',(0.,1.,0.));
#40560=DIRECTION('',(0.,1.,0.));
#40561=DIRECTION('center_axis',(0.,1.,0.));
#40562=DIRECTION('ref_axis',(1.,0.,0.));
#40563=DIRECTION('center_axis',(0.,1.,0.));
#40564=DIRECTION('ref_axis',(1.,0.,0.));
#40565=DIRECTION('center_axis',(0.,1.,0.));
#40566=DIRECTION('ref_axis',(1.,0.,0.));
#40567=DIRECTION('center_axis',(4.93038065763E-32,0.,-1.));
#40568=DIRECTION('ref_axis',(0.,-1.,0.));
#40569=DIRECTION('',(0.,1.,0.));
#40570=DIRECTION('',(-1.,0.,0.));
#40571=DIRECTION('',(-1.,0.,0.));
#40572=DIRECTION('center_axis',(0.,1.,0.));
#40573=DIRECTION('ref_axis',(0.260485490128613,0.,-0.965477762267188));
#40574=DIRECTION('',(0.,1.,0.));
#40575=DIRECTION('center_axis',(0.,1.,0.));
#40576=DIRECTION('ref_axis',(1.,0.,0.));
#40577=DIRECTION('center_axis',(0.,1.,0.));
#40578=DIRECTION('ref_axis',(1.,0.,0.));
#40579=DIRECTION('center_axis',(0.,1.,0.));
#40580=DIRECTION('ref_axis',(1.,0.,0.));
#40581=DIRECTION('center_axis',(0.,1.,0.));
#40582=DIRECTION('ref_axis',(1.,0.,0.));
#40583=DIRECTION('center_axis',(0.,1.,0.));
#40584=DIRECTION('ref_axis',(-3.50864490502111E-15,0.,1.));
#40585=DIRECTION('',(0.,1.,0.));
#40586=DIRECTION('center_axis',(0.,1.,0.));
#40587=DIRECTION('ref_axis',(1.,0.,0.));
#40588=DIRECTION('center_axis',(0.,-1.,0.));
#40589=DIRECTION('ref_axis',(-0.260485490128613,0.,-0.965477762267188));
#40590=DIRECTION('center_axis',(0.,1.,0.));
#40591=DIRECTION('ref_axis',(1.,0.,0.));
#40592=DIRECTION('center_axis',(0.,1.,0.));
#40593=DIRECTION('ref_axis',(1.,0.,0.));
#40594=DIRECTION('center_axis',(0.,1.,0.));
#40595=DIRECTION('ref_axis',(1.,0.,0.));
#40596=DIRECTION('center_axis',(0.,1.,0.));
#40597=DIRECTION('ref_axis',(1.,0.,0.));
#40598=DIRECTION('',(0.,1.,0.));
#40599=DIRECTION('center_axis',(4.93038065763E-32,0.,-1.));
#40600=DIRECTION('ref_axis',(0.,-1.,0.));
#40601=DIRECTION('',(-1.,0.,0.));
#40602=DIRECTION('',(-1.,0.,0.));
#40603=DIRECTION('center_axis',(1.,0.,0.));
#40604=DIRECTION('ref_axis',(0.,1.,0.));
#40605=DIRECTION('',(0.,1.,0.));
#40606=DIRECTION('',(0.,0.,-1.));
#40607=DIRECTION('',(0.,0.,-1.));
#40608=DIRECTION('',(0.,-1.,0.));
#40609=DIRECTION('center_axis',(-0.341378619534878,0.,-0.939925868419665));
#40610=DIRECTION('ref_axis',(-0.939925868419665,0.,0.341378619534878));
#40611=DIRECTION('',(0.,1.,0.));
#40612=DIRECTION('',(-0.939925868419665,0.,0.341378619534878));
#40613=DIRECTION('',(-0.939925868419665,0.,0.341378619534878));
#40614=DIRECTION('center_axis',(0.,1.,0.));
#40615=DIRECTION('ref_axis',(0.,0.,1.));
#40616=DIRECTION('',(0.,1.,0.));
#40617=DIRECTION('center_axis',(0.,1.,0.));
#40618=DIRECTION('ref_axis',(1.,0.,0.));
#40619=DIRECTION('center_axis',(0.,0.,1.));
#40620=DIRECTION('ref_axis',(1.,0.,0.));
#40621=DIRECTION('',(0.,1.,0.));
#40622=DIRECTION('',(-1.,0.,0.));
#40623=DIRECTION('',(-1.,0.,0.));
#40624=DIRECTION('center_axis',(1.,0.,0.));
#40625=DIRECTION('ref_axis',(0.,1.,0.));
#40626=DIRECTION('',(0.,1.,0.));
#40627=DIRECTION('',(0.,0.,-1.));
#40628=DIRECTION('center_axis',(0.,-1.,0.));
#40629=DIRECTION('ref_axis',(0.814642535600978,0.,0.579963394697984));
#40630=DIRECTION('',(0.,-1.,0.));
#40631=DIRECTION('center_axis',(0.,1.,0.));
#40632=DIRECTION('ref_axis',(1.,0.,0.));
#40633=DIRECTION('center_axis',(0.,1.,0.));
#40634=DIRECTION('ref_axis',(1.,0.,0.));
#40635=DIRECTION('center_axis',(0.,-1.,0.));
#40636=DIRECTION('ref_axis',(0.739062930406113,0.,-0.673636389233487));
#40637=DIRECTION('center_axis',(0.,-1.,0.));
#40638=DIRECTION('ref_axis',(1.,0.,0.));
#40639=DIRECTION('center_axis',(0.,1.,0.));
#40640=DIRECTION('ref_axis',(-0.739062931366045,0.,-0.673636388180322));
#40641=DIRECTION('',(0.,1.,0.));
#40642=DIRECTION('center_axis',(0.,1.,0.));
#40643=DIRECTION('ref_axis',(1.,0.,0.));
#40644=DIRECTION('center_axis',(0.,1.,0.));
#40645=DIRECTION('ref_axis',(-0.814642535600978,0.,0.579963394697984));
#40646=DIRECTION('center_axis',(0.,1.,0.));
#40647=DIRECTION('ref_axis',(1.,0.,0.));
#40648=DIRECTION('',(0.,1.,0.));
#40649=DIRECTION('center_axis',(1.,0.,0.));
#40650=DIRECTION('ref_axis',(0.,1.,0.));
#40651=DIRECTION('',(0.,1.,0.));
#40652=DIRECTION('center_axis',(0.,0.,1.));
#40653=DIRECTION('ref_axis',(1.,0.,0.));
#40654=DIRECTION('center_axis',(0.,-1.,0.));
#40655=DIRECTION('ref_axis',(-0.42050842009983,0.,0.907288635785297));
#40656=DIRECTION('',(0.,-1.,0.));
#40657=DIRECTION('center_axis',(0.,-1.,0.));
#40658=DIRECTION('ref_axis',(1.,0.,0.));
#40659=DIRECTION('',(0.,-1.,0.));
#40660=DIRECTION('center_axis',(-1.,0.,0.));
#40661=DIRECTION('ref_axis',(0.,0.,1.));
#40662=DIRECTION('',(0.,1.,0.));
#40663=DIRECTION('',(0.,0.,-1.));
#40664=DIRECTION('center_axis',(0.,1.,0.));
#40665=DIRECTION('ref_axis',(0.,0.,1.));
#40666=DIRECTION('',(0.,1.,0.));
#40667=DIRECTION('center_axis',(0.,1.,0.));
#40668=DIRECTION('ref_axis',(1.,0.,0.));
#40669=DIRECTION('center_axis',(0.,1.,0.));
#40670=DIRECTION('ref_axis',(1.,0.,0.));
#40671=DIRECTION('center_axis',(-0.341378619534878,0.,-0.939925868419665));
#40672=DIRECTION('ref_axis',(-0.939925868419665,0.,0.341378619534878));
#40673=DIRECTION('',(0.,1.,0.));
#40674=DIRECTION('',(-0.939925868419665,0.,0.341378619534878));
#40675=DIRECTION('',(-0.939925868419665,0.,0.341378619534878));
#40676=DIRECTION('center_axis',(1.,0.,0.));
#40677=DIRECTION('ref_axis',(0.,1.,0.));
#40678=DIRECTION('',(0.,1.,0.));
#40679=DIRECTION('',(0.,0.,-1.));
#40680=DIRECTION('center_axis',(0.,-1.,0.));
#40681=DIRECTION('ref_axis',(0.707106781186548,0.,-0.707106781186548));
#40682=DIRECTION('center_axis',(0.,-1.,0.));
#40683=DIRECTION('ref_axis',(1.,0.,0.));
#40684=DIRECTION('',(0.,-1.,0.));
#40685=DIRECTION('center_axis',(0.,-1.,0.));
#40686=DIRECTION('ref_axis',(1.,0.,0.));
#40687=DIRECTION('center_axis',(0.,1.,0.));
#40688=DIRECTION('ref_axis',(1.,0.,0.));
#40689=DIRECTION('',(0.,1.,0.));
#40690=DIRECTION('center_axis',(0.,-1.,0.));
#40691=DIRECTION('ref_axis',(1.,0.,0.));
#40692=DIRECTION('center_axis',(0.,-1.,0.));
#40693=DIRECTION('ref_axis',(1.,0.,0.));
#40694=DIRECTION('center_axis',(0.,-1.,0.));
#40695=DIRECTION('ref_axis',(1.,0.,0.));
#40696=DIRECTION('center_axis',(0.,-1.,0.));
#40697=DIRECTION('ref_axis',(1.,0.,0.));
#40698=DIRECTION('center_axis',(0.,1.,0.));
#40699=DIRECTION('ref_axis',(-2.83274710209661E-16,0.,1.));
#40700=DIRECTION('',(0.,1.,0.));
#40701=DIRECTION('center_axis',(0.,1.,0.));
#40702=DIRECTION('ref_axis',(1.,0.,0.));
#40703=DIRECTION('center_axis',(1.,0.,0.));
#40704=DIRECTION('ref_axis',(0.,1.,0.));
#40705=DIRECTION('',(0.,1.,0.));
#40706=DIRECTION('',(0.,0.,-1.));
#40707=DIRECTION('center_axis',(0.,1.,0.));
#40708=DIRECTION('ref_axis',(1.,0.,-1.73472347597681E-15));
#40709=DIRECTION('center_axis',(0.,-1.,0.));
#40710=DIRECTION('ref_axis',(1.,0.,0.));
#40711=DIRECTION('',(0.,1.,0.));
#40712=DIRECTION('center_axis',(0.,-1.,0.));
#40713=DIRECTION('ref_axis',(-0.785616163798045,0.,-0.618714185370954));
#40714=DIRECTION('center_axis',(0.,-1.,0.));
#40715=DIRECTION('ref_axis',(1.,0.,0.));
#40716=DIRECTION('',(0.,1.,0.));
#40717=DIRECTION('center_axis',(0.,1.,0.));
#40718=DIRECTION('ref_axis',(-0.974728984364045,0.,0.22339070491101));
#40719=DIRECTION('center_axis',(0.,-1.,0.));
#40720=DIRECTION('ref_axis',(1.,0.,0.));
#40721=DIRECTION('',(0.,1.,0.));
#40722=DIRECTION('center_axis',(0.,1.,0.));
#40723=DIRECTION('ref_axis',(-1.52656512918906E-15,0.,1.));
#40724=DIRECTION('center_axis',(0.,-1.,0.));
#40725=DIRECTION('ref_axis',(1.,0.,0.));
#40726=DIRECTION('',(0.,1.,0.));
#40727=DIRECTION('center_axis',(0.,1.,0.));
#40728=DIRECTION('ref_axis',(0.785616163798045,0.,-0.618714185370954));
#40729=DIRECTION('',(0.,1.,0.));
#40730=DIRECTION('center_axis',(0.,1.,0.));
#40731=DIRECTION('ref_axis',(1.,0.,0.));
#40732=DIRECTION('center_axis',(0.,-1.,0.));
#40733=DIRECTION('ref_axis',(-1.,0.,0.));
#40734=DIRECTION('center_axis',(0.,-1.,0.));
#40735=DIRECTION('ref_axis',(1.,0.,0.));
#40736=DIRECTION('',(0.,1.,0.));
#40737=DIRECTION('center_axis',(1.,0.,0.));
#40738=DIRECTION('ref_axis',(0.,1.,0.));
#40739=DIRECTION('',(0.,0.,-1.));
#40740=DIRECTION('center_axis',(0.,1.,0.));
#40741=DIRECTION('ref_axis',(-0.707106781186548,0.,-0.707106781186548));
#40742=DIRECTION('',(0.,1.,0.));
#40743=DIRECTION('center_axis',(0.,1.,0.));
#40744=DIRECTION('ref_axis',(1.,0.,0.));
#40745=DIRECTION('',(0.,-1.,0.));
#40746=DIRECTION('center_axis',(1.,0.,0.));
#40747=DIRECTION('ref_axis',(0.,1.,0.));
#40748=DIRECTION('',(0.,0.,-1.));
#40749=DIRECTION('',(0.,1.,0.));
#40750=DIRECTION('center_axis',(-0.341378619534878,0.,0.939925868419665));
#40751=DIRECTION('ref_axis',(0.,1.,0.));
#40752=DIRECTION('',(0.,1.,0.));
#40753=DIRECTION('',(0.939925868419665,0.,0.341378619534878));
#40754=DIRECTION('',(0.939925868419665,0.,0.341378619534878));
#40755=DIRECTION('center_axis',(0.,1.,0.));
#40756=DIRECTION('ref_axis',(0.,0.,1.));
#40757=DIRECTION('',(0.,1.,0.));
#40758=DIRECTION('center_axis',(0.,1.,0.));
#40759=DIRECTION('ref_axis',(1.,0.,0.));
#40760=DIRECTION('center_axis',(0.,1.,0.));
#40761=DIRECTION('ref_axis',(1.,0.,0.));
#40762=DIRECTION('center_axis',(-1.,0.,0.));
#40763=DIRECTION('ref_axis',(0.,0.,1.));
#40764=DIRECTION('',(0.,1.,0.));
#40765=DIRECTION('',(0.,0.,-1.));
#40766=DIRECTION('center_axis',(0.,1.,0.));
#40767=DIRECTION('ref_axis',(0.42050842009983,0.,0.907288635785297));
#40768=DIRECTION('center_axis',(0.,1.,0.));
#40769=DIRECTION('ref_axis',(1.,0.,0.));
#40770=DIRECTION('',(0.,-1.,0.));
#40771=DIRECTION('center_axis',(0.,1.,0.));
#40772=DIRECTION('ref_axis',(-1.,0.,0.));
#40773=DIRECTION('center_axis',(0.,1.,0.));
#40774=DIRECTION('ref_axis',(1.,0.,0.));
#40775=DIRECTION('center_axis',(0.,1.,0.));
#40776=DIRECTION('ref_axis',(1.,0.,0.));
#40777=DIRECTION('center_axis',(0.,1.,0.));
#40778=DIRECTION('ref_axis',(1.,0.,0.));
#40779=DIRECTION('center_axis',(0.,1.,0.));
#40780=DIRECTION('ref_axis',(1.,0.,0.));
#40781=DIRECTION('',(0.,-1.,0.));
#40782=DIRECTION('center_axis',(0.,-1.,0.));
#40783=DIRECTION('ref_axis',(1.,0.,0.));
#40784=DIRECTION('center_axis',(0.,-1.,0.));
#40785=DIRECTION('ref_axis',(1.,0.,0.));
#40786=DIRECTION('center_axis',(0.,1.,0.));
#40787=DIRECTION('ref_axis',(1.,0.,0.));
#40788=DIRECTION('center_axis',(0.,1.,0.));
#40789=DIRECTION('ref_axis',(1.,0.,0.));
#40790=DIRECTION('',(0.,0.,-1.));
#40791=DIRECTION('center_axis',(-1.,0.,0.));
#40792=DIRECTION('ref_axis',(0.,0.,1.));
#40793=DIRECTION('',(0.,0.,-1.));
#40794=DIRECTION('',(0.,-1.,0.));
#40795=DIRECTION('center_axis',(0.,0.,1.));
#40796=DIRECTION('ref_axis',(1.,0.,0.));
#40797=DIRECTION('',(0.,-1.,0.));
#40798=DIRECTION('',(-1.,0.,0.));
#40799=DIRECTION('',(0.,1.,0.));
#40800=DIRECTION('',(-1.,0.,0.));
#40801=DIRECTION('',(-1.,0.,0.));
#40802=DIRECTION('',(0.,1.,0.));
#40803=DIRECTION('',(-1.,0.,0.));
#40804=DIRECTION('center_axis',(0.,1.,0.));
#40805=DIRECTION('ref_axis',(1.,0.,0.));
#40806=DIRECTION('center_axis',(0.,1.,0.));
#40807=DIRECTION('ref_axis',(-0.989619470215645,0.,0.143712574850308));
#40808=DIRECTION('',(-1.,0.,0.));
#40809=DIRECTION('center_axis',(0.,0.,1.));
#40810=DIRECTION('ref_axis',(1.,0.,0.));
#40811=DIRECTION('',(-1.,0.,0.));
#40812=DIRECTION('',(0.,1.,0.));
#40813=DIRECTION('',(-1.,0.,0.));
#40814=DIRECTION('',(0.,1.,0.));
#40815=DIRECTION('',(-1.,0.,0.));
#40816=DIRECTION('',(0.,-1.,0.));
#40817=DIRECTION('center_axis',(-1.,0.,0.));
#40818=DIRECTION('ref_axis',(0.,0.,1.));
#40819=DIRECTION('',(0.,0.,-1.));
#40820=DIRECTION('',(0.,0.,-1.));
#40821=DIRECTION('',(0.,-1.,0.));
#40822=DIRECTION('center_axis',(0.,1.,0.));
#40823=DIRECTION('ref_axis',(1.,0.,0.));
#40824=DIRECTION('center_axis',(0.,1.,0.));
#40825=DIRECTION('ref_axis',(1.,0.,0.));
#40826=DIRECTION('',(0.,0.,-1.));
#40827=DIRECTION('center_axis',(-1.,0.,0.));
#40828=DIRECTION('ref_axis',(0.,0.,1.));
#40829=DIRECTION('',(0.,-1.,0.));
#40830=DIRECTION('',(0.,0.,-1.));
#40831=DIRECTION('center_axis',(0.,1.,0.));
#40832=DIRECTION('ref_axis',(1.,0.,0.));
#40833=DIRECTION('',(0.,0.,-1.));
#40834=DIRECTION('center_axis',(-1.,0.,0.));
#40835=DIRECTION('ref_axis',(0.,0.,1.));
#40836=DIRECTION('',(0.,-1.,0.));
#40837=DIRECTION('',(0.,0.,-1.));
#40838=DIRECTION('center_axis',(0.,0.,1.));
#40839=DIRECTION('ref_axis',(1.,0.,0.));
#40840=DIRECTION('',(-1.,0.,0.));
#40841=DIRECTION('',(0.,1.,0.));
#40842=DIRECTION('',(-1.,0.,0.));
#40843=DIRECTION('',(0.,-1.,0.));
#40844=DIRECTION('',(1.,0.,0.));
#40845=DIRECTION('',(0.,1.,0.));
#40846=DIRECTION('',(1.,0.,0.));
#40847=DIRECTION('center_axis',(0.,1.,0.));
#40848=DIRECTION('ref_axis',(1.,0.,0.));
#40849=DIRECTION('center_axis',(2.56173517218487E-14,-1.,0.));
#40850=DIRECTION('ref_axis',(0.989619470215645,2.526255984177E-14,0.143712574850308));
#40851=DIRECTION('',(1.,0.,0.));
#40852=DIRECTION('center_axis',(0.,0.,1.));
#40853=DIRECTION('ref_axis',(1.,0.,0.));
#40854=DIRECTION('',(0.,1.,0.));
#40855=DIRECTION('',(1.,0.,0.));
#40856=DIRECTION('',(0.,-1.,0.));
#40857=DIRECTION('',(-1.,0.,0.));
#40858=DIRECTION('',(0.,1.,0.));
#40859=DIRECTION('',(-1.,0.,0.));
#40860=DIRECTION('center_axis',(0.,1.,0.));
#40861=DIRECTION('ref_axis',(1.,0.,0.));
#40862=DIRECTION('',(0.,0.,-1.));
#40863=DIRECTION('',(0.,0.,-1.));
#40864=DIRECTION('center_axis',(0.,-1.,0.));
#40865=DIRECTION('ref_axis',(-7.00720136310847E-15,0.,-1.));
#40866=DIRECTION('center_axis',(0.,0.,-1.));
#40867=DIRECTION('ref_axis',(0.70710678118139,0.707106781191705,0.));
#40868=DIRECTION('center_axis',(0.,0.,-1.));
#40869=DIRECTION('ref_axis',(-0.70710678118139,0.707106781191705,0.));
#40870=DIRECTION('center_axis',(0.,1.,0.));
#40871=DIRECTION('ref_axis',(1.,0.,0.));
#40872=DIRECTION('',(0.,0.,-1.));
#40873=DIRECTION('center_axis',(0.,1.,0.));
#40874=DIRECTION('ref_axis',(1.,0.,0.));
#40875=DIRECTION('center_axis',(0.,1.,0.));
#40876=DIRECTION('ref_axis',(1.,0.,-8.24040019504512E-15));
#40877=DIRECTION('',(0.,0.,-1.));
#40878=DIRECTION('center_axis',(0.,1.,0.));
#40879=DIRECTION('ref_axis',(1.,0.,0.));
#40880=DIRECTION('center_axis',(0.,1.,0.));
#40881=DIRECTION('ref_axis',(1.,0.,0.));
#40882=DIRECTION('',(0.,0.,-1.));
#40883=DIRECTION('',(0.,0.,-1.));
#40884=DIRECTION('center_axis',(0.,1.,0.));
#40885=DIRECTION('ref_axis',(1.,0.,0.));
#40886=DIRECTION('center_axis',(0.,1.,0.));
#40887=DIRECTION('ref_axis',(1.,0.,0.));
#40888=DIRECTION('center_axis',(0.,1.,0.));
#40889=DIRECTION('ref_axis',(1.,0.,0.));
#40890=DIRECTION('center_axis',(0.,1.,0.));
#40891=DIRECTION('ref_axis',(0.974839739488413,0.,-0.222906891580687));
#40892=DIRECTION('center_axis',(0.,1.,0.));
#40893=DIRECTION('ref_axis',(1.,0.,0.));
#40894=DIRECTION('center_axis',(0.,1.,0.));
#40895=DIRECTION('ref_axis',(0.350308709237325,0.,0.936634298022702));
#40896=DIRECTION('center_axis',(0.,1.,0.));
#40897=DIRECTION('ref_axis',(1.,0.,0.));
#40898=DIRECTION('center_axis',(0.,1.,0.));
#40899=DIRECTION('ref_axis',(1.,0.,0.));
#40900=DIRECTION('',(0.,0.,-1.));
#40901=DIRECTION('center_axis',(0.,1.,0.));
#40902=DIRECTION('ref_axis',(0.949788039554192,0.,0.312894039444354));
#40903=DIRECTION('center_axis',(0.,1.,0.));
#40904=DIRECTION('ref_axis',(1.,0.,0.));
#40905=DIRECTION('center_axis',(0.,1.,0.));
#40906=DIRECTION('ref_axis',(0.662256581371297,0.,0.749277131928103));
#40907=DIRECTION('center_axis',(0.,1.,0.));
#40908=DIRECTION('ref_axis',(1.,0.,0.));
#40909=DIRECTION('center_axis',(0.,1.,0.));
#40910=DIRECTION('ref_axis',(1.,0.,7.89491928622333E-16));
#40911=DIRECTION('center_axis',(-9.86864910777917E-16,0.,1.));
#40912=DIRECTION('ref_axis',(-1.,0.,-9.86864910777917E-16));
#40913=DIRECTION('center_axis',(0.,1.,0.));
#40914=DIRECTION('ref_axis',(1.,0.,0.));
#40915=DIRECTION('center_axis',(0.,-1.,0.));
#40916=DIRECTION('ref_axis',(0.,0.,-1.));
#40917=DIRECTION('center_axis',(0.,-1.,0.));
#40918=DIRECTION('ref_axis',(1.,0.,0.));
#40919=DIRECTION('center_axis',(0.,1.,0.));
#40920=DIRECTION('ref_axis',(1.,0.,0.));
#40921=DIRECTION('center_axis',(0.,-1.,0.));
#40922=DIRECTION('ref_axis',(1.,0.,0.));
#40923=DIRECTION('center_axis',(0.,-1.,0.));
#40924=DIRECTION('ref_axis',(1.,0.,0.));
#40925=DIRECTION('center_axis',(0.,-1.,0.));
#40926=DIRECTION('ref_axis',(1.,0.,0.));
#40927=DIRECTION('',(0.,0.,-1.));
#40928=DIRECTION('center_axis',(0.,-1.,0.));
#40929=DIRECTION('ref_axis',(1.,0.,0.));
#40930=DIRECTION('center_axis',(0.,1.,0.));
#40931=DIRECTION('ref_axis',(1.,0.,0.));
#40932=DIRECTION('',(0.,0.,-1.));
#40933=DIRECTION('center_axis',(0.,1.,0.));
#40934=DIRECTION('ref_axis',(1.,0.,0.));
#40935=DIRECTION('center_axis',(0.,-1.,0.));
#40936=DIRECTION('ref_axis',(1.,0.,0.));
#40937=DIRECTION('center_axis',(0.,1.,0.));
#40938=DIRECTION('ref_axis',(1.,0.,0.));
#40939=DIRECTION('center_axis',(0.,1.,0.));
#40940=DIRECTION('ref_axis',(-0.662256581371391,0.,0.749277131928019));
#40941=DIRECTION('center_axis',(0.,1.,0.));
#40942=DIRECTION('ref_axis',(1.,0.,0.));
#40943=DIRECTION('',(0.,0.,-1.));
#40944=DIRECTION('center_axis',(0.,1.,0.));
#40945=DIRECTION('ref_axis',(0.949788039554207,0.,-0.312894039444309));
#40946=DIRECTION('center_axis',(0.,1.,0.));
#40947=DIRECTION('ref_axis',(1.,0.,0.));
#40948=DIRECTION('center_axis',(0.,1.,0.));
#40949=DIRECTION('ref_axis',(1.,0.,2.368475785867E-15));
#40950=DIRECTION('center_axis',(-1.97372982155583E-15,0.,1.));
#40951=DIRECTION('ref_axis',(-1.,0.,-1.97372982155583E-15));
#40952=DIRECTION('center_axis',(0.,-1.,0.));
#40953=DIRECTION('ref_axis',(1.,0.,0.));
#40954=DIRECTION('center_axis',(0.,0.,-1.));
#40955=DIRECTION('ref_axis',(-0.707106781186548,0.707106781186547,0.));
#40956=DIRECTION('',(0.,0.,-1.));
#40957=DIRECTION('center_axis',(0.,1.,0.));
#40958=DIRECTION('ref_axis',(0.,0.,1.));
#40959=DIRECTION('center_axis',(0.,-1.,0.));
#40960=DIRECTION('ref_axis',(1.,0.,0.));
#40961=DIRECTION('center_axis',(0.,-1.,0.));
#40962=DIRECTION('ref_axis',(1.,0.,0.));
#40963=DIRECTION('center_axis',(0.,1.,0.));
#40964=DIRECTION('ref_axis',(-1.,0.,0.));
#40965=DIRECTION('',(0.,1.,0.));
#40966=DIRECTION('center_axis',(0.,-1.,0.));
#40967=DIRECTION('ref_axis',(1.,0.,0.));
#40968=DIRECTION('center_axis',(0.,1.,0.));
#40969=DIRECTION('ref_axis',(1.,0.,0.));
#40970=DIRECTION('center_axis',(0.,-1.,0.));
#40971=DIRECTION('ref_axis',(0.720353042651791,0.,0.693607593630799));
#40972=DIRECTION('center_axis',(0.,-1.,0.));
#40973=DIRECTION('ref_axis',(1.,0.,0.));
#40974=DIRECTION('',(0.,-1.,0.));
#40975=DIRECTION('center_axis',(0.,1.,0.));
#40976=DIRECTION('ref_axis',(1.,0.,0.));
#40977=DIRECTION('',(0.,-1.,0.));
#40978=DIRECTION('center_axis',(0.,1.,0.));
#40979=DIRECTION('ref_axis',(-1.,0.,0.));
#40980=DIRECTION('',(0.,1.,0.));
#40981=DIRECTION('center_axis',(0.,1.,0.));
#40982=DIRECTION('ref_axis',(1.,0.,0.));
#40983=DIRECTION('',(0.,1.,0.));
#40984=DIRECTION('center_axis',(0.,-1.,0.));
#40985=DIRECTION('ref_axis',(1.,0.,0.));
#40986=DIRECTION('center_axis',(0.,1.,0.));
#40987=DIRECTION('ref_axis',(-1.,0.,0.));
#40988=DIRECTION('',(0.,1.,0.));
#40989=DIRECTION('center_axis',(0.,-1.,0.));
#40990=DIRECTION('ref_axis',(1.,0.,0.));
#40991=DIRECTION('',(0.,1.,0.));
#40992=DIRECTION('center_axis',(0.,1.,0.));
#40993=DIRECTION('ref_axis',(1.,0.,0.));
#40994=DIRECTION('center_axis',(0.,1.,0.));
#40995=DIRECTION('ref_axis',(-0.720353042651791,0.,0.693607593630799));
#40996=DIRECTION('center_axis',(0.,-1.,0.));
#40997=DIRECTION('ref_axis',(1.,0.,0.));
#40998=DIRECTION('',(0.,-1.,0.));
#40999=DIRECTION('center_axis',(0.,-1.,0.));
#41000=DIRECTION('ref_axis',(1.,0.,0.));
#41001=DIRECTION('',(0.,-1.,0.));
#41002=DIRECTION('center_axis',(0.,1.,0.));
#41003=DIRECTION('ref_axis',(-1.,0.,0.));
#41004=DIRECTION('',(0.,1.,0.));
#41005=DIRECTION('center_axis',(0.,1.,0.));
#41006=DIRECTION('ref_axis',(1.,0.,0.));
#41007=DIRECTION('center_axis',(0.,-1.,0.));
#41008=DIRECTION('ref_axis',(1.,0.,0.));
#41009=DIRECTION('center_axis',(1.,0.,0.));
#41010=DIRECTION('ref_axis',(0.,1.,0.));
#41011=DIRECTION('',(0.,0.,-1.));
#41012=DIRECTION('',(0.,0.,-1.));
#41013=DIRECTION('center_axis',(0.,1.,0.));
#41014=DIRECTION('ref_axis',(1.,0.,0.));
#41015=DIRECTION('center_axis',(0.,1.,0.));
#41016=DIRECTION('ref_axis',(1.,0.,0.));
#41017=DIRECTION('center_axis',(0.,1.,0.));
#41018=DIRECTION('ref_axis',(-1.,0.,-2.44929359829735E-16));
#41019=DIRECTION('center_axis',(0.,1.,0.));
#41020=DIRECTION('ref_axis',(1.,0.,0.));
#41021=DIRECTION('',(0.716064653815062,0.,0.698033961606966));
#41022=DIRECTION('center_axis',(0.,1.,0.));
#41023=DIRECTION('ref_axis',(-0.137277512281788,0.,-0.990532626732569));
#41024=DIRECTION('',(0.,0.,-1.));
#41025=DIRECTION('center_axis',(0.,-1.,0.));
#41026=DIRECTION('ref_axis',(-0.0324675324676818,0.,-0.999472790692903));
#41027=DIRECTION('center_axis',(0.,1.,0.));
#41028=DIRECTION('ref_axis',(1.,0.,0.));
#41029=DIRECTION('center_axis',(0.,-1.,0.));
#41030=DIRECTION('ref_axis',(-0.670496489123443,0.,-0.741912702461102));
#41031=DIRECTION('center_axis',(-5.55025254589126E-14,1.,2.83382379459511E-15));
#41032=DIRECTION('ref_axis',(-0.698033961645093,-4.44089209850066E-14,0.716064653777895));
#41033=DIRECTION('',(0.716064653810392,0.,0.698033961611757));
#41034=DIRECTION('',(0.71606465381051,0.,0.698033961611635));
#41035=DIRECTION('center_axis',(1.03196692270593E-15,1.,-5.46377092356529E-14));
#41036=DIRECTION('ref_axis',(-0.670496489136716,-4.44089209850059E-14,-0.741912702449107));
#41037=DIRECTION('center_axis',(0.,1.,0.));
#41038=DIRECTION('ref_axis',(1.,0.,0.));
#41039=DIRECTION('',(0.716064653808873,0.,0.698033961613315));
#41040=DIRECTION('center_axis',(0.,-1.,0.));
#41041=DIRECTION('ref_axis',(-0.818163015360923,0.,-0.574986330529276));
#41042=DIRECTION('',(-0.716064653796352,0.,0.69803396162616));
#41043=DIRECTION('center_axis',(0.,1.,0.));
#41044=DIRECTION('ref_axis',(-0.698033961628439,0.,-0.716064653794129));
#41045=DIRECTION('',(0.698033961547156,0.,0.716064653873366));
#41046=DIRECTION('center_axis',(0.,1.,0.));
#41047=DIRECTION('ref_axis',(0.716064653746231,0.,-0.698033961677575));
#41048=DIRECTION('',(-0.716064653813429,0.,0.698033961608642));
#41049=DIRECTION('center_axis',(-5.78811379739961E-14,1.,-3.92120274457636E-15));
#41050=DIRECTION('ref_axis',(-0.788233466082538,-4.44089209850063E-14,0.615376310031113));
#41051=DIRECTION('center_axis',(2.02347729834534E-15,1.,5.69830917539279E-14));
#41052=DIRECTION('ref_axis',(0.698033961510944,-4.44089209850061E-14,0.716064653908666));
#41053=DIRECTION('',(-0.716064653799089,0.,0.698033961623351));
#41054=DIRECTION('center_axis',(0.,1.,0.));
#41055=DIRECTION('ref_axis',(-0.698033961694648,0.,-0.716064653729587));
#41056=DIRECTION('',(0.698033961635916,0.,0.716064653786841));
#41057=DIRECTION('center_axis',(0.,1.,0.));
#41058=DIRECTION('ref_axis',(0.716064653777882,0.,-0.698033961645107));
#41059=DIRECTION('',(-0.716064653794199,0.,0.698033961628368));
#41060=DIRECTION('',(0.,0.,-1.));
#41061=DIRECTION('center_axis',(-3.40810699911546E-15,-1.,3.13651749681814E-15));
#41062=DIRECTION('ref_axis',(-0.999929890837095,3.15250835974135E-15,-0.0118411743723115));
#41063=DIRECTION('center_axis',(6.83821351836324E-14,1.,-8.83723547502582E-14));
#41064=DIRECTION('ref_axis',(-0.262414447485415,-8.88178419700126E-14,-0.964955262046342));
#41065=DIRECTION('center_axis',(0.,1.,0.));
#41066=DIRECTION('ref_axis',(-1.,0.,0.));
#41067=DIRECTION('',(0.,1.,0.));
#41068=DIRECTION('center_axis',(0.,1.,0.));
#41069=DIRECTION('ref_axis',(1.,0.,0.));
#41070=DIRECTION('center_axis',(0.,-1.,0.));
#41071=DIRECTION('ref_axis',(-0.720675546312773,0.,-0.693272498334375));
#41072=DIRECTION('',(0.,-1.,0.));
#41073=DIRECTION('center_axis',(0.,1.,0.));
#41074=DIRECTION('ref_axis',(1.,0.,0.));
#41075=DIRECTION('',(0.,-1.,0.));
#41076=DIRECTION('center_axis',(0.,1.,0.));
#41077=DIRECTION('ref_axis',(-1.,0.,0.));
#41078=DIRECTION('',(0.,1.,0.));
#41079=DIRECTION('',(0.,1.,0.));
#41080=DIRECTION('center_axis',(0.,1.,0.));
#41081=DIRECTION('ref_axis',(1.,0.,0.));
#41082=DIRECTION('center_axis',(0.,1.,0.));
#41083=DIRECTION('ref_axis',(-1.,0.,0.));
#41084=DIRECTION('',(0.,1.,0.));
#41085=DIRECTION('center_axis',(0.,1.,0.));
#41086=DIRECTION('ref_axis',(1.,0.,0.));
#41087=DIRECTION('',(0.,1.,0.));
#41088=DIRECTION('center_axis',(0.,-1.,0.));
#41089=DIRECTION('ref_axis',(1.,0.,0.));
#41090=DIRECTION('center_axis',(0.,1.,0.));
#41091=DIRECTION('ref_axis',(0.720675546312773,0.,-0.693272498334375));
#41092=DIRECTION('center_axis',(0.,-1.,0.));
#41093=DIRECTION('ref_axis',(1.,0.,0.));
#41094=DIRECTION('',(0.,-1.,0.));
#41095=DIRECTION('center_axis',(0.,-1.,0.));
#41096=DIRECTION('ref_axis',(1.,0.,0.));
#41097=DIRECTION('',(0.,-1.,0.));
#41098=DIRECTION('center_axis',(0.,1.,0.));
#41099=DIRECTION('ref_axis',(-1.,0.,0.));
#41100=DIRECTION('',(0.,1.,0.));
#41101=DIRECTION('center_axis',(0.,-1.,0.));
#41102=DIRECTION('ref_axis',(1.,0.,0.));
#41103=DIRECTION('center_axis',(0.,1.,0.));
#41104=DIRECTION('ref_axis',(1.,0.,0.));
#41105=DIRECTION('center_axis',(0.,1.,0.));
#41106=DIRECTION('ref_axis',(1.22464679914735E-16,0.,-1.));
#41107=DIRECTION('center_axis',(0.,-1.,0.));
#41108=DIRECTION('ref_axis',(1.,0.,0.));
#41109=DIRECTION('center_axis',(0.,1.,0.));
#41110=DIRECTION('ref_axis',(1.,0.,0.));
#41111=DIRECTION('',(0.,0.,-1.));
#41112=DIRECTION('center_axis',(0.,0.,-1.));
#41113=DIRECTION('ref_axis',(0.707106781186548,0.707106781186548,0.));
#41114=DIRECTION('center_axis',(0.,-1.,0.));
#41115=DIRECTION('ref_axis',(1.,0.,-2.44929359829735E-16));
#41116=DIRECTION('center_axis',(0.,-1.,0.));
#41117=DIRECTION('ref_axis',(1.,0.,0.));
#41118=DIRECTION('center_axis',(0.,1.,0.));
#41119=DIRECTION('ref_axis',(1.,0.,0.));
#41120=DIRECTION('',(0.,0.,-1.));
#41121=DIRECTION('center_axis',(1.,0.,0.));
#41122=DIRECTION('ref_axis',(0.,1.,0.));
#41123=DIRECTION('',(0.,0.,-1.));
#41124=DIRECTION('center_axis',(0.,1.,0.));
#41125=DIRECTION('ref_axis',(1.,0.,0.));
#41126=DIRECTION('',(0.,0.,-1.));
#41127=DIRECTION('center_axis',(0.,1.,0.));
#41128=DIRECTION('ref_axis',(0.0462962962962933,0.,-0.998927751616325));
#41129=DIRECTION('',(-0.716064653815062,0.,0.698033961606966));
#41130=DIRECTION('center_axis',(0.,1.,0.));
#41131=DIRECTION('ref_axis',(1.,0.,0.));
#41132=DIRECTION('',(-0.716064653810392,0.,0.698033961611757));
#41133=DIRECTION('center_axis',(5.55025254589126E-14,1.,2.83382379459511E-15));
#41134=DIRECTION('ref_axis',(0.767334963166091,-4.44089209850066E-14,-0.64124648482693));
#41135=DIRECTION('center_axis',(-1.03196692270593E-15,1.,-5.46377092356529E-14));
#41136=DIRECTION('ref_axis',(-0.698033961459682,-4.44089209850059E-14,-0.716064653958638));
#41137=DIRECTION('',(-0.71606465381051,0.,0.698033961611635));
#41138=DIRECTION('center_axis',(0.,1.,0.));
#41139=DIRECTION('ref_axis',(1.,0.,0.));
#41140=DIRECTION('center_axis',(5.55025254589126E-14,1.,-2.83382379459511E-15));
#41141=DIRECTION('ref_axis',(0.698033961645093,-4.44089209850066E-14,-0.716064653777895));
#41142=DIRECTION('',(0.716064653788584,0.,0.698033961634128));
#41143=DIRECTION('center_axis',(0.,1.,0.));
#41144=DIRECTION('ref_axis',(-0.698033961474199,0.,0.716064653944486));
#41145=DIRECTION('',(-0.698033961547149,0.,0.716064653873372));
#41146=DIRECTION('center_axis',(0.,1.,0.));
#41147=DIRECTION('ref_axis',(-0.716064653908654,0.,-0.698033961510957));
#41148=DIRECTION('',(0.716064653792681,0.,0.698033961629925));
#41149=DIRECTION('',(-0.716064653808873,0.,0.698033961613315));
#41150=DIRECTION('center_axis',(0.,-1.,0.));
#41151=DIRECTION('ref_axis',(0.262414447485428,0.,-0.964955262046338));
#41152=DIRECTION('center_axis',(0.,1.,0.));
#41153=DIRECTION('ref_axis',(0.999929890837095,0.,-0.0118411743723112));
#41154=DIRECTION('',(0.,0.,-1.));
#41155=DIRECTION('',(0.716064653815542,0.,0.698033961606474));
#41156=DIRECTION('center_axis',(0.,1.,0.));
#41157=DIRECTION('ref_axis',(-0.698033961677567,0.,0.716064653746239));
#41158=DIRECTION('',(-0.698033961510961,0.,0.71606465390865));
#41159=DIRECTION('center_axis',(0.,1.,0.));
#41160=DIRECTION('ref_axis',(-0.716064653794122,0.,-0.698033961628447));
#41161=DIRECTION('',(0.716064653808028,0.,0.698033961614182));
#41162=DIRECTION('center_axis',(-1.03196692270593E-15,1.,5.46377092356529E-14));
#41163=DIRECTION('ref_axis',(0.670496489136716,-4.44089209850059E-14,0.741912702449107));
#41164=DIRECTION('center_axis',(0.,1.,0.));
#41165=DIRECTION('ref_axis',(1.,0.,0.));
#41166=DIRECTION('center_axis',(0.,1.,0.));
#41167=DIRECTION('ref_axis',(-1.,0.,0.));
#41168=DIRECTION('center_axis',(0.,1.,0.));
#41169=DIRECTION('ref_axis',(1.,0.,8.67361737988404E-16));
#41170=DIRECTION('',(0.,1.,0.));
#41171=DIRECTION('center_axis',(0.,1.,0.));
#41172=DIRECTION('ref_axis',(1.,0.,0.));
#41173=DIRECTION('',(0.,1.,0.));
#41174=DIRECTION('center_axis',(0.,1.,0.));
#41175=DIRECTION('ref_axis',(-0.993447607883928,0.,0.114288452564992));
#41176=DIRECTION('center_axis',(0.,-1.,0.));
#41177=DIRECTION('ref_axis',(1.,0.,0.));
#41178=DIRECTION('',(0.,1.,0.));
#41179=DIRECTION('center_axis',(0.,-1.,0.));
#41180=DIRECTION('ref_axis',(-0.97470054788071,0.,-0.223514746629933));
#41181=DIRECTION('center_axis',(0.,1.,0.));
#41182=DIRECTION('ref_axis',(1.,0.,0.));
#41183=DIRECTION('',(0.,1.,0.));
#41184=DIRECTION('center_axis',(0.,-1.,0.));
#41185=DIRECTION('ref_axis',(0.993447607883928,0.,0.114288452564992));
#41186=DIRECTION('',(0.,1.,0.));
#41187=DIRECTION('center_axis',(0.,1.,0.));
#41188=DIRECTION('ref_axis',(1.,0.,0.));
#41189=DIRECTION('center_axis',(0.,-1.,0.));
#41190=DIRECTION('ref_axis',(-1.,0.,0.));
#41191=DIRECTION('center_axis',(0.,1.,0.));
#41192=DIRECTION('ref_axis',(1.,0.,0.));
#41193=DIRECTION('',(0.,1.,0.));
#41194=DIRECTION('center_axis',(1.,0.,0.));
#41195=DIRECTION('ref_axis',(0.,1.,0.));
#41196=DIRECTION('',(0.,0.,-1.));
#41197=DIRECTION('',(0.,1.,0.));
#41198=DIRECTION('center_axis',(0.,-1.,0.));
#41199=DIRECTION('ref_axis',(2.83273781220225E-16,0.,1.));
#41200=DIRECTION('center_axis',(0.,-1.,0.));
#41201=DIRECTION('ref_axis',(1.,0.,0.));
#41202=DIRECTION('',(0.,1.,0.));
#41203=DIRECTION('center_axis',(0.,1.,0.));
#41204=DIRECTION('ref_axis',(-2.83273781220225E-16,0.,1.));
#41205=DIRECTION('center_axis',(0.,1.,0.));
#41206=DIRECTION('ref_axis',(1.,0.,0.));
#41207=DIRECTION('',(0.,1.,0.));
#41208=DIRECTION('center_axis',(1.,0.,0.));
#41209=DIRECTION('ref_axis',(0.,1.,0.));
#41210=DIRECTION('',(0.,0.,-1.));
#41211=DIRECTION('center_axis',(0.,1.,0.));
#41212=DIRECTION('ref_axis',(-1.,0.,0.));
#41213=DIRECTION('',(0.,-1.,0.));
#41214=DIRECTION('center_axis',(0.,1.,0.));
#41215=DIRECTION('ref_axis',(1.,0.,0.));
#41216=DIRECTION('center_axis',(0.,-1.,0.));
#41217=DIRECTION('ref_axis',(1.,0.,0.));
#41218=DIRECTION('center_axis',(0.,-1.,0.));
#41219=DIRECTION('ref_axis',(1.,0.,0.));
#41220=DIRECTION('',(0.,1.,0.));
#41221=DIRECTION('center_axis',(0.,1.,0.));
#41222=DIRECTION('ref_axis',(1.,0.,0.));
#41223=DIRECTION('center_axis',(0.,-1.,0.));
#41224=DIRECTION('ref_axis',(-1.,0.,0.));
#41225=DIRECTION('center_axis',(0.,-1.,0.));
#41226=DIRECTION('ref_axis',(-5.9077376355796E-5,0.,0.999999998254932));
#41227=DIRECTION('center_axis',(0.,-1.,0.));
#41228=DIRECTION('ref_axis',(1.,0.,0.));
#41229=DIRECTION('',(0.,1.,0.));
#41230=DIRECTION('',(0.,1.,0.));
#41231=DIRECTION('center_axis',(0.,1.,0.));
#41232=DIRECTION('ref_axis',(0.999929890837101,0.,0.011841174371802));
#41233=DIRECTION('center_axis',(0.,-1.,0.));
#41234=DIRECTION('ref_axis',(1.,0.,0.));
#41235=DIRECTION('',(0.,1.,0.));
#41236=DIRECTION('',(0.,1.,0.));
#41237=DIRECTION('',(0.,1.,0.));
#41238=DIRECTION('',(0.,1.,0.));
#41239=DIRECTION('',(0.,1.,0.));
#41240=DIRECTION('',(0.,1.,0.));
#41241=DIRECTION('',(0.,1.,0.));
#41242=DIRECTION('',(0.,1.,0.));
#41243=DIRECTION('center_axis',(0.,1.,0.));
#41244=DIRECTION('ref_axis',(0.137277512281937,0.,-0.990532626732549));
#41245=DIRECTION('center_axis',(0.,-1.,0.));
#41246=DIRECTION('ref_axis',(1.,0.,0.));
#41247=DIRECTION('',(0.,1.,0.));
#41248=DIRECTION('center_axis',(0.,1.,0.));
#41249=DIRECTION('ref_axis',(0.137277512281937,0.,-0.990532626732549));
#41250=DIRECTION('center_axis',(0.,-1.,0.));
#41251=DIRECTION('ref_axis',(1.,0.,0.));
#41252=DIRECTION('',(0.,1.,0.));
#41253=DIRECTION('',(0.,1.,0.));
#41254=DIRECTION('',(0.,1.,0.));
#41255=DIRECTION('',(0.,1.,0.));
#41256=DIRECTION('',(0.,1.,0.));
#41257=DIRECTION('',(0.,1.,0.));
#41258=DIRECTION('',(0.,1.,0.));
#41259=DIRECTION('',(0.,1.,0.));
#41260=DIRECTION('',(0.,-1.,0.));
#41261=DIRECTION('center_axis',(0.,-1.,0.));
#41262=DIRECTION('ref_axis',(-0.999929890837101,0.,0.011841174371802));
#41263=DIRECTION('center_axis',(0.,-1.,0.));
#41264=DIRECTION('ref_axis',(1.,0.,0.));
#41265=DIRECTION('',(0.,-1.,0.));
#41266=DIRECTION('center_axis',(0.,1.,0.));
#41267=DIRECTION('ref_axis',(5.9077376355796E-5,0.,0.999999998254932));
#41268=DIRECTION('center_axis',(0.,1.,0.));
#41269=DIRECTION('ref_axis',(1.,0.,0.));
#41270=DIRECTION('',(0.,1.,0.));
#41271=DIRECTION('center_axis',(0.,-1.,0.));
#41272=DIRECTION('ref_axis',(1.,0.,0.));
#41273=DIRECTION('center_axis',(0.,-1.,0.));
#41274=DIRECTION('ref_axis',(1.,0.,0.));
#41275=DIRECTION('',(0.,-1.,0.));
#41276=DIRECTION('center_axis',(0.,1.,0.));
#41277=DIRECTION('ref_axis',(1.,0.,0.));
#41278=DIRECTION('center_axis',(0.,1.,0.));
#41279=DIRECTION('ref_axis',(1.,0.,0.));
#41280=DIRECTION('',(0.,0.,1.));
#41281=DIRECTION('center_axis',(0.,1.,0.));
#41282=DIRECTION('ref_axis',(1.,0.,0.));
#41283=DIRECTION('center_axis',(0.,-1.,0.));
#41284=DIRECTION('ref_axis',(1.,0.,0.));
#41285=DIRECTION('',(0.,0.,1.));
#41286=DIRECTION('center_axis',(0.,1.,0.));
#41287=DIRECTION('ref_axis',(1.,0.,0.));
#41288=DIRECTION('center_axis',(0.,1.,0.));
#41289=DIRECTION('ref_axis',(1.,0.,0.));
#41290=DIRECTION('center_axis',(0.,1.,0.));
#41291=DIRECTION('ref_axis',(1.,0.,0.));
#41292=DIRECTION('center_axis',(0.,-1.,0.));
#41293=DIRECTION('ref_axis',(1.,0.,0.));
#41294=DIRECTION('center_axis',(0.,1.,0.));
#41295=DIRECTION('ref_axis',(-1.,0.,0.));
#41296=DIRECTION('',(0.,1.,0.));
#41297=DIRECTION('center_axis',(0.,1.,0.));
#41298=DIRECTION('ref_axis',(1.,0.,0.));
#41299=DIRECTION('center_axis',(0.,-1.,0.));
#41300=DIRECTION('ref_axis',(0.,0.,-1.));
#41301=DIRECTION('center_axis',(0.,-1.,0.));
#41302=DIRECTION('ref_axis',(6.12267139103014E-17,0.,1.));
#41303=DIRECTION('',(0.,1.,0.));
#41304=DIRECTION('center_axis',(0.,1.,0.));
#41305=DIRECTION('ref_axis',(1.,0.,0.));
#41306=DIRECTION('center_axis',(0.,1.,0.));
#41307=DIRECTION('ref_axis',(1.,0.,0.));
#41308=DIRECTION('center_axis',(1.,0.,0.));
#41309=DIRECTION('ref_axis',(0.,1.,0.));
#41310=DIRECTION('',(0.,0.,1.));
#41311=DIRECTION('',(0.,0.,1.));
#41312=DIRECTION('',(0.,1.,0.));
#41313=DIRECTION('center_axis',(0.,1.,0.));
#41314=DIRECTION('ref_axis',(-0.934587360002009,0.,0.355733701699003));
#41315=DIRECTION('center_axis',(0.,1.,0.));
#41316=DIRECTION('ref_axis',(1.,0.,0.));
#41317=DIRECTION('center_axis',(0.,1.,0.));
#41318=DIRECTION('ref_axis',(1.,0.,0.));
#41319=DIRECTION('',(0.,1.,0.));
#41320=DIRECTION('center_axis',(0.,-1.,0.));
#41321=DIRECTION('ref_axis',(0.934587360002009,0.,0.355733701699003));
#41322=DIRECTION('center_axis',(0.,-1.,0.));
#41323=DIRECTION('ref_axis',(1.,0.,0.));
#41324=DIRECTION('center_axis',(0.,-1.,0.));
#41325=DIRECTION('ref_axis',(1.,0.,0.));
#41326=DIRECTION('',(0.,1.,0.));
#41327=DIRECTION('center_axis',(1.,0.,0.));
#41328=DIRECTION('ref_axis',(0.,1.,0.));
#41329=DIRECTION('',(0.,0.,1.));
#41330=DIRECTION('',(1.90171128996581E-6,0.,0.999999999998192));
#41331=DIRECTION('',(0.,0.,1.));
#41332=DIRECTION('center_axis',(0.,1.,0.));
#41333=DIRECTION('ref_axis',(-1.,0.,0.));
#41334=DIRECTION('',(0.,1.,0.));
#41335=DIRECTION('center_axis',(0.,-1.,0.));
#41336=DIRECTION('ref_axis',(1.,0.,0.));
#41337=DIRECTION('center_axis',(0.,-1.,0.));
#41338=DIRECTION('ref_axis',(1.,0.,0.));
#41339=DIRECTION('center_axis',(0.,-1.,0.));
#41340=DIRECTION('ref_axis',(1.,0.,0.));
#41341=DIRECTION('center_axis',(0.,-1.,0.));
#41342=DIRECTION('ref_axis',(1.,0.,0.));
#41343=DIRECTION('center_axis',(0.,-1.,0.));
#41344=DIRECTION('ref_axis',(1.,0.,0.));
#41345=DIRECTION('center_axis',(0.,-1.,0.));
#41346=DIRECTION('ref_axis',(1.,0.,0.));
#41347=DIRECTION('center_axis',(0.,-1.,0.));
#41348=DIRECTION('ref_axis',(1.,0.,0.));
#41349=DIRECTION('center_axis',(0.,-1.,0.));
#41350=DIRECTION('ref_axis',(1.,0.,0.));
#41351=DIRECTION('center_axis',(0.,1.,0.));
#41352=DIRECTION('ref_axis',(1.,0.,0.));
#41353=DIRECTION('',(0.,-1.,0.));
#41354=DIRECTION('center_axis',(0.,1.,0.));
#41355=DIRECTION('ref_axis',(1.,0.,0.));
#41356=DIRECTION('center_axis',(0.,1.,0.));
#41357=DIRECTION('ref_axis',(1.,0.,0.));
#41358=DIRECTION('center_axis',(0.,1.,0.));
#41359=DIRECTION('ref_axis',(1.,0.,0.));
#41360=DIRECTION('center_axis',(0.,1.,0.));
#41361=DIRECTION('ref_axis',(1.,0.,0.));
#41362=DIRECTION('center_axis',(0.,1.,0.));
#41363=DIRECTION('ref_axis',(1.,0.,0.));
#41364=DIRECTION('center_axis',(0.,1.,0.));
#41365=DIRECTION('ref_axis',(1.,0.,0.));
#41366=DIRECTION('center_axis',(0.,-1.,0.));
#41367=DIRECTION('ref_axis',(0.,0.,-1.));
#41368=DIRECTION('center_axis',(0.,-1.,0.));
#41369=DIRECTION('ref_axis',(-6.66472423784048E-5,0.,0.999999997779073));
#41370=DIRECTION('center_axis',(0.,-1.,0.));
#41371=DIRECTION('ref_axis',(1.,0.,0.));
#41372=DIRECTION('',(0.,1.,0.));
#41373=DIRECTION('center_axis',(0.,-1.,0.));
#41374=DIRECTION('ref_axis',(1.,0.,0.));
#41375=DIRECTION('',(0.,-1.,0.));
#41376=DIRECTION('center_axis',(0.,-1.,0.));
#41377=DIRECTION('ref_axis',(-0.55530622998795,0.,-0.831645952876926));
#41378=DIRECTION('',(0.,-1.,0.));
#41379=DIRECTION('center_axis',(0.,-1.,0.));
#41380=DIRECTION('ref_axis',(1.,0.,0.));
#41381=DIRECTION('center_axis',(0.,-1.,0.));
#41382=DIRECTION('ref_axis',(1.,0.,0.));
#41383=DIRECTION('',(0.,1.,0.));
#41384=DIRECTION('',(0.,1.,0.));
#41385=DIRECTION('',(0.,-1.,0.));
#41386=DIRECTION('center_axis',(0.,-1.,0.));
#41387=DIRECTION('ref_axis',(-0.138699292007931,0.,-0.990334542665507));
#41388=DIRECTION('center_axis',(0.,-1.,0.));
#41389=DIRECTION('ref_axis',(1.,0.,0.));
#41390=DIRECTION('center_axis',(0.,-1.,0.));
#41391=DIRECTION('ref_axis',(1.,0.,0.));
#41392=DIRECTION('',(0.,-1.,0.));
#41393=DIRECTION('',(0.,1.,0.));
#41394=DIRECTION('',(0.,1.,0.));
#41395=DIRECTION('',(0.,1.,0.));
#41396=DIRECTION('center_axis',(0.,1.,0.));
#41397=DIRECTION('ref_axis',(0.55530622998795,0.,-0.831645952876926));
#41398=DIRECTION('',(0.,1.,0.));
#41399=DIRECTION('center_axis',(0.,-1.,0.));
#41400=DIRECTION('ref_axis',(1.,0.,0.));
#41401=DIRECTION('center_axis',(0.,1.,0.));
#41402=DIRECTION('ref_axis',(1.,0.,0.));
#41403=DIRECTION('center_axis',(0.,1.,0.));
#41404=DIRECTION('ref_axis',(6.66472423784048E-5,0.,0.999999997779073));
#41405=DIRECTION('center_axis',(0.,1.,0.));
#41406=DIRECTION('ref_axis',(1.,0.,0.));
#41407=DIRECTION('center_axis',(0.,1.,0.));
#41408=DIRECTION('ref_axis',(1.,0.,0.));
#41409=DIRECTION('center_axis',(0.,1.,0.));
#41410=DIRECTION('ref_axis',(1.,0.,0.));
#41411=DIRECTION('center_axis',(0.,-1.,0.));
#41412=DIRECTION('ref_axis',(0.358624086674959,0.,-0.933482064346472));
#41413=DIRECTION('center_axis',(0.,1.,0.));
#41414=DIRECTION('ref_axis',(0.365247039092674,0.,0.930910629670773));
#41415=DIRECTION('center_axis',(0.,1.,0.));
#41416=DIRECTION('ref_axis',(1.,0.,0.));
#41417=DIRECTION('center_axis',(0.,-1.,0.));
#41418=DIRECTION('ref_axis',(-0.999436570354898,0.,0.033563996145276));
#41419=DIRECTION('center_axis',(-4.94340750637177E-15,1.,-5.11172940430608E-15));
#41420=DIRECTION('ref_axis',(0.999436570354898,4.99714829851786E-15,0.0335639961452762));
#41421=DIRECTION('center_axis',(0.,1.,0.));
#41422=DIRECTION('ref_axis',(1.,0.,0.));
#41423=DIRECTION('',(0.,-1.,0.));
#41424=DIRECTION('',(0.,-1.,0.));
#41425=DIRECTION('center_axis',(0.,1.,0.));
#41426=DIRECTION('ref_axis',(1.,0.,0.));
#41427=DIRECTION('center_axis',(0.,-1.,0.));
#41428=DIRECTION('ref_axis',(1.,0.,0.));
#41429=DIRECTION('center_axis',(0.,1.,0.));
#41430=DIRECTION('ref_axis',(1.,0.,0.));
#41431=DIRECTION('',(0.,-1.,0.));
#41432=DIRECTION('',(0.,-1.,0.));
#41433=DIRECTION('center_axis',(0.,1.,0.));
#41434=DIRECTION('ref_axis',(1.,0.,0.));
#41435=DIRECTION('center_axis',(1.50992280148742E-14,1.,-9.75211599539184E-15));
#41436=DIRECTION('ref_axis',(0.722348824225048,-1.76507793442358E-14,-0.691528868624217));
#41437=DIRECTION('center_axis',(0.,1.,0.));
#41438=DIRECTION('ref_axis',(-0.373228907029859,0.,0.927739286091355));
#41439=DIRECTION('center_axis',(0.,1.,0.));
#41440=DIRECTION('ref_axis',(0.731786637712586,0.,0.681533797302311));
#41441=DIRECTION('center_axis',(0.,1.,0.));
#41442=DIRECTION('ref_axis',(1.,0.,0.));
#41443=DIRECTION('center_axis',(0.,1.,0.));
#41444=DIRECTION('ref_axis',(1.,0.,0.));
#41445=DIRECTION('center_axis',(0.,-1.,0.));
#41446=DIRECTION('ref_axis',(0.188519518005548,0.,-0.982069443232481));
#41447=DIRECTION('center_axis',(0.,1.,0.));
#41448=DIRECTION('ref_axis',(1.,0.,0.));
#41449=DIRECTION('center_axis',(0.,1.,0.));
#41450=DIRECTION('ref_axis',(1.,0.,0.));
#41451=DIRECTION('center_axis',(0.,1.,0.));
#41452=DIRECTION('ref_axis',(1.,0.,0.));
#41453=DIRECTION('',(0.,0.,-1.));
#41454=DIRECTION('center_axis',(0.,1.,0.));
#41455=DIRECTION('ref_axis',(1.,0.,0.));
#41456=DIRECTION('center_axis',(7.97796769687341E-14,1.,-1.47631083777498E-13));
#41457=DIRECTION('ref_axis',(0.82647940397254,-1.49047681880818E-13,-0.562966957120215));
#41458=DIRECTION('center_axis',(0.,1.,0.));
#41459=DIRECTION('ref_axis',(1.,0.,0.));
#41460=DIRECTION('center_axis',(0.,1.,0.));
#41461=DIRECTION('ref_axis',(1.,0.,0.));
#41462=DIRECTION('center_axis',(7.97796769693144E-14,-1.,1.47631083778477E-13));
#41463=DIRECTION('ref_axis',(0.826479404012423,1.49047681876387E-13,0.562966957061665));
#41464=DIRECTION('center_axis',(0.,-1.,0.));
#41465=DIRECTION('ref_axis',(1.,0.,0.));
#41466=DIRECTION('',(0.,0.,-1.));
#41467=DIRECTION('center_axis',(0.,-1.,0.));
#41468=DIRECTION('ref_axis',(1.,0.,0.));
#41469=DIRECTION('center_axis',(0.,1.,0.));
#41470=DIRECTION('ref_axis',(1.,0.,0.));
#41471=DIRECTION('center_axis',(0.,-1.,0.));
#41472=DIRECTION('ref_axis',(0.373228907029852,0.,0.927739286091358));
#41473=DIRECTION('center_axis',(1.50992280148742E-14,-1.,9.75211599539184E-15));
#41474=DIRECTION('ref_axis',(0.722348824225048,1.76507793442358E-14,0.691528868624217));
#41475=DIRECTION('center_axis',(0.,-1.,0.));
#41476=DIRECTION('ref_axis',(0.731786637488438,0.,-0.681533797542987));
#41477=DIRECTION('center_axis',(0.,1.,0.));
#41478=DIRECTION('ref_axis',(1.,0.,0.));
#41479=DIRECTION('center_axis',(0.,1.,0.));
#41480=DIRECTION('ref_axis',(1.,0.,0.));
#41481=DIRECTION('center_axis',(0.,1.,0.));
#41482=DIRECTION('ref_axis',(0.188519616822252,0.,0.982069424263474));
#41483=DIRECTION('center_axis',(0.,1.,0.));
#41484=DIRECTION('ref_axis',(1.,0.,0.));
#41485=DIRECTION('center_axis',(0.,1.,0.));
#41486=DIRECTION('ref_axis',(0.196635535421533,0.,-0.980476652557055));
#41487=DIRECTION('center_axis',(0.,-1.,0.));
#41488=DIRECTION('ref_axis',(-1.,0.,1.11022302462516E-15));
#41489=DIRECTION('',(0.,0.,-1.));
#41490=DIRECTION('center_axis',(0.,1.,0.));
#41491=DIRECTION('ref_axis',(-0.999983860839812,0.,-0.00568137834545477));
#41492=DIRECTION('center_axis',(0.,-1.,0.));
#41493=DIRECTION('ref_axis',(0.182889314799161,0.,-0.983133510024093));
#41494=DIRECTION('center_axis',(0.,1.,0.));
#41495=DIRECTION('ref_axis',(-0.201763361402965,0.,-0.979434298968224));
#41496=DIRECTION('center_axis',(0.,1.,0.));
#41497=DIRECTION('ref_axis',(0.999436570354936,0.,0.0335639961441162));
#41498=DIRECTION('center_axis',(0.,-1.,0.));
#41499=DIRECTION('ref_axis',(-0.999436570354936,0.,0.0335639961441164));
#41500=DIRECTION('center_axis',(0.,1.,0.));
#41501=DIRECTION('ref_axis',(0.18615784526743,0.,0.98251985050959));
#41502=DIRECTION('center_axis',(0.,-1.,0.));
#41503=DIRECTION('ref_axis',(0.999983860839812,0.,-0.00568137834545072));
#41504=DIRECTION('',(0.,0.,-1.));
#41505=DIRECTION('center_axis',(0.,1.,0.));
#41506=DIRECTION('ref_axis',(1.,0.,0.));
#41507=DIRECTION('center_axis',(0.,-1.,0.));
#41508=DIRECTION('ref_axis',(-0.196635535421533,0.,-0.980476652557055));
#41509=DIRECTION('center_axis',(0.,1.,0.));
#41510=DIRECTION('ref_axis',(9.36455599968238E-5,0.,0.999999995615255));
#41511=DIRECTION('center_axis',(0.,1.,0.));
#41512=DIRECTION('ref_axis',(1.,0.,0.));
#41513=DIRECTION('',(0.,-1.,0.));
#41514=DIRECTION('center_axis',(0.,-1.,0.));
#41515=DIRECTION('ref_axis',(-9.36455599961238E-5,0.,0.999999995615255));
#41516=DIRECTION('center_axis',(0.,-1.,0.));
#41517=DIRECTION('ref_axis',(1.,0.,0.));
#41518=DIRECTION('',(0.,-1.,0.));
#41519=DIRECTION('center_axis',(0.,1.,0.));
#41520=DIRECTION('ref_axis',(1.,0.,0.));
#41521=DIRECTION('center_axis',(0.,-1.,0.));
#41522=DIRECTION('ref_axis',(1.,0.,0.));
#41523=DIRECTION('center_axis',(0.,1.,0.));
#41524=DIRECTION('ref_axis',(1.,0.,0.));
#41525=DIRECTION('center_axis',(0.,-1.,0.));
#41526=DIRECTION('ref_axis',(1.,0.,0.));
#41527=DIRECTION('center_axis',(0.,-1.,0.));
#41528=DIRECTION('ref_axis',(1.,0.,0.));
#41529=DIRECTION('center_axis',(0.,-1.,0.));
#41530=DIRECTION('ref_axis',(-0.257358836141954,0.,-0.966315905622824));
#41531=DIRECTION('',(0.,-1.,0.));
#41532=DIRECTION('',(0.,-1.,0.));
#41533=DIRECTION('',(0.,-1.,0.));
#41534=DIRECTION('center_axis',(0.,1.,0.));
#41535=DIRECTION('ref_axis',(-0.898888448298522,0.,0.438177541089767));
#41536=DIRECTION('center_axis',(0.,1.,0.));
#41537=DIRECTION('ref_axis',(1.,0.,0.));
#41538=DIRECTION('',(0.,-1.,0.));
#41539=DIRECTION('',(0.,-1.,0.));
#41540=DIRECTION('',(0.,-1.,0.));
#41541=DIRECTION('',(0.,-1.,0.));
#41542=DIRECTION('',(0.,-1.,0.));
#41543=DIRECTION('',(0.,-1.,0.));
#41544=DIRECTION('center_axis',(0.,1.,0.));
#41545=DIRECTION('ref_axis',(0.17719394991793,0.,-0.984175951805612));
#41546=DIRECTION('center_axis',(0.,1.,0.));
#41547=DIRECTION('ref_axis',(1.,0.,0.));
#41548=DIRECTION('',(0.,-1.,0.));
#41549=DIRECTION('center_axis',(1.,0.,3.3635018779E-16));
#41550=DIRECTION('ref_axis',(-3.3635018779E-16,0.,1.));
#41551=DIRECTION('',(3.3635018779E-16,0.,-1.));
#41552=DIRECTION('',(0.,-1.,0.));
#41553=DIRECTION('center_axis',(0.,1.,0.));
#41554=DIRECTION('ref_axis',(-1.,0.,0.));
#41555=DIRECTION('center_axis',(0.,1.,0.));
#41556=DIRECTION('ref_axis',(1.,0.,0.));
#41557=DIRECTION('',(0.,-1.,0.));
#41558=DIRECTION('',(0.,-1.,0.));
#41559=DIRECTION('',(0.,-1.,0.));
#41560=DIRECTION('',(0.,-1.,0.));
#41561=DIRECTION('center_axis',(0.,-1.,0.));
#41562=DIRECTION('ref_axis',(1.,0.,0.));
#41563=DIRECTION('center_axis',(0.,-1.,0.));
#41564=DIRECTION('ref_axis',(1.,0.,0.));
#41565=DIRECTION('',(0.,-1.,0.));
#41566=DIRECTION('center_axis',(1.,0.,-3.3635018779E-16));
#41567=DIRECTION('ref_axis',(-3.3635018779E-16,0.,-1.));
#41568=DIRECTION('',(-3.3635018779E-16,0.,-1.));
#41569=DIRECTION('',(0.,-1.,0.));
#41570=DIRECTION('center_axis',(0.,-1.,0.));
#41571=DIRECTION('ref_axis',(-0.17719394991793,0.,-0.984175951805612));
#41572=DIRECTION('center_axis',(0.,-1.,0.));
#41573=DIRECTION('ref_axis',(1.,0.,0.));
#41574=DIRECTION('center_axis',(0.,-1.,0.));
#41575=DIRECTION('ref_axis',(0.898888448298522,0.,0.438177541089767));
#41576=DIRECTION('center_axis',(0.,-1.,0.));
#41577=DIRECTION('ref_axis',(1.,0.,0.));
#41578=DIRECTION('',(0.,-1.,0.));
#41579=DIRECTION('',(0.,-1.,0.));
#41580=DIRECTION('',(0.,-1.,0.));
#41581=DIRECTION('',(0.,-1.,0.));
#41582=DIRECTION('',(0.,1.,0.));
#41583=DIRECTION('',(0.,1.,0.));
#41584=DIRECTION('',(0.,1.,0.));
#41585=DIRECTION('center_axis',(0.,1.,0.));
#41586=DIRECTION('ref_axis',(0.426033148631104,0.,-0.904707552896221));
#41587=DIRECTION('center_axis',(0.,1.,0.));
#41588=DIRECTION('ref_axis',(1.,0.,0.));
#41589=DIRECTION('',(0.,-1.,0.));
#41590=DIRECTION('center_axis',(0.,-1.,0.));
#41591=DIRECTION('ref_axis',(-0.196635535421993,0.,0.980476652556962));
#41592=DIRECTION('',(0.,-1.,0.));
#41593=DIRECTION('center_axis',(0.,-1.,0.));
#41594=DIRECTION('ref_axis',(1.,0.,0.));
#41595=DIRECTION('center_axis',(1.,0.,0.));
#41596=DIRECTION('ref_axis',(0.,1.,0.));
#41597=DIRECTION('',(0.,0.,-1.));
#41598=DIRECTION('',(0.,1.,0.));
#41599=DIRECTION('center_axis',(0.,1.,0.));
#41600=DIRECTION('ref_axis',(0.204297691364974,0.,-0.978908807449878));
#41601=DIRECTION('',(0.,-1.,0.));
#41602=DIRECTION('center_axis',(0.,1.,0.));
#41603=DIRECTION('ref_axis',(1.,0.,0.));
#41604=DIRECTION('center_axis',(0.,-1.,0.));
#41605=DIRECTION('ref_axis',(-0.17925890877697,0.,0.983801933126831));
#41606=DIRECTION('center_axis',(0.,-1.,0.));
#41607=DIRECTION('ref_axis',(1.,0.,0.));
#41608=DIRECTION('',(0.,-1.,0.));
#41609=DIRECTION('',(0.,1.,0.));
#41610=DIRECTION('',(0.,1.,0.));
#41611=DIRECTION('',(0.,1.,0.));
#41612=DIRECTION('',(0.,1.,0.));
#41613=DIRECTION('center_axis',(0.,1.,0.));
#41614=DIRECTION('ref_axis',(0.201763361403043,0.,-0.979434298968208));
#41615=DIRECTION('',(0.,1.,0.));
#41616=DIRECTION('',(0.,1.,0.));
#41617=DIRECTION('',(0.,1.,0.));
#41618=DIRECTION('center_axis',(0.,1.,0.));
#41619=DIRECTION('ref_axis',(7.9357870457813E-5,0.,0.999999996851164));
#41620=DIRECTION('',(0.,1.,0.));
#41621=DIRECTION('center_axis',(0.,-1.,0.));
#41622=DIRECTION('ref_axis',(-7.9357870457813E-5,0.,0.999999996851164));
#41623=DIRECTION('center_axis',(0.,1.,0.));
#41624=DIRECTION('ref_axis',(0.17925890877697,0.,0.983801933126831));
#41625=DIRECTION('center_axis',(0.,-1.,0.));
#41626=DIRECTION('ref_axis',(1.,0.,0.));
#41627=DIRECTION('',(0.,1.,0.));
#41628=DIRECTION('',(0.,1.,0.));
#41629=DIRECTION('center_axis',(0.,-1.,0.));
#41630=DIRECTION('ref_axis',(-0.204297691364974,0.,-0.978908807449878));
#41631=DIRECTION('center_axis',(0.,-1.,0.));
#41632=DIRECTION('ref_axis',(1.,0.,0.));
#41633=DIRECTION('',(0.,1.,0.));
#41634=DIRECTION('center_axis',(1.,0.,0.));
#41635=DIRECTION('ref_axis',(0.,1.,0.));
#41636=DIRECTION('',(0.,0.,-1.));
#41637=DIRECTION('',(0.,1.,0.));
#41638=DIRECTION('center_axis',(0.,1.,0.));
#41639=DIRECTION('ref_axis',(0.196635535421993,0.,0.980476652556962));
#41640=DIRECTION('center_axis',(0.,-1.,0.));
#41641=DIRECTION('ref_axis',(1.,0.,0.));
#41642=DIRECTION('',(0.,1.,0.));
#41643=DIRECTION('center_axis',(0.,-1.,0.));
#41644=DIRECTION('ref_axis',(-0.426033148631104,0.,-0.904707552896221));
#41645=DIRECTION('center_axis',(0.,-1.,0.));
#41646=DIRECTION('ref_axis',(1.,0.,0.));
#41647=DIRECTION('',(0.,1.,0.));
#41648=DIRECTION('',(0.,1.,0.));
#41649=DIRECTION('',(0.,1.,0.));
#41650=DIRECTION('',(0.,1.,0.));
#41651=DIRECTION('center_axis',(0.,1.,0.));
#41652=DIRECTION('ref_axis',(1.,0.,0.));
#41653=DIRECTION('center_axis',(0.,1.,0.));
#41654=DIRECTION('ref_axis',(1.,0.,0.));
#41655=DIRECTION('center_axis',(-1.,0.,0.));
#41656=DIRECTION('ref_axis',(0.,0.,1.));
#41657=DIRECTION('',(0.,0.,1.));
#41658=DIRECTION('center_axis',(-1.,0.,0.));
#41659=DIRECTION('ref_axis',(0.,0.,1.));
#41660=DIRECTION('',(0.,0.,1.));
#41661=DIRECTION('center_axis',(-1.,0.,0.));
#41662=DIRECTION('ref_axis',(0.,0.,1.));
#41663=DIRECTION('',(0.,0.,1.));
#41664=DIRECTION('center_axis',(-1.,0.,0.));
#41665=DIRECTION('ref_axis',(0.,0.,1.));
#41666=DIRECTION('',(0.,0.,1.));
#41667=DIRECTION('center_axis',(-0.698033961608027,0.,0.716064653814028));
#41668=DIRECTION('ref_axis',(0.,1.,0.));
#41669=DIRECTION('',(0.,-1.,0.));
#41670=DIRECTION('',(0.716064653814028,0.,0.698033961608027));
#41671=DIRECTION('',(0.,1.,0.));
#41672=DIRECTION('',(0.716064653814028,0.,0.698033961608027));
#41673=DIRECTION('center_axis',(-0.698033961608027,0.,0.716064653814028));
#41674=DIRECTION('ref_axis',(0.,1.,0.));
#41675=DIRECTION('',(0.716064653814028,0.,0.698033961608027));
#41676=DIRECTION('',(0.,1.,0.));
#41677=DIRECTION('',(-0.716064653814028,0.,-0.698033961608027));
#41678=DIRECTION('',(0.,1.,0.));
#41679=DIRECTION('',(-0.716064653814028,0.,-0.698033961608027));
#41680=DIRECTION('center_axis',(-0.698033961608027,0.,0.716064653814028));
#41681=DIRECTION('ref_axis',(0.,1.,0.));
#41682=DIRECTION('',(-0.716064653814028,0.,-0.698033961608027));
#41683=DIRECTION('',(0.,1.,0.));
#41684=DIRECTION('',(0.716064653814028,0.,0.698033961608027));
#41685=DIRECTION('',(0.,1.,0.));
#41686=DIRECTION('',(0.716064653814028,0.,0.698033961608027));
#41687=DIRECTION('center_axis',(-0.698033961608027,0.,0.716064653814028));
#41688=DIRECTION('ref_axis',(0.,1.,0.));
#41689=DIRECTION('',(0.716064653814028,0.,0.698033961608027));
#41690=DIRECTION('',(0.,1.,0.));
#41691=DIRECTION('',(-0.716064653814028,0.,-0.698033961608027));
#41692=DIRECTION('',(0.,-1.,0.));
#41693=DIRECTION('center_axis',(-0.698033961608027,0.,-0.716064653814028));
#41694=DIRECTION('ref_axis',(-0.716064653814028,0.,0.698033961608027));
#41695=DIRECTION('',(0.,-1.,0.));
#41696=DIRECTION('',(0.716064653814028,0.,-0.698033961608027));
#41697=DIRECTION('',(0.,1.,0.));
#41698=DIRECTION('',(-0.716064653814028,0.,0.698033961608027));
#41699=DIRECTION('center_axis',(-0.698033961608027,0.,-0.716064653814028));
#41700=DIRECTION('ref_axis',(-0.716064653814028,0.,0.698033961608027));
#41701=DIRECTION('',(-0.716064653814028,0.,0.698033961608027));
#41702=DIRECTION('',(0.,1.,0.));
#41703=DIRECTION('',(-0.716064653814028,0.,0.698033961608027));
#41704=DIRECTION('',(0.,1.,0.));
#41705=DIRECTION('',(0.716064653814028,0.,-0.698033961608027));
#41706=DIRECTION('center_axis',(-0.698033961608027,0.,-0.716064653814028));
#41707=DIRECTION('ref_axis',(-0.716064653814028,0.,0.698033961608027));
#41708=DIRECTION('',(0.716064653814028,0.,-0.698033961608027));
#41709=DIRECTION('',(0.,1.,0.));
#41710=DIRECTION('',(0.716064653814028,0.,-0.698033961608027));
#41711=DIRECTION('',(0.,1.,0.));
#41712=DIRECTION('',(-0.716064653814028,0.,0.698033961608027));
#41713=DIRECTION('center_axis',(-0.698033961608027,0.,-0.716064653814028));
#41714=DIRECTION('ref_axis',(-0.716064653814028,0.,0.698033961608027));
#41715=DIRECTION('',(-0.716064653814028,0.,0.698033961608027));
#41716=DIRECTION('',(0.,1.,0.));
#41717=DIRECTION('',(-0.716064653814028,0.,0.698033961608027));
#41718=DIRECTION('',(0.,-1.,0.));
#41719=DIRECTION('center_axis',(0.,1.,0.));
#41720=DIRECTION('ref_axis',(1.,0.,0.));
#41721=DIRECTION('center_axis',(0.,1.,0.));
#41722=DIRECTION('ref_axis',(1.,0.,0.));
#41723=DIRECTION('center_axis',(0.,1.,0.));
#41724=DIRECTION('ref_axis',(1.,0.,0.));
#41725=DIRECTION('',(0.716064653814028,0.,0.698033961608027));
#41726=DIRECTION('center_axis',(0.,1.,0.));
#41727=DIRECTION('ref_axis',(1.,0.,0.));
#41728=DIRECTION('center_axis',(0.,1.,0.));
#41729=DIRECTION('ref_axis',(1.,0.,0.));
#41730=DIRECTION('center_axis',(0.,1.,0.));
#41731=DIRECTION('ref_axis',(1.,0.,0.));
#41732=DIRECTION('',(-0.698033961608027,0.,-0.716064653814028));
#41733=DIRECTION('center_axis',(0.,1.,0.));
#41734=DIRECTION('ref_axis',(1.,0.,0.));
#41735=DIRECTION('center_axis',(0.,1.,0.));
#41736=DIRECTION('ref_axis',(1.,0.,0.));
#41737=DIRECTION('center_axis',(0.,1.,0.));
#41738=DIRECTION('ref_axis',(1.,0.,0.));
#41739=DIRECTION('center_axis',(0.,1.,0.));
#41740=DIRECTION('ref_axis',(1.,0.,0.));
#41741=DIRECTION('',(0.698033961608027,0.,-0.716064653814028));
#41742=DIRECTION('center_axis',(0.,1.,0.));
#41743=DIRECTION('ref_axis',(1.,0.,0.));
#41744=DIRECTION('center_axis',(0.,1.,0.));
#41745=DIRECTION('ref_axis',(1.,0.,0.));
#41746=DIRECTION('',(0.698033961608027,0.,-0.716064653814028));
#41747=DIRECTION('center_axis',(0.,1.,0.));
#41748=DIRECTION('ref_axis',(1.,0.,0.));
#41749=DIRECTION('',(-0.716064653814028,0.,0.698033961608027));
#41750=DIRECTION('center_axis',(0.,1.,0.));
#41751=DIRECTION('ref_axis',(1.,0.,0.));
#41752=DIRECTION('center_axis',(0.,1.,0.));
#41753=DIRECTION('ref_axis',(1.,0.,0.));
#41754=DIRECTION('',(0.716064653814028,0.,0.698033961608027));
#41755=DIRECTION('center_axis',(0.,1.,0.));
#41756=DIRECTION('ref_axis',(1.,0.,0.));
#41757=DIRECTION('',(-0.698033961608027,0.,-0.716064653814028));
#41758=DIRECTION('center_axis',(0.,1.,0.));
#41759=DIRECTION('ref_axis',(1.,0.,0.));
#41760=DIRECTION('center_axis',(0.,1.,0.));
#41761=DIRECTION('ref_axis',(1.,0.,0.));
#41762=DIRECTION('center_axis',(0.,1.,0.));
#41763=DIRECTION('ref_axis',(1.,0.,0.));
#41764=DIRECTION('center_axis',(0.,1.,0.));
#41765=DIRECTION('ref_axis',(1.,0.,0.));
#41766=DIRECTION('center_axis',(0.,1.,0.));
#41767=DIRECTION('ref_axis',(1.,0.,0.));
#41768=DIRECTION('',(-0.716064653814028,0.,0.698033961608027));
#41769=DIRECTION('center_axis',(0.716064653814028,3.32064561166926E-28,
-0.698033961608027));
#41770=DIRECTION('ref_axis',(-2.37779695035902E-28,1.,2.31792341140981E-28));
#41771=DIRECTION('center_axis',(0.716064653814028,0.,-0.698033961608027));
#41772=DIRECTION('ref_axis',(0.698033961608027,0.,0.716064653814028));
#41773=DIRECTION('center_axis',(0.716064653814028,0.,-0.698033961608027));
#41774=DIRECTION('ref_axis',(0.698033961608027,0.,0.716064653814028));
#41775=DIRECTION('',(0.716064653814028,0.,-0.698033961608027));
#41776=DIRECTION('center_axis',(0.,-1.,0.));
#41777=DIRECTION('ref_axis',(0.803032113208901,0.,-0.595935755895925));
#41778=DIRECTION('center_axis',(0.,1.,0.));
#41779=DIRECTION('ref_axis',(1.,0.,0.));
#41780=DIRECTION('center_axis',(0.,0.,1.));
#41781=DIRECTION('ref_axis',(1.,0.,0.));
#41782=DIRECTION('center_axis',(-0.595935755895926,0.,-0.8030321132089));
#41783=DIRECTION('ref_axis',(0.8030321132089,0.,-0.595935755895926));
#41784=DIRECTION('center_axis',(0.,1.,0.));
#41785=DIRECTION('ref_axis',(-0.716064653814026,0.,0.69803396160803));
#41786=DIRECTION('center_axis',(0.,1.,0.));
#41787=DIRECTION('ref_axis',(1.,0.,0.));
#41788=DIRECTION('',(0.,1.,0.));
#41789=DIRECTION('center_axis',(1.,0.,0.));
#41790=DIRECTION('ref_axis',(0.,-1.,0.));
#41791=DIRECTION('center_axis',(0.698033961608027,0.,0.716064653814028));
#41792=DIRECTION('ref_axis',(0.716064653814028,0.,-0.698033961608027));
#41793=DIRECTION('center_axis',(0.,1.,0.));
#41794=DIRECTION('ref_axis',(0.8030321132089,0.,-0.595935755895926));
#41795=DIRECTION('center_axis',(-0.779809347293264,0.,-0.626017077941212));
#41796=DIRECTION('ref_axis',(0.626017077941212,0.,-0.779809347293264));
#41797=DIRECTION('center_axis',(0.,1.,0.));
#41798=DIRECTION('ref_axis',(1.,0.,0.));
#41799=DIRECTION('center_axis',(0.,1.,0.));
#41800=DIRECTION('ref_axis',(0.626017077941214,0.,-0.779809347293263));
#41801=DIRECTION('center_axis',(0.,1.,0.));
#41802=DIRECTION('ref_axis',(1.,0.,0.));
#41803=DIRECTION('center_axis',(1.,0.,0.));
#41804=DIRECTION('ref_axis',(0.,-1.,0.));
#41805=DIRECTION('center_axis',(-0.716064653814028,0.,0.698033961608027));
#41806=DIRECTION('ref_axis',(0.698033961608027,0.,0.716064653814028));
#41807=DIRECTION('center_axis',(0.,1.,0.));
#41808=DIRECTION('ref_axis',(1.,0.,0.));
#41809=DIRECTION('',(-0.716064653814028,0.,0.698033961608027));
#41810=DIRECTION('',(0.698033961608027,0.,0.716064653814028));
#41811=DIRECTION('',(0.716064653814028,0.,-0.698033961608027));
#41812=DIRECTION('center_axis',(0.,-1.,0.));
#41813=DIRECTION('ref_axis',(1.,0.,0.));
#41814=DIRECTION('center_axis',(0.,-1.,0.));
#41815=DIRECTION('ref_axis',(1.,0.,0.));
#41816=DIRECTION('center_axis',(0.,-1.,0.));
#41817=DIRECTION('ref_axis',(1.,0.,0.));
#41818=DIRECTION('',(-0.716064653814028,0.,0.698033961608027));
#41819=DIRECTION('',(0.698033961608027,0.,0.716064653814028));
#41820=DIRECTION('center_axis',(-0.698033961608027,0.,-0.716064653814028));
#41821=DIRECTION('ref_axis',(-0.716064653814028,0.,0.698033961608027));
#41822=DIRECTION('center_axis',(0.698033961608027,0.,0.716064653814028));
#41823=DIRECTION('ref_axis',(0.716064653814028,0.,-0.698033961608027));
#41824=DIRECTION('',(0.698033961608027,0.,0.716064653814028));
#41825=DIRECTION('center_axis',(0.,0.,1.));
#41826=DIRECTION('ref_axis',(1.,0.,0.));
#41827=DIRECTION('center_axis',(-0.716064653814028,0.,0.698033961608027));
#41828=DIRECTION('ref_axis',(0.698033961608027,0.,0.716064653814028));
#41829=DIRECTION('center_axis',(0.,1.,0.));
#41830=DIRECTION('ref_axis',(1.,0.,0.));
#41831=DIRECTION('center_axis',(0.716064653814028,0.,-0.698033961608027));
#41832=DIRECTION('ref_axis',(-0.698033961608027,0.,-0.716064653814028));
#41833=DIRECTION('center_axis',(-0.716064653814028,0.,0.698033961608027));
#41834=DIRECTION('ref_axis',(0.698033961608027,0.,0.716064653814028));
#41835=DIRECTION('center_axis',(0.,0.,1.));
#41836=DIRECTION('ref_axis',(1.,0.,0.));
#41837=DIRECTION('center_axis',(0.,1.,0.));
#41838=DIRECTION('ref_axis',(1.,0.,0.));
#41839=DIRECTION('center_axis',(0.698033961608027,0.,0.716064653814028));
#41840=DIRECTION('ref_axis',(0.716064653814028,0.,-0.698033961608027));
#41841=DIRECTION('center_axis',(-0.698033961608027,0.,-0.716064653814028));
#41842=DIRECTION('ref_axis',(-0.716064653814028,0.,0.698033961608027));
#41843=DIRECTION('',(0.698033961608027,0.,0.716064653814028));
#41844=DIRECTION('center_axis',(0.698033961608027,0.,0.716064653814028));
#41845=DIRECTION('ref_axis',(0.716064653814028,0.,-0.698033961608027));
#41846=DIRECTION('center_axis',(1.,0.,0.));
#41847=DIRECTION('ref_axis',(0.,-1.,0.));
#41848=DIRECTION('center_axis',(0.,1.,0.));
#41849=DIRECTION('ref_axis',(1.,0.,0.));
#41850=DIRECTION('center_axis',(0.716064653814028,0.,-0.698033961608027));
#41851=DIRECTION('ref_axis',(0.698033961608027,0.,0.716064653814028));
#41852=DIRECTION('center_axis',(0.716064653814028,3.32064561166926E-28,
-0.698033961608027));
#41853=DIRECTION('ref_axis',(-2.37779695035902E-28,1.,2.31792341140981E-28));
#41854=DIRECTION('center_axis',(0.716064653814028,0.,-0.698033961608027));
#41855=DIRECTION('ref_axis',(0.698033961608027,0.,0.716064653814028));
#41856=DIRECTION('center_axis',(0.,1.,0.));
#41857=DIRECTION('ref_axis',(0.67049648912325,0.,-0.741912702461277));
#41858=DIRECTION('center_axis',(0.,-1.,0.));
#41859=DIRECTION('ref_axis',(1.,0.,0.));
#41860=DIRECTION('center_axis',(0.741912702461277,0.,0.67049648912325));
#41861=DIRECTION('ref_axis',(0.67049648912325,0.,-0.741912702461277));
#41862=DIRECTION('center_axis',(0.,1.,0.));
#41863=DIRECTION('ref_axis',(0.767334963051732,0.,-0.641246484963776));
#41864=DIRECTION('center_axis',(0.641246484963776,0.,0.767334963051731));
#41865=DIRECTION('ref_axis',(0.767334963051731,0.,-0.641246484963776));
#41866=DIRECTION('center_axis',(0.,1.,0.));
#41867=DIRECTION('ref_axis',(0.698033961608026,0.,0.716064653814029));
#41868=DIRECTION('center_axis',(0.,-1.,0.));
#41869=DIRECTION('ref_axis',(1.,0.,0.));
#41870=DIRECTION('center_axis',(-0.716064653814028,0.,0.698033961608027));
#41871=DIRECTION('ref_axis',(0.698033961608027,0.,0.716064653814028));
#41872=DIRECTION('center_axis',(0.716064653814028,0.,-0.698033961608027));
#41873=DIRECTION('ref_axis',(-0.698033961608027,0.,-0.716064653814028));
#41874=DIRECTION('center_axis',(0.716064653814028,0.,-0.698033961608027));
#41875=DIRECTION('ref_axis',(0.,-1.,0.));
#41876=DIRECTION('',(0.,1.,0.));
#41877=DIRECTION('center_axis',(0.,1.,0.));
#41878=DIRECTION('ref_axis',(-0.69803396160803,0.,-0.716064653814026));
#41879=DIRECTION('center_axis',(0.,1.,0.));
#41880=DIRECTION('ref_axis',(-0.69803396160803,0.,-0.716064653814026));
#41881=DIRECTION('',(0.,1.,0.));
#41882=DIRECTION('center_axis',(0.716064653814028,0.,-0.698033961608027));
#41883=DIRECTION('ref_axis',(0.,-1.,0.));
#41884=DIRECTION('',(0.,1.,0.));
#41885=DIRECTION('center_axis',(0.,1.,0.));
#41886=DIRECTION('ref_axis',(-0.716064653814028,0.,0.698033961608027));
#41887=DIRECTION('center_axis',(0.,-1.,0.));
#41888=DIRECTION('ref_axis',(-0.698033961608027,0.,-0.716064653814028));
#41889=DIRECTION('center_axis',(0.,1.,0.));
#41890=DIRECTION('ref_axis',(0.698033961608027,0.,0.716064653814028));
#41891=DIRECTION('center_axis',(-0.698033961608027,0.,0.716064653814028));
#41892=DIRECTION('ref_axis',(0.,1.,0.));
#41893=DIRECTION('',(0.,1.,0.));
#41894=DIRECTION('',(0.716064653814028,0.,0.698033961608027));
#41895=DIRECTION('',(0.,1.,0.));
#41896=DIRECTION('center_axis',(0.716064653814028,-3.32064561166926E-28,
0.698033961608027));
#41897=DIRECTION('ref_axis',(2.37779695035902E-28,1.,2.31792341140981E-28));
#41898=DIRECTION('center_axis',(0.716064653814028,0.,0.698033961608027));
#41899=DIRECTION('ref_axis',(0.698033961608027,0.,-0.716064653814028));
#41900=DIRECTION('center_axis',(0.716064653814028,0.,0.698033961608027));
#41901=DIRECTION('ref_axis',(0.698033961608027,0.,-0.716064653814028));
#41902=DIRECTION('',(0.716064653814028,0.,0.698033961608027));
#41903=DIRECTION('center_axis',(0.,-1.,0.));
#41904=DIRECTION('ref_axis',(0.626017077941214,0.,0.779809347293263));
#41905=DIRECTION('center_axis',(0.,1.,0.));
#41906=DIRECTION('ref_axis',(1.,0.,0.));
#41907=DIRECTION('center_axis',(1.,0.,0.));
#41908=DIRECTION('ref_axis',(0.,-1.,0.));
#41909=DIRECTION('center_axis',(0.779809347293264,0.,-0.626017077941212));
#41910=DIRECTION('ref_axis',(0.626017077941212,0.,0.779809347293264));
#41911=DIRECTION('center_axis',(0.,1.,0.));
#41912=DIRECTION('ref_axis',(-0.716064653814026,0.,-0.69803396160803));
#41913=DIRECTION('',(0.,1.,0.));
#41914=DIRECTION('center_axis',(0.,1.,0.));
#41915=DIRECTION('ref_axis',(1.,0.,0.));
#41916=DIRECTION('center_axis',(0.,0.,1.));
#41917=DIRECTION('ref_axis',(1.,0.,0.));
#41918=DIRECTION('center_axis',(-0.698033961608027,0.,0.716064653814028));
#41919=DIRECTION('ref_axis',(0.716064653814028,0.,0.698033961608027));
#41920=DIRECTION('center_axis',(0.,1.,0.));
#41921=DIRECTION('ref_axis',(0.626017077941212,0.,0.779809347293264));
#41922=DIRECTION('center_axis',(0.595935755895926,0.,-0.8030321132089));
#41923=DIRECTION('ref_axis',(0.8030321132089,0.,0.595935755895926));
#41924=DIRECTION('center_axis',(0.,1.,0.));
#41925=DIRECTION('ref_axis',(1.,0.,0.));
#41926=DIRECTION('center_axis',(0.,1.,0.));
#41927=DIRECTION('ref_axis',(0.803032113208901,0.,0.595935755895925));
#41928=DIRECTION('',(0.,1.,0.));
#41929=DIRECTION('center_axis',(0.,1.,0.));
#41930=DIRECTION('ref_axis',(1.,0.,0.));
#41931=DIRECTION('center_axis',(0.,0.,1.));
#41932=DIRECTION('ref_axis',(1.,0.,0.));
#41933=DIRECTION('center_axis',(-0.716064653814028,0.,-0.698033961608027));
#41934=DIRECTION('ref_axis',(0.698033961608027,0.,-0.716064653814028));
#41935=DIRECTION('center_axis',(0.,1.,0.));
#41936=DIRECTION('ref_axis',(1.,0.,0.));
#41937=DIRECTION('',(-0.716064653814028,0.,-0.698033961608027));
#41938=DIRECTION('',(-0.698033961608027,0.,0.716064653814028));
#41939=DIRECTION('',(0.716064653814028,0.,0.698033961608027));
#41940=DIRECTION('center_axis',(0.,-1.,0.));
#41941=DIRECTION('ref_axis',(1.,0.,0.));
#41942=DIRECTION('center_axis',(0.,-1.,0.));
#41943=DIRECTION('ref_axis',(1.,0.,0.));
#41944=DIRECTION('center_axis',(0.,-1.,0.));
#41945=DIRECTION('ref_axis',(1.,0.,0.));
#41946=DIRECTION('',(-0.716064653814028,0.,-0.698033961608027));
#41947=DIRECTION('',(-0.698033961608027,0.,0.716064653814028));
#41948=DIRECTION('center_axis',(-0.698033961608027,-3.32064561166926E-28,
0.716064653814028));
#41949=DIRECTION('ref_axis',(-2.31792341140981E-28,1.,2.37779695035902E-28));
#41950=DIRECTION('center_axis',(-0.698033961608027,0.,0.716064653814028));
#41951=DIRECTION('ref_axis',(0.716064653814028,0.,0.698033961608027));
#41952=DIRECTION('',(-0.698033961608027,0.,0.716064653814028));
#41953=DIRECTION('center_axis',(1.,0.,0.));
#41954=DIRECTION('ref_axis',(0.,-1.,0.));
#41955=DIRECTION('center_axis',(-0.716064653814028,0.,-0.698033961608027));
#41956=DIRECTION('ref_axis',(0.698033961608027,0.,-0.716064653814028));
#41957=DIRECTION('center_axis',(0.,1.,0.));
#41958=DIRECTION('ref_axis',(1.,0.,0.));
#41959=DIRECTION('center_axis',(0.716064653814028,0.,0.698033961608027));
#41960=DIRECTION('ref_axis',(0.698033961608027,0.,-0.716064653814028));
#41961=DIRECTION('',(-0.716064653814028,0.,-0.698033961608027));
#41962=DIRECTION('center_axis',(-0.716064653814028,0.,-0.698033961608027));
#41963=DIRECTION('ref_axis',(0.698033961608027,0.,-0.716064653814028));
#41964=DIRECTION('center_axis',(1.,0.,0.));
#41965=DIRECTION('ref_axis',(0.,-1.,0.));
#41966=DIRECTION('center_axis',(0.,1.,0.));
#41967=DIRECTION('ref_axis',(1.,0.,0.));
#41968=DIRECTION('center_axis',(-0.698033961608027,0.,0.716064653814028));
#41969=DIRECTION('ref_axis',(0.716064653814028,0.,0.698033961608027));
#41970=DIRECTION('center_axis',(-0.698033961608027,-3.32064561166926E-28,
0.716064653814028));
#41971=DIRECTION('ref_axis',(-2.31792341140981E-28,1.,2.37779695035902E-28));
#41972=DIRECTION('',(-0.698033961608027,0.,0.716064653814028));
#41973=DIRECTION('center_axis',(-0.698033961608027,0.,0.716064653814028));
#41974=DIRECTION('ref_axis',(0.716064653814028,0.,0.698033961608027));
#41975=DIRECTION('center_axis',(0.,0.,1.));
#41976=DIRECTION('ref_axis',(1.,0.,0.));
#41977=DIRECTION('center_axis',(0.,1.,0.));
#41978=DIRECTION('ref_axis',(1.,0.,0.));
#41979=DIRECTION('center_axis',(0.716064653814028,0.,0.698033961608027));
#41980=DIRECTION('ref_axis',(0.698033961608027,0.,-0.716064653814028));
#41981=DIRECTION('center_axis',(0.716064653814028,-3.32064561166926E-28,
0.698033961608027));
#41982=DIRECTION('ref_axis',(2.37779695035902E-28,1.,2.31792341140981E-28));
#41983=DIRECTION('',(0.716064653814028,0.,0.698033961608027));
#41984=DIRECTION('center_axis',(0.716064653814028,0.,0.698033961608027));
#41985=DIRECTION('ref_axis',(0.698033961608027,0.,-0.716064653814028));
#41986=DIRECTION('center_axis',(0.,1.,0.));
#41987=DIRECTION('ref_axis',(0.767334963051732,0.,0.641246484963776));
#41988=DIRECTION('center_axis',(0.,-1.,0.));
#41989=DIRECTION('ref_axis',(1.,0.,0.));
#41990=DIRECTION('center_axis',(-0.641246484963776,0.,0.767334963051731));
#41991=DIRECTION('ref_axis',(0.767334963051731,0.,0.641246484963776));
#41992=DIRECTION('center_axis',(0.,1.,0.));
#41993=DIRECTION('ref_axis',(0.67049648912325,0.,0.741912702461277));
#41994=DIRECTION('center_axis',(-0.741912702461277,0.,0.67049648912325));
#41995=DIRECTION('ref_axis',(0.67049648912325,0.,0.741912702461277));
#41996=DIRECTION('center_axis',(0.,1.,0.));
#41997=DIRECTION('ref_axis',(-0.698033961608026,0.,0.716064653814029));
#41998=DIRECTION('center_axis',(0.,-1.,0.));
#41999=DIRECTION('ref_axis',(1.,0.,0.));
#42000=DIRECTION('center_axis',(-0.716064653814028,0.,-0.698033961608027));
#42001=DIRECTION('ref_axis',(0.698033961608027,0.,-0.716064653814028));
#42002=DIRECTION('center_axis',(0.716064653814028,0.,0.698033961608027));
#42003=DIRECTION('ref_axis',(0.698033961608027,0.,-0.716064653814028));
#42004=DIRECTION('',(-0.716064653814028,0.,-0.698033961608027));
#42005=DIRECTION('center_axis',(-0.716064653814028,0.,-0.698033961608027));
#42006=DIRECTION('ref_axis',(-0.698033961608027,0.,0.716064653814028));
#42007=DIRECTION('',(0.,1.,0.));
#42008=DIRECTION('center_axis',(0.,1.,0.));
#42009=DIRECTION('ref_axis',(0.69803396160803,0.,-0.716064653814026));
#42010=DIRECTION('',(0.,1.,0.));
#42011=DIRECTION('center_axis',(-0.698033961608027,0.,0.716064653814028));
#42012=DIRECTION('ref_axis',(0.,1.,0.));
#42013=DIRECTION('',(0.,1.,0.));
#42014=DIRECTION('center_axis',(0.,1.,0.));
#42015=DIRECTION('ref_axis',(0.69803396160803,0.,-0.716064653814026));
#42016=DIRECTION('',(0.,1.,0.));
#42017=DIRECTION('center_axis',(-0.716064653814028,0.,-0.698033961608027));
#42018=DIRECTION('ref_axis',(-0.698033961608027,0.,0.716064653814028));
#42019=DIRECTION('',(0.,1.,0.));
#42020=DIRECTION('center_axis',(0.,1.,0.));
#42021=DIRECTION('ref_axis',(-0.716064653814028,0.,-0.698033961608027));
#42022=DIRECTION('',(0.,1.,0.));
#42023=DIRECTION('center_axis',(-0.698033961608027,0.,0.716064653814028));
#42024=DIRECTION('ref_axis',(0.,1.,0.));
#42025=DIRECTION('',(0.,-1.,0.));
#42026=DIRECTION('center_axis',(0.,-1.,0.));
#42027=DIRECTION('ref_axis',(0.698033961608027,0.,-0.716064653814028));
#42028=DIRECTION('center_axis',(0.,1.,0.));
#42029=DIRECTION('ref_axis',(-0.698033961608027,0.,0.716064653814028));
#42030=DIRECTION('',(0.,-1.,0.));
#42031=DIRECTION('center_axis',(-0.698033961608027,0.,0.716064653814028));
#42032=DIRECTION('ref_axis',(0.,1.,0.));
#42033=DIRECTION('center_axis',(-0.716064653814028,0.,-0.698033961608027));
#42034=DIRECTION('ref_axis',(-0.698033961608027,0.,0.716064653814028));
#42035=DIRECTION('center_axis',(-0.716064653814028,0.,-0.698033961608027));
#42036=DIRECTION('ref_axis',(0.698033961608027,0.,-0.716064653814028));
#42037=DIRECTION('',(-0.716064653814028,0.,-0.698033961608027));
#42038=DIRECTION('center_axis',(-0.716064653814028,0.,-0.698033961608027));
#42039=DIRECTION('ref_axis',(0.698033961608027,0.,-0.716064653814028));
#42040=DIRECTION('center_axis',(0.,1.,0.));
#42041=DIRECTION('ref_axis',(-0.803032113208901,0.,-0.595935755895925));
#42042=DIRECTION('center_axis',(0.,-1.,0.));
#42043=DIRECTION('ref_axis',(1.,0.,0.));
#42044=DIRECTION('center_axis',(0.,0.,1.));
#42045=DIRECTION('ref_axis',(1.,0.,0.));
#42046=DIRECTION('center_axis',(0.595935755895926,0.,-0.8030321132089));
#42047=DIRECTION('ref_axis',(0.8030321132089,0.,0.595935755895926));
#42048=DIRECTION('center_axis',(0.,1.,0.));
#42049=DIRECTION('ref_axis',(-0.69803396160803,0.,0.716064653814026));
#42050=DIRECTION('',(0.,1.,0.));
#42051=DIRECTION('center_axis',(0.,-1.,0.));
#42052=DIRECTION('ref_axis',(1.,0.,0.));
#42053=DIRECTION('center_axis',(1.,0.,0.));
#42054=DIRECTION('ref_axis',(0.,-1.,0.));
#42055=DIRECTION('center_axis',(-0.698033961608027,0.,0.716064653814028));
#42056=DIRECTION('ref_axis',(0.716064653814028,0.,0.698033961608027));
#42057=DIRECTION('center_axis',(0.,1.,0.));
#42058=DIRECTION('ref_axis',(-0.626017077941212,0.,-0.779809347293264));
#42059=DIRECTION('center_axis',(0.,-1.,0.));
#42060=DIRECTION('ref_axis',(1.,0.,0.));
#42061=DIRECTION('center_axis',(0.779809347293264,0.,-0.626017077941212));
#42062=DIRECTION('ref_axis',(0.626017077941212,0.,0.779809347293264));
#42063=DIRECTION('center_axis',(0.,-1.,0.));
#42064=DIRECTION('ref_axis',(-0.626017077941214,0.,-0.779809347293263));
#42065=DIRECTION('center_axis',(0.,-1.,0.));
#42066=DIRECTION('ref_axis',(1.,0.,0.));
#42067=DIRECTION('center_axis',(1.,0.,0.));
#42068=DIRECTION('ref_axis',(0.,-1.,0.));
#42069=DIRECTION('center_axis',(0.716064653814028,0.,0.698033961608027));
#42070=DIRECTION('ref_axis',(0.698033961608027,0.,-0.716064653814028));
#42071=DIRECTION('center_axis',(0.,1.,0.));
#42072=DIRECTION('ref_axis',(1.,0.,0.));
#42073=DIRECTION('',(-0.698033961608027,0.,0.716064653814028));
#42074=DIRECTION('',(0.716064653814028,0.,0.698033961608027));
#42075=DIRECTION('center_axis',(0.,1.,0.));
#42076=DIRECTION('ref_axis',(1.,0.,0.));
#42077=DIRECTION('center_axis',(0.,1.,0.));
#42078=DIRECTION('ref_axis',(1.,0.,0.));
#42079=DIRECTION('center_axis',(0.,1.,0.));
#42080=DIRECTION('ref_axis',(1.,0.,0.));
#42081=DIRECTION('',(-0.716064653814028,0.,-0.698033961608027));
#42082=DIRECTION('',(-0.698033961608027,0.,0.716064653814028));
#42083=DIRECTION('',(0.716064653814028,0.,0.698033961608027));
#42084=DIRECTION('center_axis',(0.698033961608027,0.,-0.716064653814028));
#42085=DIRECTION('ref_axis',(0.,1.,0.));
#42086=DIRECTION('center_axis',(-0.698033961608027,0.,0.716064653814028));
#42087=DIRECTION('ref_axis',(0.716064653814028,0.,0.698033961608027));
#42088=DIRECTION('',(-0.698033961608027,0.,0.716064653814028));
#42089=DIRECTION('center_axis',(0.,0.,1.));
#42090=DIRECTION('ref_axis',(1.,0.,0.));
#42091=DIRECTION('center_axis',(0.716064653814028,0.,0.698033961608027));
#42092=DIRECTION('ref_axis',(0.698033961608027,0.,-0.716064653814028));
#42093=DIRECTION('center_axis',(0.,-1.,0.));
#42094=DIRECTION('ref_axis',(1.,0.,0.));
#42095=DIRECTION('center_axis',(-0.716064653814028,0.,-0.698033961608027));
#42096=DIRECTION('ref_axis',(0.,1.,0.));
#42097=DIRECTION('center_axis',(0.716064653814028,0.,0.698033961608027));
#42098=DIRECTION('ref_axis',(0.698033961608027,0.,-0.716064653814028));
#42099=DIRECTION('center_axis',(0.,0.,1.));
#42100=DIRECTION('ref_axis',(1.,0.,0.));
#42101=DIRECTION('center_axis',(-0.698033961608027,0.,0.716064653814028));
#42102=DIRECTION('ref_axis',(0.716064653814028,0.,0.698033961608027));
#42103=DIRECTION('center_axis',(0.,-1.,0.));
#42104=DIRECTION('ref_axis',(1.,0.,0.));
#42105=DIRECTION('center_axis',(0.698033961608027,0.,-0.716064653814028));
#42106=DIRECTION('ref_axis',(0.,1.,0.));
#42107=DIRECTION('center_axis',(-0.698033961608027,0.,0.716064653814028));
#42108=DIRECTION('ref_axis',(0.716064653814028,0.,0.698033961608027));
#42109=DIRECTION('',(-0.698033961608027,0.,0.716064653814028));
#42110=DIRECTION('center_axis',(1.,0.,0.));
#42111=DIRECTION('ref_axis',(0.,-1.,0.));
#42112=DIRECTION('center_axis',(-0.716064653814028,0.,-0.698033961608027));
#42113=DIRECTION('ref_axis',(0.698033961608027,0.,-0.716064653814028));
#42114=DIRECTION('center_axis',(0.,-1.,0.));
#42115=DIRECTION('ref_axis',(1.,0.,0.));
#42116=DIRECTION('center_axis',(-0.716064653814028,0.,-0.698033961608027));
#42117=DIRECTION('ref_axis',(-0.698033961608027,0.,0.716064653814028));
#42118=DIRECTION('center_axis',(-0.716064653814028,0.,-0.698033961608027));
#42119=DIRECTION('ref_axis',(0.698033961608027,0.,-0.716064653814028));
#42120=DIRECTION('center_axis',(0.,1.,0.));
#42121=DIRECTION('ref_axis',(0.698033961608026,0.,-0.716064653814029));
#42122=DIRECTION('center_axis',(-0.741912702461277,0.,0.67049648912325));
#42123=DIRECTION('ref_axis',(0.67049648912325,0.,0.741912702461277));
#42124=DIRECTION('center_axis',(0.,1.,0.));
#42125=DIRECTION('ref_axis',(1.,0.,0.));
#42126=DIRECTION('center_axis',(0.,1.,0.));
#42127=DIRECTION('ref_axis',(-0.67049648912325,0.,-0.741912702461277));
#42128=DIRECTION('center_axis',(-0.641246484963776,0.,0.767334963051731));
#42129=DIRECTION('ref_axis',(0.767334963051731,0.,0.641246484963776));
#42130=DIRECTION('center_axis',(0.,1.,0.));
#42131=DIRECTION('ref_axis',(-0.767334963051732,0.,-0.641246484963776));
#42132=DIRECTION('center_axis',(0.716064653814028,0.,0.698033961608027));
#42133=DIRECTION('ref_axis',(0.698033961608027,0.,-0.716064653814028));
#42134=DIRECTION('center_axis',(0.,1.,0.));
#42135=DIRECTION('ref_axis',(1.,0.,0.));
#42136=DIRECTION('center_axis',(-0.716064653814028,0.,-0.698033961608027));
#42137=DIRECTION('ref_axis',(0.,1.,0.));
#42138=DIRECTION('center_axis',(0.716064653814028,0.,0.698033961608027));
#42139=DIRECTION('ref_axis',(0.,-1.,0.));
#42140=DIRECTION('',(0.,1.,0.));
#42141=DIRECTION('center_axis',(0.,1.,0.));
#42142=DIRECTION('ref_axis',(0.716064653814028,0.,0.698033961608027));
#42143=DIRECTION('center_axis',(0.,1.,0.));
#42144=DIRECTION('ref_axis',(0.716064653814026,0.,0.69803396160803));
#42145=DIRECTION('',(0.,1.,0.));
#42146=DIRECTION('center_axis',(0.716064653814028,0.,0.698033961608027));
#42147=DIRECTION('ref_axis',(0.,-1.,0.));
#42148=DIRECTION('',(0.,1.,0.));
#42149=DIRECTION('center_axis',(0.,1.,0.));
#42150=DIRECTION('ref_axis',(-0.69803396160803,0.,0.716064653814026));
#42151=DIRECTION('center_axis',(0.,1.,0.));
#42152=DIRECTION('ref_axis',(0.698033961608027,0.,-0.716064653814028));
#42153=DIRECTION('center_axis',(0.,-1.,0.));
#42154=DIRECTION('ref_axis',(-0.698033961608027,0.,0.716064653814028));
#42155=DIRECTION('center_axis',(-0.698033961608027,0.,-0.716064653814028));
#42156=DIRECTION('ref_axis',(-0.716064653814028,0.,0.698033961608027));
#42157=DIRECTION('',(0.,1.,0.));
#42158=DIRECTION('',(-0.716064653814028,0.,0.698033961608027));
#42159=DIRECTION('',(0.,1.,0.));
#42160=DIRECTION('center_axis',(-0.716064653814028,0.,0.698033961608027));
#42161=DIRECTION('ref_axis',(0.698033961608027,0.,0.716064653814028));
#42162=DIRECTION('center_axis',(-0.716064653814028,0.,0.698033961608027));
#42163=DIRECTION('ref_axis',(0.698033961608027,0.,0.716064653814028));
#42164=DIRECTION('',(-0.716064653814028,0.,0.698033961608027));
#42165=DIRECTION('center_axis',(-0.716064653814028,0.,0.698033961608027));
#42166=DIRECTION('ref_axis',(0.698033961608027,0.,0.716064653814028));
#42167=DIRECTION('center_axis',(0.,1.,0.));
#42168=DIRECTION('ref_axis',(0.698033961608027,0.,0.716064653814028));
#42169=DIRECTION('',(0.,1.,0.));
#42170=DIRECTION('center_axis',(0.,-1.,0.));
#42171=DIRECTION('ref_axis',(1.,0.,0.));
#42172=DIRECTION('center_axis',(0.,0.,1.));
#42173=DIRECTION('ref_axis',(1.,0.,0.));
#42174=DIRECTION('center_axis',(0.698033961608027,0.,0.716064653814028));
#42175=DIRECTION('ref_axis',(0.716064653814028,0.,-0.698033961608027));
#42176=DIRECTION('center_axis',(0.,1.,0.));
#42177=DIRECTION('ref_axis',(-0.601264366509671,0.,0.799050162108565));
#42178=DIRECTION('center_axis',(0.,-1.,0.));
#42179=DIRECTION('ref_axis',(1.,0.,0.));
#42180=DIRECTION('center_axis',(1.,0.,0.));
#42181=DIRECTION('ref_axis',(0.,-1.,0.));
#42182=DIRECTION('center_axis',(-0.799050162108564,0.,-0.601264366509672));
#42183=DIRECTION('ref_axis',(0.601264366509672,0.,-0.799050162108564));
#42184=DIRECTION('center_axis',(0.,1.,0.));
#42185=DIRECTION('ref_axis',(1.,0.,0.));
#42186=DIRECTION('',(0.698033961608027,0.,0.716064653814028));
#42187=DIRECTION('',(0.716064653814028,0.,-0.698033961608027));
#42188=DIRECTION('center_axis',(0.,1.,0.));
#42189=DIRECTION('ref_axis',(1.,0.,0.));
#42190=DIRECTION('center_axis',(0.,1.,0.));
#42191=DIRECTION('ref_axis',(1.,0.,0.));
#42192=DIRECTION('center_axis',(0.,1.,0.));
#42193=DIRECTION('ref_axis',(1.,0.,0.));
#42194=DIRECTION('',(-0.716064653814028,0.,0.698033961608027));
#42195=DIRECTION('',(0.698033961608027,0.,0.716064653814028));
#42196=DIRECTION('',(0.716064653814028,0.,-0.698033961608027));
#42197=DIRECTION('center_axis',(0.,-1.,0.));
#42198=DIRECTION('ref_axis',(1.,0.,0.));
#42199=DIRECTION('center_axis',(0.698033961608027,0.,0.716064653814028));
#42200=DIRECTION('ref_axis',(0.716064653814028,0.,-0.698033961608027));
#42201=DIRECTION('center_axis',(0.698033961608027,0.,0.716064653814028));
#42202=DIRECTION('ref_axis',(0.716064653814028,0.,-0.698033961608027));
#42203=DIRECTION('',(0.698033961608027,0.,0.716064653814028));
#42204=DIRECTION('center_axis',(1.,0.,0.));
#42205=DIRECTION('ref_axis',(0.,-1.,0.));
#42206=DIRECTION('center_axis',(0.716064653814028,0.,-0.698033961608027));
#42207=DIRECTION('ref_axis',(0.698033961608027,0.,0.716064653814028));
#42208=DIRECTION('center_axis',(0.,-1.,0.));
#42209=DIRECTION('ref_axis',(1.,0.,0.));
#42210=DIRECTION('center_axis',(0.,1.,0.));
#42211=DIRECTION('ref_axis',(-0.821350998880235,0.,0.570423120708164));
#42212=DIRECTION('center_axis',(-0.570423120708163,0.,-0.821350998880235));
#42213=DIRECTION('ref_axis',(0.821350998880235,0.,-0.570423120708163));
#42214=DIRECTION('center_axis',(0.,0.,1.));
#42215=DIRECTION('ref_axis',(1.,0.,0.));
#42216=DIRECTION('center_axis',(0.716064653814028,0.,-0.698033961608027));
#42217=DIRECTION('ref_axis',(0.698033961608027,0.,0.716064653814028));
#42218=DIRECTION('center_axis',(0.,-1.,0.));
#42219=DIRECTION('ref_axis',(1.,0.,0.));
#42220=DIRECTION('center_axis',(0.698033961608027,0.,0.716064653814028));
#42221=DIRECTION('ref_axis',(0.716064653814028,0.,-0.698033961608027));
#42222=DIRECTION('center_axis',(0.698033961608027,0.,0.716064653814028));
#42223=DIRECTION('ref_axis',(0.716064653814028,0.,-0.698033961608027));
#42224=DIRECTION('center_axis',(0.698033961608027,0.,0.716064653814028));
#42225=DIRECTION('ref_axis',(0.716064653814028,0.,-0.698033961608027));
#42226=DIRECTION('',(0.698033961608027,0.,0.716064653814028));
#42227=DIRECTION('center_axis',(1.,0.,0.));
#42228=DIRECTION('ref_axis',(0.,-1.,0.));
#42229=DIRECTION('center_axis',(0.716064653814028,0.,-0.698033961608027));
#42230=DIRECTION('ref_axis',(0.698033961608027,0.,0.716064653814028));
#42231=DIRECTION('center_axis',(0.,-1.,0.));
#42232=DIRECTION('ref_axis',(1.,0.,0.));
#42233=DIRECTION('center_axis',(0.,0.,1.));
#42234=DIRECTION('ref_axis',(1.,0.,0.));
#42235=DIRECTION('center_axis',(-0.716064653814028,0.,0.698033961608027));
#42236=DIRECTION('ref_axis',(0.698033961608027,0.,0.716064653814028));
#42237=DIRECTION('center_axis',(0.,-1.,0.));
#42238=DIRECTION('ref_axis',(1.,0.,0.));
#42239=DIRECTION('center_axis',(-0.716064653814028,0.,0.698033961608027));
#42240=DIRECTION('ref_axis',(0.,1.,0.));
#42241=DIRECTION('',(0.716064653814028,0.,-0.698033961608027));
#42242=DIRECTION('center_axis',(-0.716064653814028,0.,0.698033961608027));
#42243=DIRECTION('ref_axis',(0.698033961608027,0.,0.716064653814028));
#42244=DIRECTION('center_axis',(-0.716064653814028,0.,0.698033961608027));
#42245=DIRECTION('ref_axis',(0.698033961608027,0.,0.716064653814028));
#42246=DIRECTION('',(-0.716064653814028,0.,0.698033961608027));
#42247=DIRECTION('center_axis',(0.,1.,0.));
#42248=DIRECTION('ref_axis',(-0.698033961608026,0.,-0.716064653814029));
#42249=DIRECTION('center_axis',(0.615376309981942,0.,0.788233466120926));
#42250=DIRECTION('ref_axis',(0.788233466120926,0.,-0.615376309981942));
#42251=DIRECTION('center_axis',(0.,1.,0.));
#42252=DIRECTION('ref_axis',(1.,0.,0.));
#42253=DIRECTION('center_axis',(0.,1.,0.));
#42254=DIRECTION('ref_axis',(-0.788233466120926,0.,0.615376309981942));
#42255=DIRECTION('center_axis',(0.763773184102633,0.,0.645484719606689));
#42256=DIRECTION('ref_axis',(0.645484719606689,0.,-0.763773184102633));
#42257=DIRECTION('center_axis',(0.,1.,0.));
#42258=DIRECTION('ref_axis',(-0.645484719606688,0.,0.763773184102634));
#42259=DIRECTION('center_axis',(0.716064653814028,0.,-0.698033961608027));
#42260=DIRECTION('ref_axis',(0.698033961608027,0.,0.716064653814028));
#42261=DIRECTION('center_axis',(0.,1.,0.));
#42262=DIRECTION('ref_axis',(1.,0.,0.));
#42263=DIRECTION('center_axis',(-0.716064653814028,0.,0.698033961608027));
#42264=DIRECTION('ref_axis',(0.,1.,0.));
#42265=DIRECTION('',(0.716064653814028,0.,-0.698033961608027));
#42266=DIRECTION('center_axis',(-0.716064653814028,0.,0.698033961608027));
#42267=DIRECTION('ref_axis',(0.,1.,0.));
#42268=DIRECTION('',(0.,1.,0.));
#42269=DIRECTION('center_axis',(0.,1.,0.));
#42270=DIRECTION('ref_axis',(0.716064653814028,0.,-0.698033961608027));
#42271=DIRECTION('',(0.,1.,0.));
#42272=DIRECTION('center_axis',(0.,-1.,0.));
#42273=DIRECTION('ref_axis',(-0.821350998880237,0.,0.570423120708161));
#42274=DIRECTION('',(0.,1.,0.));
#42275=DIRECTION('center_axis',(-0.716064653814028,0.,0.698033961608027));
#42276=DIRECTION('ref_axis',(0.,1.,0.));
#42277=DIRECTION('',(0.,1.,0.));
#42278=DIRECTION('',(0.,1.,0.));
#42279=DIRECTION('center_axis',(0.,1.,0.));
#42280=DIRECTION('ref_axis',(0.716064653814027,0.,-0.698033961608028));
#42281=DIRECTION('',(0.,1.,0.));
#42282=DIRECTION('center_axis',(0.,1.,0.));
#42283=DIRECTION('ref_axis',(0.69803396160803,0.,0.716064653814026));
#42284=DIRECTION('',(0.,1.,0.));
#42285=DIRECTION('center_axis',(-0.698033961608027,0.,-0.716064653814028));
#42286=DIRECTION('ref_axis',(-0.716064653814028,0.,0.698033961608027));
#42287=DIRECTION('center_axis',(-0.698033961608027,0.,-0.716064653814028));
#42288=DIRECTION('ref_axis',(-0.716064653814028,0.,0.698033961608027));
#42289=DIRECTION('',(0.,-1.,0.));
#42290=DIRECTION('center_axis',(0.,1.,0.));
#42291=DIRECTION('ref_axis',(-0.698033961608027,0.,-0.716064653814028));
#42292=DIRECTION('center_axis',(0.,-1.,0.));
#42293=DIRECTION('ref_axis',(0.69803396160803,0.,0.716064653814026));
#42294=DIRECTION('',(0.,-1.,0.));
#42295=DIRECTION('center_axis',(-0.698033961608027,0.,-0.716064653814028));
#42296=DIRECTION('ref_axis',(-0.716064653814028,0.,0.698033961608027));
#74301=CARTESIAN_POINT('',(0.,0.,0.));
#74302=CARTESIAN_POINT('Origin',(-3.35265884719E-30,-38.2742356128,3.15283103411E-22));
#74303=CARTESIAN_POINT('',(-2.02924878182,-38.2742356128,-3.59534899368));
#74304=CARTESIAN_POINT('',(-1.71727342606,-38.2742356128,-3.85789277743));
#74305=CARTESIAN_POINT('Ctrl Pts',(-2.02924878182,-38.2742356128,-3.59534899368));
#74306=CARTESIAN_POINT('Ctrl Pts',(-1.93266642605,-38.2742356128,-3.68930297977));
#74307=CARTESIAN_POINT('Ctrl Pts',(-1.82884081082,-38.2742356128,-3.77671908511));
#74308=CARTESIAN_POINT('Ctrl Pts',(-1.71727342605654,-38.2742356128,-3.85789277742524));
#74309=CARTESIAN_POINT('',(-1.71727342606,-38.2742356128,-3.68636669298));
#74310=CARTESIAN_POINT('',(-1.71727342606,-38.2742356128,0.));
#74311=CARTESIAN_POINT('Origin',(4.8544501751735E-13,-38.2742356128,2.77999550541204));
#74312=CARTESIAN_POINT('Origin',(-6.28286804938E-15,-37.6642356128,2.77999550541));
#74313=CARTESIAN_POINT('',(-2.02924878182,-39.7742356128,-3.59534899368));
#74314=CARTESIAN_POINT('',(-2.02924878182,-38.7792356128,-3.59534899368));
#74315=CARTESIAN_POINT('',(-1.71727342606,-39.7742356128,-3.68636669298));
#74316=CARTESIAN_POINT('',(-1.71727342606,-38.7792356128,-3.68636669298));
#74317=CARTESIAN_POINT('Origin',(-6.28286804938E-15,-39.7742356128,2.77999550541));
#74318=CARTESIAN_POINT('Origin',(-1.71727342606,-39.2742356128,-2.86512409447));
#74319=CARTESIAN_POINT('',(-1.71727342606,-39.7742356128,-3.85789277743));
#74320=CARTESIAN_POINT('',(-1.71727342606,-38.2792356128,-3.85789277743));
#74321=CARTESIAN_POINT('',(-1.71727342606,-39.7742356128,-5.61958386968));
#74322=CARTESIAN_POINT('Ctrl Pts',(-2.02924878182,-39.7742356128,-3.59534899368));
#74323=CARTESIAN_POINT('Ctrl Pts',(-2.02924878182,-37.9742356128,-3.59534899368));
#74324=CARTESIAN_POINT('Ctrl Pts',(-1.93266642605,-39.7742356128,-3.68930297977));
#74325=CARTESIAN_POINT('Ctrl Pts',(-1.93266642605,-37.9742356128,-3.68930297977));
#74326=CARTESIAN_POINT('Ctrl Pts',(-1.82884081082,-39.7742356128,-3.77671908511));
#74327=CARTESIAN_POINT('Ctrl Pts',(-1.82884081082,-37.9742356128,-3.77671908511));
#74328=CARTESIAN_POINT('Ctrl Pts',(-1.71727342605,-39.7742356128,-3.85789277743));
#74329=CARTESIAN_POINT('Ctrl Pts',(-1.71727342605,-37.9742356128,-3.85789277743));
#74330=CARTESIAN_POINT('Ctrl Pts',(-2.02924878182,-39.7742356128,-3.59534899368));
#74331=CARTESIAN_POINT('Ctrl Pts',(-1.93266642605,-39.7742356128,-3.68930297977));
#74332=CARTESIAN_POINT('Ctrl Pts',(-1.82884081082,-39.7742356128,-3.77671908511));
#74333=CARTESIAN_POINT('Ctrl Pts',(-1.71727342605654,-39.7742356128,-3.85789277742524));
#74334=CARTESIAN_POINT('Origin',(-3.35265884719E-30,-39.7742356128,3.15283103411E-22));
#74335=CARTESIAN_POINT('Origin',(-3.35265884719E-30,-38.2742356128,3.15283103411E-22));
#74336=CARTESIAN_POINT('',(2.02924878231356,-38.2742356128,-3.59534899352193));
#74337=CARTESIAN_POINT('',(1.71727342605667,-38.2742356128,-3.85789277798081));
#74338=CARTESIAN_POINT('Ctrl Pts',(2.02924878182,-38.2742356128,-3.59534899368));
#74339=CARTESIAN_POINT('Ctrl Pts',(1.93266642605,-38.2742356128,-3.68930297977));
#74340=CARTESIAN_POINT('Ctrl Pts',(1.82884081082,-38.2742356128,-3.77671908511));
#74341=CARTESIAN_POINT('Ctrl Pts',(1.71727342605,-38.2742356128,-3.85789277743));
#74342=CARTESIAN_POINT('',(1.71727342606,-38.2742356128,-3.68636669298));
#74343=CARTESIAN_POINT('Origin',(-3.60822483003176E-15,-38.2742356128,2.7799955054097));
#74344=CARTESIAN_POINT('',(1.71727342606,-38.2742356128,0.));
#74345=CARTESIAN_POINT('Origin',(1.71727342606,-39.2742356128,-2.86512409447));
#74346=CARTESIAN_POINT('',(1.71727342606,-39.7742356128,-3.68636669298));
#74347=CARTESIAN_POINT('',(1.71727342606,-38.2792356128,-3.68636669298));
#74348=CARTESIAN_POINT('',(1.71727342606,-39.7742356128,-3.85789277743));
#74349=CARTESIAN_POINT('',(1.71727342606,-39.7742356128,-5.61958386968));
#74350=CARTESIAN_POINT('',(1.71727342606,-38.2792356128,-3.85789277743));
#74351=CARTESIAN_POINT('Origin',(6.28286804938E-15,-37.6642356128,2.77999550541));
#74352=CARTESIAN_POINT('',(2.02924878182,-39.7742356128,-3.59534899368));
#74353=CARTESIAN_POINT('',(2.02924878182,-38.7792356128,-3.59534899368));
#74354=CARTESIAN_POINT('Origin',(6.28286804938E-15,-39.7742356128,2.77999550541));
#74355=CARTESIAN_POINT('Ctrl Pts',(2.02924878182,-39.7742356128,-3.59534899368));
#74356=CARTESIAN_POINT('Ctrl Pts',(2.02924878182,-37.9742356128,-3.59534899368));
#74357=CARTESIAN_POINT('Ctrl Pts',(1.93266642605,-39.7742356128,-3.68930297977));
#74358=CARTESIAN_POINT('Ctrl Pts',(1.93266642605,-37.9742356128,-3.68930297977));
#74359=CARTESIAN_POINT('Ctrl Pts',(1.82884081082,-39.7742356128,-3.77671908511));
#74360=CARTESIAN_POINT('Ctrl Pts',(1.82884081082,-37.9742356128,-3.77671908511));
#74361=CARTESIAN_POINT('Ctrl Pts',(1.71727342605,-39.7742356128,-3.85789277743));
#74362=CARTESIAN_POINT('Ctrl Pts',(1.71727342605,-37.9742356128,-3.85789277743));
#74363=CARTESIAN_POINT('Ctrl Pts',(2.02924878182,-39.7742356128,-3.59534899368));
#74364=CARTESIAN_POINT('Ctrl Pts',(1.93266642605,-39.7742356128,-3.68930297977));
#74365=CARTESIAN_POINT('Ctrl Pts',(1.82884081082,-39.7742356128,-3.77671908511));
#74366=CARTESIAN_POINT('Ctrl Pts',(1.71727342605654,-39.7742356128,-3.85789277742524));
#74367=CARTESIAN_POINT('Origin',(-3.35265884719E-30,-39.7742356128,3.15283103411E-22));
#74368=CARTESIAN_POINT('Origin',(0.000416107150126,-40.1142356128,6.92091963994));
#74369=CARTESIAN_POINT('',(4.44384247076,-41.6742356128,6.92091963994));
#74370=CARTESIAN_POINT('',(-0.000416107140392043,-41.6742356128,11.3643459775889));
#74371=CARTESIAN_POINT('Origin',(0.000416107150126,-41.6742356128,6.92091963994));
#74372=CARTESIAN_POINT('',(-0.000416107136785584,-39.7742356128,11.3643459650651));
#74373=CARTESIAN_POINT('',(-0.000416107150125,-40.1142356128,11.3643460036));
#74374=CARTESIAN_POINT('',(3.64378781517,-39.7742356128,9.46451560746));
#74375=CARTESIAN_POINT('Origin',(0.000416107150126,-39.7742356128,6.92091963994));
#74376=CARTESIAN_POINT('',(4.44384247076,-39.7742356128,6.92091963994));
#74377=CARTESIAN_POINT('Origin',(0.000416107150126,-39.7742356128,6.92091963994));
#74378=CARTESIAN_POINT('',(4.44384247076,-40.1142356128,6.92091963994));
#74379=CARTESIAN_POINT('Origin',(-0.000416107150126,-40.1142356128,6.92091963994));
#74380=CARTESIAN_POINT('',(0.000416107143369473,-40.6742356128,13.1643459761606));
#74381=CARTESIAN_POINT('',(-6.24384247076,-40.6742356128,6.92091963994));
#74382=CARTESIAN_POINT('Origin',(-0.000416107150126,-40.6742356128,6.92091963994));
#74383=CARTESIAN_POINT('',(0.000416107145187488,-41.6742356128,13.1643459850784));
#74384=CARTESIAN_POINT('',(0.000416107150124,-40.1142356128,13.1643460036));
#74385=CARTESIAN_POINT('',(-6.24384247076,-41.6742356128,6.92091963994));
#74386=CARTESIAN_POINT('Origin',(-0.000416107150126,-41.6742356128,6.92091963994));
#74387=CARTESIAN_POINT('',(-6.24384247076,-40.1142356128,6.92091963994));
#74388=CARTESIAN_POINT('Origin',(6.86146892388,-41.6742356128,4.85630581709));
#74389=CARTESIAN_POINT('',(7.34384247076,-41.6742356128,5.03150262953));
#74390=CARTESIAN_POINT('',(7.34384247076,-39.7742356128,5.03150262895));
#74391=CARTESIAN_POINT('',(7.34384247076,-40.7242356128,5.03150262895));
#74392=CARTESIAN_POINT('',(13.5647513306,-39.7742356128,7.2909204726));
#74393=CARTESIAN_POINT('',(10.4542969007,-39.7742356128,6.16121155078));
#74394=CARTESIAN_POINT('',(14.2293511975,-39.7742356128,7.53230140778));
#74395=CARTESIAN_POINT('',(13.8970512641,-39.7742356128,7.41161094019));
#74396=CARTESIAN_POINT('',(14.2293511975,-41.6742356128,7.53230140778));
#74397=CARTESIAN_POINT('',(14.2293511975,-40.7242356128,7.53230140778));
#74398=CARTESIAN_POINT('',(10.7865968341,-41.6742356128,6.28190201837));
#74399=CARTESIAN_POINT('Origin',(-3.35265884719E-30,-41.6742356128,3.15283103411E-22));
#74400=CARTESIAN_POINT('',(-16.2234398325,-41.6742356128,-2.4));
#74401=CARTESIAN_POINT('',(-17.2336839201,-41.6742356128,-2.4));
#74402=CARTESIAN_POINT('',(-16.7285618762,-41.6742356128,-2.4));
#74403=CARTESIAN_POINT('',(-17.0705772097,-41.6742356128,-3.4));
#74404=CARTESIAN_POINT('Ctrl Pts',(-17.0705772097,-41.6742356128,-3.4));
#74405=CARTESIAN_POINT('Ctrl Pts',(-17.1142405474,-41.6742356128,-3.15603772018));
#74406=CARTESIAN_POINT('Ctrl Pts',(-17.1569007064,-41.6742356128,-2.91066121221));
#74407=CARTESIAN_POINT('Ctrl Pts',(-17.1980377987,-41.6742356128,-2.65606214167));
#74408=CARTESIAN_POINT('Ctrl Pts',(-17.2336839201,-41.6742356128,-2.4));
#74409=CARTESIAN_POINT('',(-17.0645832062,-41.6742356128,-3.4));
#74410=CARTESIAN_POINT('',(-17.067580208,-41.6742356128,-3.4));
#74411=CARTESIAN_POINT('',(17.0645832062,-41.6742356128,-3.4));
#74412=CARTESIAN_POINT('Origin',(-3.5527136788E-15,-41.6742356128,-8.88178104417E-16));
#74413=CARTESIAN_POINT('',(17.0705772097,-41.6742356128,-3.4));
#74414=CARTESIAN_POINT('',(17.067580208,-41.6742356128,-3.4));
#74415=CARTESIAN_POINT('',(17.2336839201,-41.6742356128,-2.4));
#74416=CARTESIAN_POINT('Ctrl Pts',(17.0705772097,-41.6742356128,-3.4));
#74417=CARTESIAN_POINT('Ctrl Pts',(17.1142405474,-41.6742356128,-3.15603772018));
#74418=CARTESIAN_POINT('Ctrl Pts',(17.1569007064,-41.6742356128,-2.91066121221));
#74419=CARTESIAN_POINT('Ctrl Pts',(17.1980377987,-41.6742356128,-2.65606214167));
#74420=CARTESIAN_POINT('Ctrl Pts',(17.2336839201,-41.6742356128,-2.39999999999));
#74421=CARTESIAN_POINT('',(16.2234398325,-41.6742356128,-2.4));
#74422=CARTESIAN_POINT('',(16.7285618762,-41.6742356128,-2.4));
#74423=CARTESIAN_POINT('',(16.2234398325,-41.6742356128,2.4));
#74424=CARTESIAN_POINT('Origin',(-3.35265884719E-30,-41.6742356128,3.15283103411E-22));
#74425=CARTESIAN_POINT('',(17.2336839201,-41.6742356128,2.4));
#74426=CARTESIAN_POINT('',(16.7285618762,-41.6742356128,2.4));
#74427=CARTESIAN_POINT('',(17.0705772096,-41.6742356128,3.4));
#74428=CARTESIAN_POINT('Ctrl Pts',(17.2336839201,-41.6742356128,2.39999999999));
#74429=CARTESIAN_POINT('Ctrl Pts',(17.1980377987,-41.6742356128,2.65606214167));
#74430=CARTESIAN_POINT('Ctrl Pts',(17.1569007064,-41.6742356128,2.91066121221));
#74431=CARTESIAN_POINT('Ctrl Pts',(17.1142405474,-41.6742356128,3.15603772019));
#74432=CARTESIAN_POINT('Ctrl Pts',(17.0705772097,-41.6742356128,3.40000000002));
#74433=CARTESIAN_POINT('',(17.0645832062,-41.6742356128,3.4));
#74434=CARTESIAN_POINT('',(17.0675802079,-41.6742356128,3.4));
#74435=CARTESIAN_POINT('',(-17.0645832062,-41.6742356128,3.4));
#74436=CARTESIAN_POINT('Origin',(-3.5527136788E-15,-41.6742356128,-8.88178104417E-16));
#74437=CARTESIAN_POINT('',(-17.0705772096,-41.6742356128,3.4));
#74438=CARTESIAN_POINT('',(-17.0675802079,-41.6742356128,3.4));
#74439=CARTESIAN_POINT('',(-17.2336839201,-41.6742356128,2.4));
#74440=CARTESIAN_POINT('Ctrl Pts',(-17.2336839201,-41.6742356128,2.39999999999));
#74441=CARTESIAN_POINT('Ctrl Pts',(-17.1980377987,-41.6742356128,2.65606214167));
#74442=CARTESIAN_POINT('Ctrl Pts',(-17.1569007064,-41.6742356128,2.91066121221));
#74443=CARTESIAN_POINT('Ctrl Pts',(-17.1142405474,-41.6742356128,3.15603772019));
#74444=CARTESIAN_POINT('Ctrl Pts',(-17.0705772097,-41.6742356128,3.40000000002));
#74445=CARTESIAN_POINT('',(-16.2234398325,-41.6742356128,2.4));
#74446=CARTESIAN_POINT('',(-16.7285618762,-41.6742356128,2.4));
#74447=CARTESIAN_POINT('Origin',(-3.35265884719E-30,-41.6742356128,3.15283103411E-22));
#74448=CARTESIAN_POINT('',(-14.4212065313,-41.6742356128,-3.4));
#74449=CARTESIAN_POINT('',(-15.7368993134,-41.6742356128,-3.4));
#74450=CARTESIAN_POINT('',(-15.0790529224,-41.6742356128,-3.4));
#74451=CARTESIAN_POINT('',(-0.174946252184,-41.6742356128,-7.24363497156));
#74452=CARTESIAN_POINT('Origin',(-6.82290383517,-41.6742356128,-3.56061176027));
#74453=CARTESIAN_POINT('',(0.174946252184,-41.6742356128,-7.24363497156));
#74454=CARTESIAN_POINT('Origin',(1.44328993201E-15,-41.6742356128,-7.34055663501));
#74455=CARTESIAN_POINT('',(14.4212065313,-41.6742356128,-3.4));
#74456=CARTESIAN_POINT('Origin',(6.82290383517,-41.6742356128,-3.56061176027));
#74457=CARTESIAN_POINT('',(15.7368993134,-41.6742356128,-3.4));
#74458=CARTESIAN_POINT('',(15.0790529224,-41.6742356128,-3.4));
#74459=CARTESIAN_POINT('Origin',(-3.5527136788E-15,-41.6742356128,-8.88178104417E-16));
#74460=CARTESIAN_POINT('',(-7.52535686472,-41.6742356128,4.00685543432));
#74461=CARTESIAN_POINT('',(-7.34384247076,-41.6742356128,4.20599930786));
#74462=CARTESIAN_POINT('Origin',(-7.54384247076,-41.6742356128,4.20599930786));
#74463=CARTESIAN_POINT('',(-14.2514385284,-41.6742356128,-1.95534782199));
#74464=CARTESIAN_POINT('Origin',(-6.82290383517,-41.6742356128,-3.56061176027));
#74465=CARTESIAN_POINT('',(-14.251438528,-41.6742356128,3.4));
#74466=CARTESIAN_POINT('',(-14.2514385284,-41.6742356128,0.722326088933));
#74467=CARTESIAN_POINT('',(-15.7368993134,-41.6742356128,3.4));
#74468=CARTESIAN_POINT('',(-14.9941689207,-41.6742356128,3.4));
#74469=CARTESIAN_POINT('',(-14.2293511975,-41.6742356128,7.53230140778));
#74470=CARTESIAN_POINT('Origin',(-3.5527136788E-15,-41.6742356128,-8.88178104417E-16));
#74471=CARTESIAN_POINT('',(-7.34384247076,-41.6742356128,5.03150262953));
#74472=CARTESIAN_POINT('',(-10.7865968341,-41.6742356128,6.28190201837));
#74473=CARTESIAN_POINT('',(-7.34384247076,-41.6742356128,4.61875096898));
#74474=CARTESIAN_POINT('',(15.7368993134,-41.6742356128,3.4));
#74475=CARTESIAN_POINT('',(14.251438528,-41.6742356128,3.4));
#74476=CARTESIAN_POINT('',(14.9941689207,-41.6742356128,3.4));
#74477=CARTESIAN_POINT('',(14.2514385284,-41.6742356128,-1.95534782199));
#74478=CARTESIAN_POINT('',(14.2514385284,-41.6742356128,0.722326088933));
#74479=CARTESIAN_POINT('',(7.52535686472,-41.6742356128,4.00685543432));
#74480=CARTESIAN_POINT('Origin',(6.82290383517,-41.6742356128,-3.56061176027));
#74481=CARTESIAN_POINT('',(7.34384247076,-41.6742356128,4.20599930843));
#74482=CARTESIAN_POINT('Origin',(7.54384247076,-41.6742356128,4.20599930786));
#74483=CARTESIAN_POINT('',(7.34384247076,-41.6742356128,4.61875096898));
#74484=CARTESIAN_POINT('Origin',(-3.5527136788E-15,-41.6742356128,-8.88178104417E-16));
#74485=CARTESIAN_POINT('',(-5.26789531411,-41.6742356128,12.0375174903));
#74486=CARTESIAN_POINT('',(-6.88660115785,-41.6742356128,9.47167760676));
#74487=CARTESIAN_POINT('Origin',(-7.48272894647,-41.6742356128,11.6412701168));
#74488=CARTESIAN_POINT('',(-7.34384247076,-41.6742356128,6.92091963994));
#74489=CARTESIAN_POINT('Origin',(-0.000416107150126,-41.6742356128,6.92091963994));
#74490=CARTESIAN_POINT('',(-7.34384247076,-41.6742356128,6.09541632061));
#74491=CARTESIAN_POINT('',(-7.34384247076,-41.6742356128,6.50816798058));
#74492=CARTESIAN_POINT('',(-13.7266446428,-41.6742356128,8.41363339168));
#74493=CARTESIAN_POINT('',(-10.5352435568,-41.6742356128,7.25452485585));
#74494=CARTESIAN_POINT('',(-0.5,-41.6742356128,16.0922341519));
#74495=CARTESIAN_POINT('Origin',(-3.5527136788E-15,-41.6742356128,-8.88178104417E-16));
#74496=CARTESIAN_POINT('',(-0.5,-41.6742356128,14.2473325884));
#74497=CARTESIAN_POINT('',(-0.5,-41.6742356128,15.1697833702));
#74498=CARTESIAN_POINT('Origin',(-0.000416107150126,-41.6742356128,6.92091963994));
#74499=CARTESIAN_POINT('',(6.24384247076,-41.6742356128,6.92091963994));
#74500=CARTESIAN_POINT('',(6.24384247076,-41.6742356128,3.43894174696));
#74501=CARTESIAN_POINT('',(6.24384247076,-41.6742356128,5.17993069345));
#74502=CARTESIAN_POINT('',(6.74948971107,-41.6742356128,2.9389736393));
#74503=CARTESIAN_POINT('Origin',(6.74384247076,-41.6742356128,3.43894174696));
#74504=CARTESIAN_POINT('',(0.4871654368,-41.6742356128,-5.0126513422));
#74505=CARTESIAN_POINT('Origin',(6.82290383517,-41.6742356128,-3.56061176027));
#74506=CARTESIAN_POINT('',(0.000199055245640775,-41.6742356128,-4.62434677356992));
#74507=CARTESIAN_POINT('Origin',(-0.000199055382223,-41.6742356128,-5.12434669465));
#74508=CARTESIAN_POINT('',(-0.4871654368,-41.6742356128,-5.0126513422));
#74509=CARTESIAN_POINT('Origin',(0.000199055382222,-41.6742356128,-5.12434669465));
#74510=CARTESIAN_POINT('',(-6.74948971107,-41.6742356128,2.9389736393));
#74511=CARTESIAN_POINT('Origin',(-6.82290383517,-41.6742356128,-3.56061176027));
#74512=CARTESIAN_POINT('',(-6.24384247076,-41.6742356128,3.43894174696));
#74513=CARTESIAN_POINT('Origin',(-6.74384247076,-41.6742356128,3.43894174696));
#74514=CARTESIAN_POINT('',(-6.24384247076,-41.6742356128,5.17993069345));
#74515=CARTESIAN_POINT('Origin',(0.000416107150126,-41.6742356128,6.92091963994));
#74516=CARTESIAN_POINT('',(6.88660115785,-41.6742356128,9.47167760676));
#74517=CARTESIAN_POINT('',(5.26789531411,-41.6742356128,12.0375174903));
#74518=CARTESIAN_POINT('Origin',(7.48272894647,-41.6742356128,11.6412701168));
#74519=CARTESIAN_POINT('',(0.5,-41.6742356128,14.2473325884));
#74520=CARTESIAN_POINT('Origin',(0.000416107150126,-41.6742356128,6.92091963994));
#74521=CARTESIAN_POINT('',(0.5,-41.6742356128,16.0922341519));
#74522=CARTESIAN_POINT('',(0.5,-41.6742356128,15.1697833702));
#74523=CARTESIAN_POINT('',(13.7266446428,-41.6742356128,8.41363339168));
#74524=CARTESIAN_POINT('Origin',(-3.5527136788E-15,-41.6742356128,-8.88178104417E-16));
#74525=CARTESIAN_POINT('',(7.34384247076,-41.6742356128,6.09541632061));
#74526=CARTESIAN_POINT('',(10.5352435568,-41.6742356128,7.25452485585));
#74527=CARTESIAN_POINT('',(7.34384247076,-41.6742356128,6.92091963994));
#74528=CARTESIAN_POINT('',(7.34384247076,-41.6742356128,6.50816798058));
#74529=CARTESIAN_POINT('Origin',(0.000416107150126,-41.6742356128,6.92091963994));
#74530=CARTESIAN_POINT('Origin',(-3.5527136788E-15,-37.9242356128,-8.88178104417E-16));
#74531=CARTESIAN_POINT('',(15.7368993134,-39.7742356128,3.4));
#74532=CARTESIAN_POINT('Origin',(-3.5527136788E-15,-39.7742356128,-8.88178104417E-16));
#74533=CARTESIAN_POINT('',(15.7368993134,-40.7242356128,3.4));
#74534=CARTESIAN_POINT('Origin',(-3.35265884719E-30,-39.7742356128,3.15283103411E-22));
#74535=CARTESIAN_POINT('',(15.0199866844,-39.7742356128,3.4));
#74536=CARTESIAN_POINT('Origin',(3.59850171506006,-39.7742356128,1.3458683859422));
#74537=CARTESIAN_POINT('',(-3.5527136788E-15,-39.7742356128,3.4));
#74538=CARTESIAN_POINT('Origin',(-3.35265884719E-30,-39.7742356128,3.15283103411E-22));
#74539=CARTESIAN_POINT('',(7.34384247076,-39.7742356128,4.25491502787));
#74540=CARTESIAN_POINT('',(7.34384247076,-39.7742356128,0.717649133781));
#74541=CARTESIAN_POINT('',(7.4311653291,-39.7742356128,4.27488229452));
#74542=CARTESIAN_POINT('Origin',(7.20379737320062,-39.7742356128,5.068302267313));
#74543=CARTESIAN_POINT('',(9.78216646656,-39.7742356128,3.43958571397));
#74544=CARTESIAN_POINT('Ctrl Pts',(9.78216646656,-39.7742356128,3.43958571397));
#74545=CARTESIAN_POINT('Ctrl Pts',(9.44950651023,-39.7742356128,3.84219609922));
#74546=CARTESIAN_POINT('Ctrl Pts',(9.03618230028,-39.7742356128,4.19379483572));
#74547=CARTESIAN_POINT('Ctrl Pts',(8.49317585373,-39.7742356128,4.40265075658));
#74548=CARTESIAN_POINT('Ctrl Pts',(7.94364631071,-39.7742356128,4.41424876979));
#74549=CARTESIAN_POINT('Ctrl Pts',(7.4311653291,-39.7742356128,4.27488229452));
#74550=CARTESIAN_POINT('',(14.2514385284,-39.7742356128,-1.95534782207));
#74551=CARTESIAN_POINT('Origin',(6.82290383517001,-39.7742356128,-3.56061176026998));
#74552=CARTESIAN_POINT('',(14.2514385284,-39.7742356128,3.4));
#74553=CARTESIAN_POINT('',(14.2514385284,-39.7742356128,0.717649133781));
#74554=CARTESIAN_POINT('',(0.,-39.7742356128,3.4));
#74555=CARTESIAN_POINT('Origin',(7.34384247076,-41.6742356128,6.92091963994));
#74556=CARTESIAN_POINT('',(7.34384247076,-39.7742356128,4.20599930786));
#74557=CARTESIAN_POINT('',(7.34384247076,-40.7242356128,4.20599930786));
#74558=CARTESIAN_POINT('',(7.34384247076,-39.7742356128,5.5634594739));
#74559=CARTESIAN_POINT('Origin',(-3.35265884719E-30,-38.2742356128,3.15283103411E-22));
#74560=CARTESIAN_POINT('',(-9.86073561073,-37.2742356128,13.1044226585));
#74561=CARTESIAN_POINT('',(-9.86073561073,-33.7742356128,13.1044226585));
#74562=CARTESIAN_POINT('',(-9.86073561073,-38.2742356128,13.1044226585));
#74563=CARTESIAN_POINT('',(-13.4701563816,-33.7742356128,9.35493917959));
#74564=CARTESIAN_POINT('Origin',(-3.35265884719E-30,-33.7742356128,3.15283103411E-22));
#74565=CARTESIAN_POINT('',(-13.4701563816,-37.2742356128,9.35493917959));
#74566=CARTESIAN_POINT('',(-13.4701563816,-38.2742356128,9.35493917959));
#74567=CARTESIAN_POINT('',(-16.2234398325,-37.2742356128,2.4));
#74568=CARTESIAN_POINT('Origin',(-3.35265884719E-30,-37.2742356128,3.15283103411E-22));
#74569=CARTESIAN_POINT('',(-16.2234398325,-34.4742356128,2.4));
#74570=CARTESIAN_POINT('',(-16.2234398325,-38.2742356128,2.4));
#74571=CARTESIAN_POINT('',(-16.2234398325,-34.4742356128,-2.4));
#74572=CARTESIAN_POINT('Origin',(-3.35265884719E-30,-34.4742356128,3.15283103411E-22));
#74573=CARTESIAN_POINT('',(-16.2234398325,-37.2742356128,-2.4));
#74574=CARTESIAN_POINT('',(-16.2234398325,-38.2742356128,-2.4));
#74575=CARTESIAN_POINT('',(-13.1697266566,-37.2742356128,-9.77334639667));
#74576=CARTESIAN_POINT('Origin',(-3.35265884719E-30,-37.2742356128,3.15283103411E-22));
#74577=CARTESIAN_POINT('',(-13.1697266566,-33.7742356128,-9.77334639667));
#74578=CARTESIAN_POINT('',(-13.1697266566,-38.2742356128,-9.77334639667));
#74579=CARTESIAN_POINT('',(-10.2666800782,-33.7742356128,-12.7888732956));
#74580=CARTESIAN_POINT('Origin',(-3.35265884719E-30,-33.7742356128,3.15283103411E-22));
#74581=CARTESIAN_POINT('',(-10.2666800782,-37.2742356128,-12.7888732956));
#74582=CARTESIAN_POINT('',(-10.2666800782,-38.2742356128,-12.7888732956));
#74583=CARTESIAN_POINT('',(-4.7,-37.2742356128,-15.7120972502));
#74584=CARTESIAN_POINT('Origin',(-3.35265884719E-30,-37.2742356128,3.15283103411E-22));
#74585=CARTESIAN_POINT('',(-4.7,-39.2742356128,-15.7120972502));
#74586=CARTESIAN_POINT('',(-4.7,-38.2742356128,-15.7120972502));
#74587=CARTESIAN_POINT('',(-16.2234398325,-39.2742356128,-2.4));
#74588=CARTESIAN_POINT('Origin',(-3.35265884719E-30,-39.2742356128,3.15283103411E-22));
#74589=CARTESIAN_POINT('',(-16.2234398325,-38.2742356128,-2.4));
#74590=CARTESIAN_POINT('',(-16.2234398325,-39.2742356128,2.4));
#74591=CARTESIAN_POINT('',(-16.2234398325,-38.2742356128,2.4));
#74592=CARTESIAN_POINT('',(-3.7,-39.2742356128,15.9771712139));
#74593=CARTESIAN_POINT('Origin',(-3.35265884719E-30,-39.2742356128,3.15283103411E-22));
#74594=CARTESIAN_POINT('',(-3.7,-37.2742356128,15.9771712139));
#74595=CARTESIAN_POINT('',(-3.7,-38.2742356128,15.9771712139));
#74596=CARTESIAN_POINT('Origin',(-3.35265884719E-30,-37.2742356128,3.15283103411E-22));
#74597=CARTESIAN_POINT('Origin',(-16.2234398325,-41.6742356128,2.4));
#74598=CARTESIAN_POINT('',(-17.2336839201,-39.2742356128,2.4));
#74599=CARTESIAN_POINT('',(-17.2336839201,-40.4742356128,2.4));
#74600=CARTESIAN_POINT('',(-16.2433767578,-39.2742356128,2.4));
#74601=CARTESIAN_POINT('Ctrl Pts',(-17.2336839201,-41.6742356128,2.39999999999));
#74602=CARTESIAN_POINT('Ctrl Pts',(-17.2336839201,-38.7942356128,2.39999999999));
#74603=CARTESIAN_POINT('Ctrl Pts',(-17.1980377987,-41.6742356128,2.65606214167));
#74604=CARTESIAN_POINT('Ctrl Pts',(-17.1980377987,-38.7942356128,2.65606214167));
#74605=CARTESIAN_POINT('Ctrl Pts',(-17.1569007064,-41.6742356128,2.91066121221));
#74606=CARTESIAN_POINT('Ctrl Pts',(-17.1569007064,-38.7942356128,2.91066121221));
#74607=CARTESIAN_POINT('Ctrl Pts',(-17.1142405474,-41.6742356128,3.15603772019));
#74608=CARTESIAN_POINT('Ctrl Pts',(-17.1142405474,-38.7942356128,3.15603772019));
#74609=CARTESIAN_POINT('Ctrl Pts',(-17.0705772097,-41.6742356128,3.40000000002));
#74610=CARTESIAN_POINT('Ctrl Pts',(-17.0705772097,-38.7942356128,3.40000000002));
#74611=CARTESIAN_POINT('',(-17.0705772096,-39.2742356128,3.4));
#74612=CARTESIAN_POINT('',(-17.0705772097,-40.4742356128,3.4));
#74613=CARTESIAN_POINT('Ctrl Pts',(-17.2336839201,-39.2742356128,2.39999999999));
#74614=CARTESIAN_POINT('Ctrl Pts',(-17.1980377987,-39.2742356128,2.65606214167));
#74615=CARTESIAN_POINT('Ctrl Pts',(-17.1569007064,-39.2742356128,2.91066121221));
#74616=CARTESIAN_POINT('Ctrl Pts',(-17.1142405474,-39.2742356128,3.15603772019));
#74617=CARTESIAN_POINT('Ctrl Pts',(-17.0705772097,-39.2742356128,3.40000000002));
#74618=CARTESIAN_POINT('Origin',(-16.2234398325,-41.6742356128,3.4));
#74619=CARTESIAN_POINT('',(-17.0645832062,-39.2742356128,3.4));
#74620=CARTESIAN_POINT('',(-15.6610078691,-39.2742356128,3.4));
#74621=CARTESIAN_POINT('',(-17.0645832062,-40.4742356128,3.4));
#74622=CARTESIAN_POINT('Origin',(-3.5527136788E-15,-37.9242356128,-8.88178104417E-16));
#74623=CARTESIAN_POINT('',(17.0645832062,-39.2742356128,3.4));
#74624=CARTESIAN_POINT('',(17.0645832062,-37.9242356128,3.4));
#74625=CARTESIAN_POINT('',(3.7,-39.2742356128,17.0020586989));
#74626=CARTESIAN_POINT('Origin',(-3.5527136788E-15,-39.2742356128,-8.88178104417E-16));
#74627=CARTESIAN_POINT('',(3.7,-35.1742356128,17.0020586989));
#74628=CARTESIAN_POINT('',(3.7,-36.7242356128,17.0020586989));
#74629=CARTESIAN_POINT('',(3.,-34.4742356128,17.1394282285));
#74630=CARTESIAN_POINT('Ctrl Pts',(3.,-34.4742356128,17.1394282285028));
#74631=CARTESIAN_POINT('Ctrl Pts',(3.08822072668697,-34.4742356128001,17.1239865126806));
#74632=CARTESIAN_POINT('Ctrl Pts',(3.18225911112969,-34.4919134675103,17.1067526995575));
#74633=CARTESIAN_POINT('Ctrl Pts',(3.35531488240593,-34.5638806129857,17.0736528901812));
#74634=CARTESIAN_POINT('Ctrl Pts',(3.43433873884385,-34.6181717006057,17.0578246368735));
#74635=CARTESIAN_POINT('Ctrl Pts',(3.55804988739417,-34.7427937550804,17.0324452764604));
#74636=CARTESIAN_POINT('Ctrl Pts',(3.61145665151433,-34.8210247498864,17.021125060463));
#74637=CARTESIAN_POINT('Ctrl Pts',(3.68243822155749,-34.9928100970052,17.0059097439477));
#74638=CARTESIAN_POINT('Ctrl Pts',(3.7,-35.0863737311305,17.0020586988753));
#74639=CARTESIAN_POINT('Ctrl Pts',(3.7,-35.1742356128,17.0020586988753));
#74640=CARTESIAN_POINT('',(-3.,-34.4742356128,17.1394282285));
#74641=CARTESIAN_POINT('Origin',(-3.35265884719E-30,-34.4742356128,3.15283103411E-22));
#74642=CARTESIAN_POINT('',(-3.7,-35.1742356128,17.0020586989));
#74643=CARTESIAN_POINT('Ctrl Pts',(-3.7,-35.1742356128,17.0020586988753));
#74644=CARTESIAN_POINT('Ctrl Pts',(-3.7,-35.0863737311305,17.0020586988753));
#74645=CARTESIAN_POINT('Ctrl Pts',(-3.68243822155749,-34.9928100970052,
17.0059097439477));
#74646=CARTESIAN_POINT('Ctrl Pts',(-3.61145665151433,-34.8210247498864,
17.021125060463));
#74647=CARTESIAN_POINT('Ctrl Pts',(-3.55804988739417,-34.7427937550804,
17.0324452764604));
#74648=CARTESIAN_POINT('Ctrl Pts',(-3.43433873884385,-34.6181717006057,
17.0578246368735));
#74649=CARTESIAN_POINT('Ctrl Pts',(-3.35531488240592,-34.5638806129857,
17.0736528901812));
#74650=CARTESIAN_POINT('Ctrl Pts',(-3.18225911112969,-34.4919134675103,
17.1067526995575));
#74651=CARTESIAN_POINT('Ctrl Pts',(-3.08822072668697,-34.4742356128,17.1239865126806));
#74652=CARTESIAN_POINT('Ctrl Pts',(-3.,-34.4742356128,17.1394282285028));
#74653=CARTESIAN_POINT('',(-3.7,-39.2742356128,17.0020586989));
#74654=CARTESIAN_POINT('',(-3.7,-37.2242356128,17.0020586989));
#74655=CARTESIAN_POINT('Origin',(-3.5527136788E-15,-39.2742356128,-8.88178104417E-16));
#74656=CARTESIAN_POINT('Origin',(-16.2234398325,-41.6742356128,3.4));
#74657=CARTESIAN_POINT('',(17.0705772096,-39.2742356128,3.4));
#74658=CARTESIAN_POINT('',(17.0705772097,-40.4742356128,3.4));
#74659=CARTESIAN_POINT('',(-15.6610078691,-39.2742356128,3.4));
#74660=CARTESIAN_POINT('Ctrl Pts',(17.2336839201,-41.6742356128,2.39999999999));
#74661=CARTESIAN_POINT('Ctrl Pts',(17.2336839201,-38.7942356128,2.39999999999));
#74662=CARTESIAN_POINT('Ctrl Pts',(17.1980377987,-41.6742356128,2.65606214167));
#74663=CARTESIAN_POINT('Ctrl Pts',(17.1980377987,-38.7942356128,2.65606214167));
#74664=CARTESIAN_POINT('Ctrl Pts',(17.1569007064,-41.6742356128,2.91066121221));
#74665=CARTESIAN_POINT('Ctrl Pts',(17.1569007064,-38.7942356128,2.91066121221));
#74666=CARTESIAN_POINT('Ctrl Pts',(17.1142405474,-41.6742356128,3.15603772019));
#74667=CARTESIAN_POINT('Ctrl Pts',(17.1142405474,-38.7942356128,3.15603772019));
#74668=CARTESIAN_POINT('Ctrl Pts',(17.0705772097,-41.6742356128,3.40000000002));
#74669=CARTESIAN_POINT('Ctrl Pts',(17.0705772097,-38.7942356128,3.40000000002));
#74670=CARTESIAN_POINT('',(17.2336839201,-39.2742356128,2.4));
#74671=CARTESIAN_POINT('',(17.2336839201,-40.4742356128,2.4));
#74672=CARTESIAN_POINT('Ctrl Pts',(17.2336839201,-39.2742356128,2.39999999999));
#74673=CARTESIAN_POINT('Ctrl Pts',(17.1980377987,-39.2742356128,2.65606214167));
#74674=CARTESIAN_POINT('Ctrl Pts',(17.1569007064,-39.2742356128,2.91066121221));
#74675=CARTESIAN_POINT('Ctrl Pts',(17.1142405474,-39.2742356128,3.15603772019));
#74676=CARTESIAN_POINT('Ctrl Pts',(17.0705772097,-39.2742356128,3.40000000002));
#74677=CARTESIAN_POINT('Origin',(-16.2234398325,-41.6742356128,2.4));
#74678=CARTESIAN_POINT('',(16.2234398325,-39.2742356128,2.4));
#74679=CARTESIAN_POINT('',(16.2234398325,-40.4742356128,2.4));
#74680=CARTESIAN_POINT('',(-16.2433767578,-39.2742356128,2.4));
#74681=CARTESIAN_POINT('Origin',(-3.35265884719E-30,-38.2742356128,3.15283103411E-22));
#74682=CARTESIAN_POINT('',(10.2666800782,-37.2742356128,-12.7888732956));
#74683=CARTESIAN_POINT('',(10.2666800782,-33.7742356128,-12.7888732956));
#74684=CARTESIAN_POINT('',(10.2666800782,-38.2742356128,-12.7888732956));
#74685=CARTESIAN_POINT('',(13.1697266566,-33.7742356128,-9.77334639667));
#74686=CARTESIAN_POINT('Origin',(-3.35265884719E-30,-33.7742356128,3.15283103411E-22));
#74687=CARTESIAN_POINT('',(13.1697266566,-37.2742356128,-9.77334639667));
#74688=CARTESIAN_POINT('',(13.1697266566,-38.2742356128,-9.77334639667));
#74689=CARTESIAN_POINT('',(16.2234398325,-37.2742356128,-2.4));
#74690=CARTESIAN_POINT('Origin',(-3.35265884719E-30,-37.2742356128,3.15283103411E-22));
#74691=CARTESIAN_POINT('',(16.2234398325,-34.4742356128,-2.4));
#74692=CARTESIAN_POINT('',(16.2234398325,-38.2742356128,-2.4));
#74693=CARTESIAN_POINT('',(16.2234398325,-34.4742356128,2.4));
#74694=CARTESIAN_POINT('Origin',(-3.35265884719E-30,-34.4742356128,3.15283103411E-22));
#74695=CARTESIAN_POINT('',(16.2234398325,-37.2742356128,2.4));
#74696=CARTESIAN_POINT('',(16.2234398325,-38.2742356128,2.4));
#74697=CARTESIAN_POINT('',(13.1697266566,-37.2742356128,9.77334639667));
#74698=CARTESIAN_POINT('Origin',(-3.35265884719E-30,-37.2742356128,3.15283103411E-22));
#74699=CARTESIAN_POINT('',(13.1697266566,-33.7742356128,9.77334639667));
#74700=CARTESIAN_POINT('',(13.1697266566,-38.2742356128,9.77334639667));
#74701=CARTESIAN_POINT('',(10.2666800782,-33.7742356128,12.7888732956));
#74702=CARTESIAN_POINT('Origin',(-3.35265884719E-30,-33.7742356128,3.15283103411E-22));
#74703=CARTESIAN_POINT('',(10.2666800782,-37.2742356128,12.7888732956));
#74704=CARTESIAN_POINT('',(10.2666800782,-38.2742356128,12.7888732956));
#74705=CARTESIAN_POINT('',(3.7,-37.2742356128,15.977171214));
#74706=CARTESIAN_POINT('Origin',(-3.35265884719E-30,-37.2742356128,3.15283103411E-22));
#74707=CARTESIAN_POINT('',(3.7,-39.2742356128,15.9771712139));
#74708=CARTESIAN_POINT('',(3.7,-38.2742356128,15.9771712139));
#74709=CARTESIAN_POINT('Origin',(-3.35265884719E-30,-39.2742356128,3.15283103411E-22));
#74710=CARTESIAN_POINT('',(16.2234398325,-39.2742356128,-2.4));
#74711=CARTESIAN_POINT('',(16.2234398325,-38.2742356128,-2.4));
#74712=CARTESIAN_POINT('',(4.7,-39.2742356128,-15.7120972502));
#74713=CARTESIAN_POINT('Origin',(-3.35265884719E-30,-39.2742356128,3.15283103411E-22));
#74714=CARTESIAN_POINT('',(4.7,-37.2742356128,-15.7120972502));
#74715=CARTESIAN_POINT('',(4.7,-38.2742356128,-15.7120972502));
#74716=CARTESIAN_POINT('Origin',(-3.35265884719E-30,-37.2742356128,3.15283103411E-22));
#74717=CARTESIAN_POINT('Origin',(-14.2514385284,-41.6742356128,-2.4));
#74718=CARTESIAN_POINT('',(17.2336839201,-39.2742356128,-2.4));
#74719=CARTESIAN_POINT('',(17.2336839201,-40.4742356128,-2.4));
#74720=CARTESIAN_POINT('',(-16.2433767578,-39.2742356128,-2.4));
#74721=CARTESIAN_POINT('Ctrl Pts',(17.0705772097,-41.6742356128,-3.4));
#74722=CARTESIAN_POINT('Ctrl Pts',(17.0705772097,-38.7942356128,-3.4));
#74723=CARTESIAN_POINT('Ctrl Pts',(17.1142405474,-41.6742356128,-3.15603772018));
#74724=CARTESIAN_POINT('Ctrl Pts',(17.1142405474,-38.7942356128,-3.15603772018));
#74725=CARTESIAN_POINT('Ctrl Pts',(17.1569007064,-41.6742356128,-2.91066121221));
#74726=CARTESIAN_POINT('Ctrl Pts',(17.1569007064,-38.7942356128,-2.91066121221));
#74727=CARTESIAN_POINT('Ctrl Pts',(17.1980377987,-41.6742356128,-2.65606214167));
#74728=CARTESIAN_POINT('Ctrl Pts',(17.1980377987,-38.7942356128,-2.65606214167));
#74729=CARTESIAN_POINT('Ctrl Pts',(17.2336839201,-41.6742356128,-2.39999999999));
#74730=CARTESIAN_POINT('Ctrl Pts',(17.2336839201,-38.7942356128,-2.39999999999));
#74731=CARTESIAN_POINT('',(17.0705772097,-39.2742356128,-3.4));
#74732=CARTESIAN_POINT('',(17.0705772097,-40.4742356128,-3.4));
#74733=CARTESIAN_POINT('Ctrl Pts',(17.0705772097,-39.2742356128,-3.4));
#74734=CARTESIAN_POINT('Ctrl Pts',(17.1142405474,-39.2742356128,-3.15603772018));
#74735=CARTESIAN_POINT('Ctrl Pts',(17.1569007064,-39.2742356128,-2.91066121221));
#74736=CARTESIAN_POINT('Ctrl Pts',(17.1980377987,-39.2742356128,-2.65606214167));
#74737=CARTESIAN_POINT('Ctrl Pts',(17.2336839201,-39.2742356128,-2.39999999999));
#74738=CARTESIAN_POINT('Origin',(-14.2514385284,-41.6742356128,-3.4));
#74739=CARTESIAN_POINT('',(17.0645832063,-39.2742356128,-3.4));
#74740=CARTESIAN_POINT('',(-15.6610078691,-39.2742356128,-3.4));
#74741=CARTESIAN_POINT('',(17.0645832062,-40.4742356128,-3.4));
#74742=CARTESIAN_POINT('Origin',(-3.5527136788E-15,-37.9242356128,-8.88178104417E-16));
#74743=CARTESIAN_POINT('',(-17.0645832063,-39.2742356128,-3.4));
#74744=CARTESIAN_POINT('',(-17.0645832062,-37.9242356128,-3.4));
#74745=CARTESIAN_POINT('',(-4.7,-39.2742356128,-16.7532086479));
#74746=CARTESIAN_POINT('Origin',(-3.5527136788E-15,-39.2742356128,-8.88178104417E-16));
#74747=CARTESIAN_POINT('',(-4.7,-35.1742356128,-16.7532086479));
#74748=CARTESIAN_POINT('',(-4.7,-37.9242356128,-16.7532086479));
#74749=CARTESIAN_POINT('',(-4.,-34.4742356128,-16.9339894886));
#74750=CARTESIAN_POINT('Ctrl Pts',(-4.,-34.4742356128,-16.9339894885996));
#74751=CARTESIAN_POINT('Ctrl Pts',(-4.08836998503334,-34.4742356128,-16.9131154978385));
#74752=CARTESIAN_POINT('Ctrl Pts',(-4.18258473523978,-34.4919628383768,
-16.8900560280459));
#74753=CARTESIAN_POINT('Ctrl Pts',(-4.35608524188229,-34.5642875640868,
-16.8461428541903));
#74754=CARTESIAN_POINT('Ctrl Pts',(-4.43537858782587,-34.6188898563745,
-16.8253270374741));
#74755=CARTESIAN_POINT('Ctrl Pts',(-4.55872416788887,-34.74379828014,-16.7923189265584));
#74756=CARTESIAN_POINT('Ctrl Pts',(-4.61180004333827,-34.8216954565953,
-16.7777425183049));
#74757=CARTESIAN_POINT('Ctrl Pts',(-4.68244878672198,-34.9929968204804,
-16.7581626981184));
#74758=CARTESIAN_POINT('Ctrl Pts',(-4.7,-35.0864155763189,-16.7532086478979));
#74759=CARTESIAN_POINT('Ctrl Pts',(-4.7,-35.1742356128,-16.7532086478979));
#74760=CARTESIAN_POINT('',(4.,-34.4742356128,-16.9339894886));
#74761=CARTESIAN_POINT('Origin',(-3.5527136788E-15,-34.4742356128,-8.88178104417E-16));
#74762=CARTESIAN_POINT('',(4.7,-35.1742356128,-16.7532086479));
#74763=CARTESIAN_POINT('Ctrl Pts',(4.7,-35.1742356128,-16.7532086478979));
#74764=CARTESIAN_POINT('Ctrl Pts',(4.7,-35.0864155763189,-16.7532086478979));
#74765=CARTESIAN_POINT('Ctrl Pts',(4.68244878672198,-34.9929968204804,-16.7581626981184));
#74766=CARTESIAN_POINT('Ctrl Pts',(4.61180004333826,-34.8216954565953,-16.7777425183049));
#74767=CARTESIAN_POINT('Ctrl Pts',(4.55872416788887,-34.74379828014,-16.7923189265584));
#74768=CARTESIAN_POINT('Ctrl Pts',(4.43537858782587,-34.6188898563745,-16.8253270374741));
#74769=CARTESIAN_POINT('Ctrl Pts',(4.35608524188229,-34.5642875640868,-16.8461428541903));
#74770=CARTESIAN_POINT('Ctrl Pts',(4.18258473523978,-34.4919628383767,-16.8900560280459));
#74771=CARTESIAN_POINT('Ctrl Pts',(4.08836998503334,-34.4742356128,-16.9131154978385));
#74772=CARTESIAN_POINT('Ctrl Pts',(4.,-34.4742356128,-16.9339894885995));
#74773=CARTESIAN_POINT('',(4.7,-39.2742356128,-16.7532086479));
#74774=CARTESIAN_POINT('',(4.7,-37.9242356128,-16.7532086479));
#74775=CARTESIAN_POINT('Origin',(-3.5527136788E-15,-39.2742356128,-8.88178104417E-16));
#74776=CARTESIAN_POINT('Origin',(-14.2514385284,-41.6742356128,-3.4));
#74777=CARTESIAN_POINT('',(-17.0705772097,-39.2742356128,-3.4));
#74778=CARTESIAN_POINT('',(-17.0705772097,-40.4742356128,-3.4));
#74779=CARTESIAN_POINT('',(-15.6610078691,-39.2742356128,-3.4));
#74780=CARTESIAN_POINT('Ctrl Pts',(-17.0705772097,-41.6742356128,-3.4));
#74781=CARTESIAN_POINT('Ctrl Pts',(-17.0705772097,-38.7942356128,-3.4));
#74782=CARTESIAN_POINT('Ctrl Pts',(-17.1142405474,-41.6742356128,-3.15603772018));
#74783=CARTESIAN_POINT('Ctrl Pts',(-17.1142405474,-38.7942356128,-3.15603772018));
#74784=CARTESIAN_POINT('Ctrl Pts',(-17.1569007064,-41.6742356128,-2.91066121221));
#74785=CARTESIAN_POINT('Ctrl Pts',(-17.1569007064,-38.7942356128,-2.91066121221));
#74786=CARTESIAN_POINT('Ctrl Pts',(-17.1980377987,-41.6742356128,-2.65606214167));
#74787=CARTESIAN_POINT('Ctrl Pts',(-17.1980377987,-38.7942356128,-2.65606214167));
#74788=CARTESIAN_POINT('Ctrl Pts',(-17.2336839201,-41.6742356128,-2.39999999999));
#74789=CARTESIAN_POINT('Ctrl Pts',(-17.2336839201,-38.7942356128,-2.39999999999));
#74790=CARTESIAN_POINT('',(-17.2336839201,-39.2742356128,-2.4));
#74791=CARTESIAN_POINT('Ctrl Pts',(-17.0705772097,-39.2742356128,-3.4));
#74792=CARTESIAN_POINT('Ctrl Pts',(-17.1142405474,-39.2742356128,-3.15603772018));
#74793=CARTESIAN_POINT('Ctrl Pts',(-17.1569007064,-39.2742356128,-2.91066121221));
#74794=CARTESIAN_POINT('Ctrl Pts',(-17.1980377987,-39.2742356128,-2.65606214167));
#74795=CARTESIAN_POINT('Ctrl Pts',(-17.2336839201,-39.2742356128,-2.39999999999));
#74796=CARTESIAN_POINT('',(-17.2336839201,-40.4742356128,-2.4));
#74797=CARTESIAN_POINT('Origin',(-14.2514385284,-41.6742356128,-2.4));
#74798=CARTESIAN_POINT('',(-16.2433767578,-39.2742356128,-2.4));
#74799=CARTESIAN_POINT('Origin',(-3.5527136788E-15,-37.9242356128,-8.88178104417E-16));
#74800=CARTESIAN_POINT('',(-15.7368993134,-39.7742356128,-3.4));
#74801=CARTESIAN_POINT('',(-15.7368993134,-40.7242356128,-3.4));
#74802=CARTESIAN_POINT('',(15.7368993134,-39.7742356128,-3.4));
#74803=CARTESIAN_POINT('',(15.7368993134,-40.7242356128,-3.4));
#74804=CARTESIAN_POINT('',(3.7,-39.7742356128,-15.6690778286));
#74805=CARTESIAN_POINT('Origin',(-3.5527136788E-15,-39.7742356128,-8.88178104417E-16));
#74806=CARTESIAN_POINT('',(-3.7,-39.7742356128,-15.6690778286));
#74807=CARTESIAN_POINT('Origin',(-3.5527136788E-15,-39.7742356128,-8.88178104417E-16));
#74808=CARTESIAN_POINT('Origin',(-3.5527136788E-15,-39.7742356128,-8.88178104417E-16));
#74809=CARTESIAN_POINT('Origin',(-14.2514385284,-41.6742356128,-3.4));
#74810=CARTESIAN_POINT('',(14.4212065313,-39.7742356128,-3.4));
#74811=CARTESIAN_POINT('',(14.4212065313,-40.4742356128,-3.4));
#74812=CARTESIAN_POINT('',(15.0199866844,-39.7742356128,-3.4));
#74813=CARTESIAN_POINT('',(-15.6610078691,-39.7742356128,-3.4));
#74814=CARTESIAN_POINT('',(-15.6610078691,-39.7742356128,-3.4));
#74815=CARTESIAN_POINT('Origin',(6.82290383517,-40.1142356128,-3.56061176027));
#74816=CARTESIAN_POINT('',(0.174946252184,-39.7742356128,-7.24363497156));
#74817=CARTESIAN_POINT('',(0.174946252184,-40.7242356128,-7.24363497156));
#74818=CARTESIAN_POINT('',(0.517273426056,-39.7742356128,-7.80313755792));
#74819=CARTESIAN_POINT('Origin',(6.82290383517,-39.7742356128,-3.56061176027));
#74820=CARTESIAN_POINT('',(1.78291107349,-39.7742356128,-9.24906260055));
#74821=CARTESIAN_POINT('Origin',(6.82290383517,-39.7742356128,-3.56061176027));
#74822=CARTESIAN_POINT('',(2.42784894914,-39.7742356128,-9.76089341103));
#74823=CARTESIAN_POINT('Origin',(6.82290383517,-39.7742356128,-3.56061176027));
#74824=CARTESIAN_POINT('Origin',(6.82290383517,-39.7742356128,-3.56061176027));
#74825=CARTESIAN_POINT('Origin',(1.44328993201E-15,-40.7242356128,-7.34055663501));
#74826=CARTESIAN_POINT('',(-0.174946252184,-39.7742356128,-7.24363497156));
#74827=CARTESIAN_POINT('',(-0.174946252184,-40.7242356128,-7.24363497156));
#74828=CARTESIAN_POINT('Origin',(1.44328993201E-15,-39.7742356128,-7.34055663501));
#74829=CARTESIAN_POINT('Origin',(-6.82290383517,-40.1142356128,-3.56061176027));
#74830=CARTESIAN_POINT('',(-2.42784894914,-39.7742356128,-9.76089341103));
#74831=CARTESIAN_POINT('',(-14.4212065313,-39.7742356128,-3.4));
#74832=CARTESIAN_POINT('Origin',(-6.82290383517,-39.7742356128,-3.56061176027));
#74833=CARTESIAN_POINT('',(-1.78291107349,-39.7742356128,-9.24906260055));
#74834=CARTESIAN_POINT('Origin',(-6.82290383517,-39.7742356128,-3.56061176027));
#74835=CARTESIAN_POINT('',(-0.517273426056,-39.7742356128,-7.80313755792));
#74836=CARTESIAN_POINT('Origin',(-6.82290383517,-39.7742356128,-3.56061176027));
#74837=CARTESIAN_POINT('Origin',(-6.82290383517,-39.7742356128,-3.56061176027));
#74838=CARTESIAN_POINT('',(-14.4212065313,-40.7242356128,-3.4));
#74839=CARTESIAN_POINT('Origin',(-14.2514385284,-41.6742356128,-3.4));
#74840=CARTESIAN_POINT('',(-15.0199866844,-39.7742356128,-3.4));
#74841=CARTESIAN_POINT('',(-15.6610078691,-39.7742356128,-3.4));
#74842=CARTESIAN_POINT('',(-15.6610078691,-39.7742356128,-3.4));
#74843=CARTESIAN_POINT('Origin',(-7.34384247076,-41.6742356128,6.92091963994));
#74844=CARTESIAN_POINT('',(-7.34384247076,-39.7742356128,5.03150262895));
#74845=CARTESIAN_POINT('',(-7.34384247076,-40.7242356128,5.03150262895));
#74846=CARTESIAN_POINT('',(-7.34384247076,-39.7742356128,4.25491502787));
#74847=CARTESIAN_POINT('',(-7.34384247076,-39.7742356128,5.5634594739));
#74848=CARTESIAN_POINT('',(-7.34384247076,-39.7742356128,4.20599930786));
#74849=CARTESIAN_POINT('',(-7.34384247076,-39.7742356128,5.5634594739));
#74850=CARTESIAN_POINT('',(-7.34384247076,-40.7242356128,4.20599930786));
#74851=CARTESIAN_POINT('Origin',(-6.71477748978,-41.6742356128,4.80302787151));
#74852=CARTESIAN_POINT('',(-14.2293511975,-39.7742356128,7.53230140778));
#74853=CARTESIAN_POINT('',(-14.2293511975,-40.7242356128,7.53230140778));
#74854=CARTESIAN_POINT('',(-13.5647513306,-39.7742356128,7.2909204726));
#74855=CARTESIAN_POINT('',(-13.8970512641,-39.7742356128,7.41161094019));
#74856=CARTESIAN_POINT('',(-10.4542969007,-39.7742356128,6.16121155078));
#74857=CARTESIAN_POINT('Origin',(-3.5527136788E-15,-37.9242356128,-8.88178104417E-16));
#74858=CARTESIAN_POINT('',(-15.7368993134,-39.7742356128,3.4));
#74859=CARTESIAN_POINT('',(-15.7368993134,-40.7242356128,3.4));
#74860=CARTESIAN_POINT('Origin',(-3.5527136788E-15,-39.7742356128,-8.88178104417E-16));
#74861=CARTESIAN_POINT('Origin',(-16.2234398325,-41.6742356128,3.4));
#74862=CARTESIAN_POINT('',(-14.2514385284,-39.7742356128,3.4));
#74863=CARTESIAN_POINT('',(-14.2514385284,-40.4742356128,3.4));
#74864=CARTESIAN_POINT('',(-15.0199866844,-39.7742356128,3.4));
#74865=CARTESIAN_POINT('',(-15.6610078691,-39.7742356128,3.4));
#74866=CARTESIAN_POINT('',(-15.6610078691,-39.7742356128,3.4));
#74867=CARTESIAN_POINT('Origin',(-14.2514385284,-41.6742356128,2.4));
#74868=CARTESIAN_POINT('',(-14.2514385284,-39.7742356128,-1.95534782207));
#74869=CARTESIAN_POINT('',(-14.2514385284,-40.7242356128,-1.95534782207));
#74870=CARTESIAN_POINT('',(-14.2514385284,-39.7742356128,0.722326088964));
#74871=CARTESIAN_POINT('Origin',(-6.82290383517,-40.1142356128,-3.56061176027));
#74872=CARTESIAN_POINT('',(-7.52535686472,-39.7742356128,4.00685543432));
#74873=CARTESIAN_POINT('',(-7.52535686472,-40.7242356128,4.00685543432));
#74874=CARTESIAN_POINT('',(-9.78216646656,-39.7742356128,3.43958571397));
#74875=CARTESIAN_POINT('Origin',(-6.82290383517,-39.7742356128,-3.56061176027));
#74876=CARTESIAN_POINT('Origin',(-6.82290383517,-39.7742356128,-3.56061176027));
#74877=CARTESIAN_POINT('Origin',(-7.54384247076,-40.7242356128,4.20599930786));
#74878=CARTESIAN_POINT('Origin',(-7.54384247076,-39.7742356128,4.20599930786));
#74879=CARTESIAN_POINT('Origin',(7.54384247076,-40.7242356128,4.20599930786));
#74880=CARTESIAN_POINT('',(7.52535686472,-39.7742356128,4.00685543432));
#74881=CARTESIAN_POINT('',(7.52535686472,-40.7242356128,4.00685543432));
#74882=CARTESIAN_POINT('Origin',(7.54384247076,-39.7742356128,4.20599930786));
#74883=CARTESIAN_POINT('Origin',(6.82290383517,-40.1142356128,-3.56061176027));
#74884=CARTESIAN_POINT('Origin',(6.82290383517,-39.7742356128,-3.56061176027));
#74885=CARTESIAN_POINT('',(14.2514385284,-40.7242356128,-1.95534782207));
#74886=CARTESIAN_POINT('Origin',(14.2514385284,-41.6742356128,2.4));
#74887=CARTESIAN_POINT('',(14.2514385284,-40.7242356128,3.4));
#74888=CARTESIAN_POINT('Origin',(-16.2234398325,-41.6742356128,3.4));
#74889=CARTESIAN_POINT('Origin',(-0.000416107150126,-40.1142356128,6.92091963994));
#74890=CARTESIAN_POINT('',(-0.5,-39.7742356128,14.2473325884));
#74891=CARTESIAN_POINT('',(-0.5,-40.7242356128,14.2473325884));
#74892=CARTESIAN_POINT('',(-5.26789531411,-39.7742356128,12.0375174903));
#74893=CARTESIAN_POINT('Origin',(-0.000416107150126,-39.7742356128,6.92091963994));
#74894=CARTESIAN_POINT('',(-5.26789531411,-40.7242356128,12.0375174903));
#74895=CARTESIAN_POINT('Origin',(-0.5,-41.6742356128,13.1643460036));
#74896=CARTESIAN_POINT('',(-0.5,-39.7742356128,16.0922341519));
#74897=CARTESIAN_POINT('',(-0.5,-40.7242356128,16.0922341519));
#74898=CARTESIAN_POINT('',(-0.5,-39.7742356128,15.1697833702));
#74899=CARTESIAN_POINT('Origin',(-3.5527136788E-15,-37.9242356128,-8.88178104417E-16));
#74900=CARTESIAN_POINT('',(-13.7266446428,-39.7742356128,8.41363339168));
#74901=CARTESIAN_POINT('',(-13.7266446428,-40.7242356128,8.41363339168));
#74902=CARTESIAN_POINT('',(-2.7,-39.7742356128,15.8719879032));
#74903=CARTESIAN_POINT('Origin',(-3.5527136788E-15,-39.7742356128,-8.88178104417E-16));
#74904=CARTESIAN_POINT('Origin',(-3.5527136788E-15,-39.7742356128,-8.88178104417E-16));
#74905=CARTESIAN_POINT('Origin',(-6.37339887025,-41.6742356128,5.74295373993));
#74906=CARTESIAN_POINT('',(-7.34384247076,-39.7742356128,6.09541632002));
#74907=CARTESIAN_POINT('',(-7.34384247076,-40.7242356128,6.09541632002));
#74908=CARTESIAN_POINT('',(-13.0544719111,-39.7742356128,8.16950201179));
#74909=CARTESIAN_POINT('',(-10.1991571909,-39.7742356128,7.13245916591));
#74910=CARTESIAN_POINT('',(-13.390558277,-39.7742356128,8.29156770174));
#74911=CARTESIAN_POINT('Origin',(-7.34384247076,-41.6742356128,6.92091963994));
#74912=CARTESIAN_POINT('',(-7.34384247076,-39.7742356128,6.92091963994));
#74913=CARTESIAN_POINT('',(-7.34384247076,-40.7242356128,6.92091963994));
#74914=CARTESIAN_POINT('',(-7.34384247076,-39.7742356128,5.5634594739));
#74915=CARTESIAN_POINT('Origin',(-0.000416107150126,-40.1142356128,6.92091963994));
#74916=CARTESIAN_POINT('',(-6.88660115785,-39.7742356128,9.47167760676));
#74917=CARTESIAN_POINT('Origin',(-0.000416107150126,-39.7742356128,6.92091963994));
#74918=CARTESIAN_POINT('',(-6.88660115785,-40.7242356128,9.47167760676));
#74919=CARTESIAN_POINT('Origin',(-7.48272894647,-41.3342356129,11.6412701168));
#74920=CARTESIAN_POINT('',(-9.73272894647,-43.9742356128,11.6412701168));
#74921=CARTESIAN_POINT('Origin',(-7.48272894647,-43.9742356128,11.6412701168));
#74922=CARTESIAN_POINT('',(-9.73272894647,-39.7742356128,11.6412701168));
#74923=CARTESIAN_POINT('',(-9.73272894647,-41.3342356129,11.6412701168));
#74924=CARTESIAN_POINT('Origin',(-7.48272894647,-39.7742356128,11.6412701168));
#74925=CARTESIAN_POINT('',(-6.84013384355,-39.7742356128,13.7975566316));
#74926=CARTESIAN_POINT('Origin',(-7.48272894647,-39.7742356128,11.6412701168));
#74927=CARTESIAN_POINT('',(-9.71115043835,-39.7742356128,11.952136092));
#74928=CARTESIAN_POINT('Origin',(-7.48272894647,-39.7742356128,11.6412701168));
#74929=CARTESIAN_POINT('Origin',(-7.48272894647,-39.7742356128,11.6412701168));
#74930=CARTESIAN_POINT('Origin',(0.000416107150126,-40.1142356128,6.92091963994));
#74931=CARTESIAN_POINT('',(6.24384247076,-40.6742356128,6.92091963994));
#74932=CARTESIAN_POINT('',(6.24384247076,-40.1142356128,6.92091963994));
#74933=CARTESIAN_POINT('Origin',(0.000416107150126,-40.6742356128,6.92091963994));
#74934=CARTESIAN_POINT('Origin',(-6.24384247076,-41.6742356128,6.92091963994));
#74935=CARTESIAN_POINT('',(-6.24384247076,-40.6742356128,3.43894174696));
#74936=CARTESIAN_POINT('',(-6.24384247076,-41.1742356128,3.43894174696));
#74937=CARTESIAN_POINT('',(-6.24384247076,-40.6742356128,5.17993069345));
#74938=CARTESIAN_POINT('Origin',(-6.74384247076,-41.1742356128,3.43894174696));
#74939=CARTESIAN_POINT('',(-6.74948971107,-40.6742356128,2.9389736393));
#74940=CARTESIAN_POINT('Origin',(-6.74384247076,-40.6742356128,3.43894174696));
#74941=CARTESIAN_POINT('',(-6.74948971107,-41.1742356128,2.9389736393));
#74942=CARTESIAN_POINT('Origin',(-6.82290383517,-40.1142356128,-3.56061176027));
#74943=CARTESIAN_POINT('',(-0.4871654368,-40.6742356128,-5.0126513422));
#74944=CARTESIAN_POINT('Origin',(-6.82290383517,-40.6742356128,-3.56061176027));
#74945=CARTESIAN_POINT('',(-0.4871654368,-40.1142356128,-5.0126513422));
#74946=CARTESIAN_POINT('Origin',(0.000199055382222,-41.1742356128,-5.12434669465));
#74947=CARTESIAN_POINT('',(0.000199055298121561,-40.6742356128,-4.62434674748069));
#74948=CARTESIAN_POINT('Origin',(0.000199055382222,-40.6742356128,-5.12434669465));
#74949=CARTESIAN_POINT('',(0.000199055382222,-41.1742356128,-4.62434669465));
#74950=CARTESIAN_POINT('Origin',(-0.000199055382223,-41.1742356128,-5.12434669465));
#74951=CARTESIAN_POINT('',(0.4871654368,-40.6742356128,-5.0126513422));
#74952=CARTESIAN_POINT('Origin',(-0.000199055382223,-40.6742356128,-5.12434669465));
#74953=CARTESIAN_POINT('',(0.4871654368,-41.1742356128,-5.0126513422));
#74954=CARTESIAN_POINT('Origin',(6.82290383517,-40.1142356128,-3.56061176027));
#74955=CARTESIAN_POINT('',(6.74948971107,-40.6742356128,2.9389736393));
#74956=CARTESIAN_POINT('',(6.74948971107,-40.1142356128,2.9389736393));
#74957=CARTESIAN_POINT('Origin',(6.82290383517,-40.6742356128,-3.56061176027));
#74958=CARTESIAN_POINT('Origin',(6.74384247076,-41.1742356128,3.43894174696));
#74959=CARTESIAN_POINT('',(6.24384247076,-40.6742356128,3.43894174696));
#74960=CARTESIAN_POINT('Origin',(6.74384247076,-40.6742356128,3.43894174696));
#74961=CARTESIAN_POINT('',(6.24384247076,-41.1742356128,3.43894174696));
#74962=CARTESIAN_POINT('Origin',(6.24384247076,-41.6742356128,6.92091963994));
#74963=CARTESIAN_POINT('',(6.24384247076,-40.6742356128,5.17993069345));
#74964=CARTESIAN_POINT('Origin',(0.000416107150126,-40.1142356128,6.92091963994));
#74965=CARTESIAN_POINT('',(7.34384247076,-39.7742356128,6.92091963994));
#74966=CARTESIAN_POINT('',(7.34384247076,-40.7242356128,6.92091963994));
#74967=CARTESIAN_POINT('',(6.88660115785,-39.7742356128,9.47167760676));
#74968=CARTESIAN_POINT('Origin',(0.000416107150126,-39.7742356128,6.92091963994));
#74969=CARTESIAN_POINT('',(6.88660115785,-40.7242356128,9.47167760676));
#74970=CARTESIAN_POINT('Origin',(7.34384247076,-41.6742356128,6.92091963994));
#74971=CARTESIAN_POINT('',(7.34384247076,-39.7742356128,6.09541632002));
#74972=CARTESIAN_POINT('',(7.34384247076,-39.7742356128,5.5634594739));
#74973=CARTESIAN_POINT('',(7.34384247076,-40.7242356128,6.09541632002));
#74974=CARTESIAN_POINT('Origin',(6.52009030435,-41.6742356128,5.79623168551));
#74975=CARTESIAN_POINT('',(13.7266446428,-39.7742356128,8.41363339168));
#74976=CARTESIAN_POINT('',(13.7266446428,-40.7242356128,8.41363339168));
#74977=CARTESIAN_POINT('',(13.0544719111,-39.7742356128,8.16950201179));
#74978=CARTESIAN_POINT('',(13.390558277,-39.7742356128,8.29156770174));
#74979=CARTESIAN_POINT('',(10.1991571909,-39.7742356128,7.13245916591));
#74980=CARTESIAN_POINT('Origin',(-3.5527136788E-15,-37.9242356128,-8.88178104417E-16));
#74981=CARTESIAN_POINT('',(0.5,-39.7742356128,16.0922341519));
#74982=CARTESIAN_POINT('',(0.5,-40.7242356128,16.0922341519));
#74983=CARTESIAN_POINT('',(2.7,-39.7742356128,15.8719879032));
#74984=CARTESIAN_POINT('Origin',(-3.5527136788E-15,-39.7742356128,-8.88178104417E-16));
#74985=CARTESIAN_POINT('Origin',(-3.5527136788E-15,-39.7742356128,-8.88178104417E-16));
#74986=CARTESIAN_POINT('Origin',(0.5,-41.6742356128,13.1643460036));
#74987=CARTESIAN_POINT('',(0.5,-39.7742356128,14.2473325884));
#74988=CARTESIAN_POINT('',(0.5,-40.7242356128,14.2473325884));
#74989=CARTESIAN_POINT('',(0.5,-39.7742356128,15.1697833702));
#74990=CARTESIAN_POINT('Origin',(0.000416107150126,-40.1142356128,6.92091963994));
#74991=CARTESIAN_POINT('',(5.26789531411,-39.7742356128,12.0375174903));
#74992=CARTESIAN_POINT('Origin',(0.000416107150126,-39.7742356128,6.92091963994));
#74993=CARTESIAN_POINT('',(5.26789531411,-40.7242356128,12.0375174903));
#74994=CARTESIAN_POINT('Origin',(7.48272894647,-41.3342356129,11.6412701168));
#74995=CARTESIAN_POINT('',(9.71115043835,-39.7742356128,11.952136092));
#74996=CARTESIAN_POINT('',(9.73272894647,-39.7742356128,11.6412701168));
#74997=CARTESIAN_POINT('Origin',(7.48272894647,-39.7742356128,11.6412701168));
#74998=CARTESIAN_POINT('',(6.84013384355,-39.7742356128,13.7975566316));
#74999=CARTESIAN_POINT('Origin',(7.48272894647,-39.7742356128,11.6412701168));
#75000=CARTESIAN_POINT('Origin',(7.48272894647,-39.7742356128,11.6412701168));
#75001=CARTESIAN_POINT('Origin',(7.48272894647,-39.7742356128,11.6412701168));
#75002=CARTESIAN_POINT('',(9.73272894647,-43.9742356128,11.6412701168));
#75003=CARTESIAN_POINT('',(9.73272894647,-41.3342356129,11.6412701168));
#75004=CARTESIAN_POINT('',(5.23272894647,-43.9742356128,11.6412701168));
#75005=CARTESIAN_POINT('Origin',(7.48272894647,-43.9742356128,11.6412701168));
#75006=CARTESIAN_POINT('Origin',(7.48272894647,-43.9742356128,11.6412701168));
#75007=CARTESIAN_POINT('Origin',(-3.35265884719E-30,-39.7742356128,3.15283103411E-22));
#75008=CARTESIAN_POINT('Origin',(-3.35265884719E-30,-39.2742356128,3.15283103411E-22));
#75009=CARTESIAN_POINT('',(-3.7,-39.2742356128,0.));
#75010=CARTESIAN_POINT('Origin',(-3.7,-34.1742356128,16.9339894886));
#75011=CARTESIAN_POINT('',(-3.7,-35.1742356128,15.977171214));
#75012=CARTESIAN_POINT('',(-3.7,-35.1742356128,16.4899553024));
#75013=CARTESIAN_POINT('',(-3.7,-37.2242356128,15.977171214));
#75014=CARTESIAN_POINT('Origin',(-14.2514385284,-38.7742356128,2.4));
#75015=CARTESIAN_POINT('',(-14.2514385284,-33.4742356128,2.4));
#75016=CARTESIAN_POINT('',(-14.2514385284,-38.7742356128,2.4));
#75017=CARTESIAN_POINT('',(-14.2514385284,-36.1242356128,2.4));
#75018=CARTESIAN_POINT('',(-16.5266451526,-33.4742356128,2.4));
#75019=CARTESIAN_POINT('',(-15.3890418405,-33.4742356128,2.4));
#75020=CARTESIAN_POINT('',(-16.5266451526,-34.4742356128,2.4));
#75021=CARTESIAN_POINT('',(-16.5266451526,-33.9742356128,2.4));
#75022=CARTESIAN_POINT('',(-16.3750424925,-34.4742356128,2.4));
#75023=CARTESIAN_POINT('',(-15.2118374958,-37.2742356128,2.4));
#75024=CARTESIAN_POINT('',(-15.7176386641,-37.2742356128,2.4));
#75025=CARTESIAN_POINT('',(-15.2118374958,-38.7742356128,2.4));
#75026=CARTESIAN_POINT('',(-15.2118374958,-38.0242356128,2.4));
#75027=CARTESIAN_POINT('',(-14.7316380121,-38.7742356128,2.4));
#75028=CARTESIAN_POINT('Origin',(-3.35265884719E-30,-34.4742356128,3.15283103411E-22));
#75029=CARTESIAN_POINT('',(-16.5266451526,-34.4742356128,-2.4));
#75030=CARTESIAN_POINT('Origin',(6.66133814775094E-15,-34.4742356128,3.71924713249427E-14));
#75031=CARTESIAN_POINT('',(-15.8187195902,-34.4742356128,-2.4));
#75032=CARTESIAN_POINT('Origin',(-14.2514385284,-38.7742356128,-2.4));
#75033=CARTESIAN_POINT('',(-14.2514385284,-38.7742356128,-2.4));
#75034=CARTESIAN_POINT('',(-15.2118374958,-38.7742356128,-2.4));
#75035=CARTESIAN_POINT('',(-14.7316380121,-38.7742356128,-2.4));
#75036=CARTESIAN_POINT('',(-15.2118374958,-37.2742356128,-2.4));
#75037=CARTESIAN_POINT('',(-15.2118374958,-38.0242356128,-2.4));
#75038=CARTESIAN_POINT('',(-15.7176386641,-37.2742356128,-2.4));
#75039=CARTESIAN_POINT('',(-16.5266451526,-33.4742356128,-2.4));
#75040=CARTESIAN_POINT('',(-16.5266451526,-33.9742356128,-2.4));
#75041=CARTESIAN_POINT('',(-14.2514385284,-33.4742356128,-2.4));
#75042=CARTESIAN_POINT('',(-15.3890418405,-33.4742356128,-2.4));
#75043=CARTESIAN_POINT('',(-14.2514385284,-36.1242356128,-2.4));
#75044=CARTESIAN_POINT('Origin',(-4.7,-34.1742356128,-14.1421356237));
#75045=CARTESIAN_POINT('',(-4.7,-35.1742356128,-15.7120972502));
#75046=CARTESIAN_POINT('',(-4.7,-35.1742356128,-16.2330883256));
#75047=CARTESIAN_POINT('',(-4.7,-39.2742356128,-16.2330883256));
#75048=CARTESIAN_POINT('',(-4.7,-37.2242356128,-15.7120972502));
#75049=CARTESIAN_POINT('Origin',(-3.35265884719E-30,-39.2742356128,3.15283103411E-22));
#75050=CARTESIAN_POINT('Origin',(-3.35265884719E-30,-39.2742356128,3.15283103411E-22));
#75051=CARTESIAN_POINT('',(3.7,-39.2742356128,0.));
#75052=CARTESIAN_POINT('Origin',(3.7,-34.1742356128,16.9339894886));
#75053=CARTESIAN_POINT('',(3.7,-35.1742356128,15.977171214));
#75054=CARTESIAN_POINT('',(3.7,-37.2242356128,15.977171214));
#75055=CARTESIAN_POINT('',(3.7,-35.1742356128,16.4899553024));
#75056=CARTESIAN_POINT('Origin',(-3.35265884719E-30,-39.2742356128,3.15283103411E-22));
#75057=CARTESIAN_POINT('',(4.7,-39.2742356128,0.));
#75058=CARTESIAN_POINT('Origin',(4.7,-34.1742356128,-14.1421356237));
#75059=CARTESIAN_POINT('',(4.7,-35.1742356128,-15.7120972502));
#75060=CARTESIAN_POINT('',(4.7,-37.2242356128,-15.7120972502));
#75061=CARTESIAN_POINT('',(4.7,-35.1742356128,-16.2330883256));
#75062=CARTESIAN_POINT('Origin',(-14.2514385284,-38.7742356128,-2.4));
#75063=CARTESIAN_POINT('',(15.2118374958,-37.2742356128,-2.4));
#75064=CARTESIAN_POINT('',(15.7176386641,-37.2742356128,-2.4));
#75065=CARTESIAN_POINT('',(15.2118374958,-38.7742356128,-2.4));
#75066=CARTESIAN_POINT('',(15.2118374958,-38.0242356128,-2.4));
#75067=CARTESIAN_POINT('',(14.2514385284,-38.7742356128,-2.4));
#75068=CARTESIAN_POINT('',(14.7316380121,-38.7742356128,-2.4));
#75069=CARTESIAN_POINT('',(14.2514385284,-33.4742356128,-2.4));
#75070=CARTESIAN_POINT('',(14.2514385284,-36.1242356128,-2.4));
#75071=CARTESIAN_POINT('',(16.5266451526,-33.4742356128,-2.4));
#75072=CARTESIAN_POINT('',(15.3890418405,-33.4742356128,-2.4));
#75073=CARTESIAN_POINT('',(16.5266451526,-34.4742356128,-2.4));
#75074=CARTESIAN_POINT('',(16.5266451526,-33.9742356128,-2.4));
#75075=CARTESIAN_POINT('',(16.3750424925,-34.4742356128,-2.4));
#75076=CARTESIAN_POINT('Origin',(-3.35265884719E-30,-34.4742356128,3.15283103411E-22));
#75077=CARTESIAN_POINT('',(16.5266451526,-34.4742356128,2.4));
#75078=CARTESIAN_POINT('Origin',(-6.66133814775094E-15,-34.4742356128004,
3.71924713249427E-14));
#75079=CARTESIAN_POINT('',(-15.8187195902,-34.4742356128,2.4));
#75080=CARTESIAN_POINT('Origin',(-14.2514385284,-38.7742356128,2.4));
#75081=CARTESIAN_POINT('',(16.5266451526,-33.4742356128,2.4));
#75082=CARTESIAN_POINT('',(16.5266451526,-33.9742356128,2.4));
#75083=CARTESIAN_POINT('',(14.2514385284,-33.4742356128,2.4));
#75084=CARTESIAN_POINT('',(15.3890418405,-33.4742356128,2.4));
#75085=CARTESIAN_POINT('',(14.2514385284,-38.7742356128,2.4));
#75086=CARTESIAN_POINT('',(14.2514385284,-36.1242356128,2.4));
#75087=CARTESIAN_POINT('',(15.2118374958,-38.7742356128,2.4));
#75088=CARTESIAN_POINT('',(14.7316380121,-38.7742356128,2.4));
#75089=CARTESIAN_POINT('',(15.2118374958,-37.2742356128,2.4));
#75090=CARTESIAN_POINT('',(15.2118374958,-38.0242356128,2.4));
#75091=CARTESIAN_POINT('',(15.7176386641,-37.2742356128,2.4));
#75092=CARTESIAN_POINT('Origin',(-3.35265884719E-30,-34.4742356128,3.15283103411E-22));
#75093=CARTESIAN_POINT('',(4.,-34.4742356128,-15.9047162817));
#75094=CARTESIAN_POINT('',(4.,-34.4742356128,0.));
#75095=CARTESIAN_POINT('',(-4.,-34.4742356128,-15.9047162817));
#75096=CARTESIAN_POINT('',(-4.,-34.4742356128,0.));
#75097=CARTESIAN_POINT('Origin',(1.09356967925578E-13,-34.4742356128,9.10382880192628E-14));
#75098=CARTESIAN_POINT('Origin',(4.,-35.1742356128,-16.5096094651));
#75099=CARTESIAN_POINT('Ctrl Pts',(4.,-34.4742356128,-15.9047162816568));
#75100=CARTESIAN_POINT('Ctrl Pts',(4.0884342264605,-34.4742356127987,-15.8824752746765));
#75101=CARTESIAN_POINT('Ctrl Pts',(4.18270996429947,-34.4919847748025,-15.8579009499871));
#75102=CARTESIAN_POINT('Ctrl Pts',(4.35634416466974,-34.5644258306867,-15.8110831603776));
#75103=CARTESIAN_POINT('Ctrl Pts',(4.43571134875728,-34.6191227440986,-15.7888798171352));
#75104=CARTESIAN_POINT('Ctrl Pts',(4.55893320645631,-34.7441108613033,-15.7537322365075));
#75105=CARTESIAN_POINT('Ctrl Pts',(4.61190458227807,-34.821900720567,-15.738223817141));
#75106=CARTESIAN_POINT('Ctrl Pts',(4.68245030316865,-34.9930487805266,-15.7173792968254));
#75107=CARTESIAN_POINT('Ctrl Pts',(4.7,-35.0864237188467,-15.7120972502082));
#75108=CARTESIAN_POINT('Ctrl Pts',(4.7,-35.1742356128,-15.7120972502082));
#75109=CARTESIAN_POINT('Origin',(-4.,-35.1742356128,-16.5096094651));
#75110=CARTESIAN_POINT('Ctrl Pts',(-4.,-34.4742356128,-15.9047162816568));
#75111=CARTESIAN_POINT('Ctrl Pts',(-4.0884342264605,-34.4742356127987,-15.8824752746765));
#75112=CARTESIAN_POINT('Ctrl Pts',(-4.18270996429947,-34.4919847748025,
-15.8579009499871));
#75113=CARTESIAN_POINT('Ctrl Pts',(-4.35634416466974,-34.5644258306867,
-15.8110831603776));
#75114=CARTESIAN_POINT('Ctrl Pts',(-4.43571134875728,-34.6191227440986,
-15.7888798171352));
#75115=CARTESIAN_POINT('Ctrl Pts',(-4.55893320645631,-34.7441108613033,
-15.7537322365075));
#75116=CARTESIAN_POINT('Ctrl Pts',(-4.61190458227807,-34.821900720567,-15.738223817141));
#75117=CARTESIAN_POINT('Ctrl Pts',(-4.68245030316865,-34.9930487805266,
-15.7173792968254));
#75118=CARTESIAN_POINT('Ctrl Pts',(-4.7,-35.0864237188467,-15.7120972502082));
#75119=CARTESIAN_POINT('Ctrl Pts',(-4.7,-35.1742356128,-15.7120972502082));
#75120=CARTESIAN_POINT('Origin',(-3.35265884719E-30,-39.7742356128,3.15283103411E-22));
#75121=CARTESIAN_POINT('',(-3.7,-39.7742356128,-14.9489130039));
#75122=CARTESIAN_POINT('',(-3.7,-39.7742356128,0.0995229481798));
#75123=CARTESIAN_POINT('Ctrl Pts',(-3.7,-39.7742356128,-14.9489130039));
#75124=CARTESIAN_POINT('Ctrl Pts',(-7.0053528771,-39.7742356128,-14.13080632));
#75125=CARTESIAN_POINT('Ctrl Pts',(-10.0851737187,-39.7742356128,-12.3997944898));
#75126=CARTESIAN_POINT('Ctrl Pts',(-12.5992021916,-39.7742356128,-9.8349243241));
#75127=CARTESIAN_POINT('Ctrl Pts',(-14.2682129749,-39.7742356128,-6.72106797252));
#75128=CARTESIAN_POINT('Ctrl Pts',(-15.0199866844,-39.7742356128,-3.4));
#75129=CARTESIAN_POINT('Origin',(-3.35265884719E-30,-39.7742356128,3.15283103411E-22));
#75130=CARTESIAN_POINT('',(1.34531962036,-39.7742356128,-9.93626746742));
#75131=CARTESIAN_POINT('Ctrl Pts',(1.34531962036,-39.7742356128,-9.93626746742));
#75132=CARTESIAN_POINT('Ctrl Pts',(1.61677669863,-39.7742356128,-9.89864634179));
#75133=CARTESIAN_POINT('Ctrl Pts',(1.86584893824,-39.7742356128,-9.86245065748));
#75134=CARTESIAN_POINT('Ctrl Pts',(2.0496779846,-39.7742356128,-9.83314926899));
#75135=CARTESIAN_POINT('Ctrl Pts',(2.23813956402,-39.7742356128,-9.79905599631));
#75136=CARTESIAN_POINT('Ctrl Pts',(2.42784894914,-39.7742356128,-9.76089341103));
#75137=CARTESIAN_POINT('',(-1.34531962036,-39.7742356128,-9.93626746742));
#75138=CARTESIAN_POINT('Origin',(-1.99840144432528E-14,-39.7742356128,-2.6737364819903));
#75139=CARTESIAN_POINT('Ctrl Pts',(-1.34531962036,-39.7742356128,-9.93626746742));
#75140=CARTESIAN_POINT('Ctrl Pts',(-1.61677669863,-39.7742356128,-9.89864634179));
#75141=CARTESIAN_POINT('Ctrl Pts',(-1.86584893824,-39.7742356128,-9.86245065748));
#75142=CARTESIAN_POINT('Ctrl Pts',(-2.0496779846,-39.7742356128,-9.83314926899));
#75143=CARTESIAN_POINT('Ctrl Pts',(-2.23813956402,-39.7742356128,-9.79905599631));
#75144=CARTESIAN_POINT('Ctrl Pts',(-2.42784894914,-39.7742356128,-9.76089341103));
#75145=CARTESIAN_POINT('',(3.7,-39.7742356128,-14.9489130039));
#75146=CARTESIAN_POINT('',(3.7,-39.7742356128,0.717649133781));
#75147=CARTESIAN_POINT('Ctrl Pts',(15.0199866844,-39.7742356128,-3.4));
#75148=CARTESIAN_POINT('Ctrl Pts',(14.2682129749,-39.7742356128,-6.72106797252));
#75149=CARTESIAN_POINT('Ctrl Pts',(12.5992021916,-39.7742356128,-9.8349243241));
#75150=CARTESIAN_POINT('Ctrl Pts',(10.0851737187,-39.7742356128,-12.3997944898));
#75151=CARTESIAN_POINT('Ctrl Pts',(7.0053528771,-39.7742356128,-14.13080632));
#75152=CARTESIAN_POINT('Ctrl Pts',(3.7,-39.7742356128,-14.9489130039));
#75153=CARTESIAN_POINT('Origin',(-3.35265884719E-30,-39.7742356128,3.15283103411E-22));
#75154=CARTESIAN_POINT('Origin',(-3.35265884719E-30,-39.7742356128,3.15283103411E-22));
#75155=CARTESIAN_POINT('',(0.517273426056,-39.7742356128,-7.9495168227));
#75156=CARTESIAN_POINT('Ctrl Pts',(1.78291107349,-39.7742356128,-9.24906260055));
#75157=CARTESIAN_POINT('Ctrl Pts',(1.28116922679,-39.7742356128,-9.2357956341));
#75158=CARTESIAN_POINT('Ctrl Pts',(0.780312185558,-39.7742356128,-8.95942136571));
#75159=CARTESIAN_POINT('Ctrl Pts',(0.517273426057,-39.7742356128,-8.45143404011));
#75160=CARTESIAN_POINT('Ctrl Pts',(0.517273426056,-39.7742356128,-7.9495168227));
#75161=CARTESIAN_POINT('',(0.517273426056,-39.7742356128,0.717649133781));
#75162=CARTESIAN_POINT('',(-0.517273426056,-39.7742356128,-7.9495168227));
#75163=CARTESIAN_POINT('',(-0.517273426056,-39.7742356128,0.717649133781));
#75164=CARTESIAN_POINT('Ctrl Pts',(-0.517273426056,-39.7742356128,-7.9495168227));
#75165=CARTESIAN_POINT('Ctrl Pts',(-0.517273426057,-39.7742356128,-8.45143404011));
#75166=CARTESIAN_POINT('Ctrl Pts',(-0.780312185558,-39.7742356128,-8.95942136571));
#75167=CARTESIAN_POINT('Ctrl Pts',(-1.28116922679,-39.7742356128,-9.2357956341));
#75168=CARTESIAN_POINT('Ctrl Pts',(-1.78291107349,-39.7742356128,-9.24906260055));
#75169=CARTESIAN_POINT('Origin',(-3.35265884719E-30,-39.7742356128,3.15283103411E-22));
#75170=CARTESIAN_POINT('Origin',(-3.35265884719E-30,-39.7742356128,3.15283103411E-22));
#75171=CARTESIAN_POINT('Origin',(-3.35265884719E-30,-39.7742356128,3.15283103411E-22));
#75172=CARTESIAN_POINT('',(-7.4311653291,-39.7742356128,4.27488229452));
#75173=CARTESIAN_POINT('Ctrl Pts',(-9.78216646656,-39.7742356128,3.43958571397));
#75174=CARTESIAN_POINT('Ctrl Pts',(-9.44950651023,-39.7742356128,3.84219609922));
#75175=CARTESIAN_POINT('Ctrl Pts',(-9.03618230028,-39.7742356128,4.19379483572));
#75176=CARTESIAN_POINT('Ctrl Pts',(-8.49317585372,-39.7742356128,4.40265075658));
#75177=CARTESIAN_POINT('Ctrl Pts',(-7.94364631071,-39.7742356128,4.41424876979));
#75178=CARTESIAN_POINT('Ctrl Pts',(-7.4311653291,-39.7742356128,4.27488229452));
#75179=CARTESIAN_POINT('Origin',(-7.20379737374474,-39.7742356128,5.06830226500522));
#75180=CARTESIAN_POINT('Origin',(-3.35265884719E-30,-39.7742356128,3.15283103411E-22));
#75181=CARTESIAN_POINT('Origin',(-3.59850171520844,-39.7742356128,1.3458683859997));
#75182=CARTESIAN_POINT('Origin',(-3.35265884719E-30,-39.7742356128,3.15283103411E-22));
#75183=CARTESIAN_POINT('Origin',(-3.35265884719E-30,-39.7742356128,3.15283103411E-22));
#75184=CARTESIAN_POINT('',(-2.7,-39.7742356128,15.1614643092));
#75185=CARTESIAN_POINT('',(-2.7,-39.7742356128,0.717649133781));
#75186=CARTESIAN_POINT('Origin',(-1.20186252263148,-39.7742356128,3.64824670717903));
#75187=CARTESIAN_POINT('Origin',(-3.35265884719E-30,-39.7742356128,3.15283103411E-22));
#75188=CARTESIAN_POINT('Origin',(-2.87571670214971,-39.7742356128,2.54173286620876));
#75189=CARTESIAN_POINT('Origin',(-3.35265884719E-30,-39.7742356128,3.15283103411E-22));
#75190=CARTESIAN_POINT('Origin',(-7.48272894647,-43.9742356128,11.6412701168));
#75191=CARTESIAN_POINT('',(-9.23272894647,-44.4742356128,11.6412701168));
#75192=CARTESIAN_POINT('Origin',(-9.23272894647,-43.9742356128,11.6412701168));
#75193=CARTESIAN_POINT('Origin',(-7.48272894647,-44.4742356128,11.6412701168));
#75194=CARTESIAN_POINT('Origin',(-3.35265884719E-30,-40.6742356128,3.15283103411E-22));
#75195=CARTESIAN_POINT('',(4.89234685393,-40.6742356128,2.64607413014));
#75196=CARTESIAN_POINT('',(5.24384247076,-40.6742356128,3.12351150632));
#75197=CARTESIAN_POINT('Origin',(4.74384247076,-40.6742356128,3.12351150632));
#75198=CARTESIAN_POINT('',(0.48735027394,-40.6742356128,-2.10776590718));
#75199=CARTESIAN_POINT('Origin',(6.82290383517,-40.6742356128,-3.56061176027));
#75200=CARTESIAN_POINT('',(-0.48735027394,-40.6742356128,-2.10776590718));
#75201=CARTESIAN_POINT('Origin',(-4.99600361081E-16,-40.6742356128,-1.99600853387));
#75202=CARTESIAN_POINT('',(-4.89234685393,-40.6742356128,2.64607413014));
#75203=CARTESIAN_POINT('Origin',(-6.82290383517,-40.6742356128,-3.56061176027));
#75204=CARTESIAN_POINT('',(-5.24384247076,-40.6742356128,3.12351150632));
#75205=CARTESIAN_POINT('Origin',(-4.74384247076,-40.6742356128,3.12351150632));
#75206=CARTESIAN_POINT('',(-5.24384247076,-40.6742356128,6.92091963994));
#75207=CARTESIAN_POINT('',(-5.24384247076,-40.6742356128,5.02221557313));
#75208=CARTESIAN_POINT('',(-0.000416107143134986,-40.6742356128,12.1643459815524));
#75209=CARTESIAN_POINT('Origin',(-0.000416107150126,-40.6742356128,6.92091963994));
#75210=CARTESIAN_POINT('',(5.24384247076,-40.6742356128,6.92091963994));
#75211=CARTESIAN_POINT('Origin',(0.000416107150126,-40.6742356128,6.92091963994));
#75212=CARTESIAN_POINT('',(5.24384247076,-40.6742356128,5.02221557313));
#75213=CARTESIAN_POINT('',(12.3229038352,-40.6742356128,-3.56061176027));
#75214=CARTESIAN_POINT('Origin',(6.82290383517,-40.6742356128,-3.56061176027));
#75215=CARTESIAN_POINT('',(-12.3229038352,-40.6742356128,-3.56061176027));
#75216=CARTESIAN_POINT('Origin',(-6.82290383517,-40.6742356128,-3.56061176027));
#75217=CARTESIAN_POINT('Origin',(-3.35265884719E-30,-39.7742356128,3.15283103411E-22));
#75218=CARTESIAN_POINT('Origin',(2.87571670201055,-39.7742356128,2.54173286608641));
#75219=CARTESIAN_POINT('Origin',(-3.35265884719E-30,-39.7742356128,3.15283103411E-22));
#75220=CARTESIAN_POINT('',(2.7,-39.7742356128,15.1614643092));
#75221=CARTESIAN_POINT('',(2.7,-39.7742356128,0.0995229481798));
#75222=CARTESIAN_POINT('Origin',(1.20186252262849,-39.7742356128,3.64824670717053));
#75223=CARTESIAN_POINT('Origin',(-3.35265884719E-30,-39.7742356128,3.15283103411E-22));
#75224=CARTESIAN_POINT('Origin',(7.48272894647,-43.9742356128,11.6412701168));
#75225=CARTESIAN_POINT('',(5.73272894647,-44.4742356128,11.6412701168));
#75226=CARTESIAN_POINT('Origin',(5.73272894647,-43.9742356128,11.6412701168));
#75227=CARTESIAN_POINT('Origin',(7.48272894647,-44.4742356128,11.6412701168));
#75228=CARTESIAN_POINT('Origin',(-3.,-35.1742356128,16.6523581407));
#75229=CARTESIAN_POINT('',(-3.,-34.4742356128,16.1232751015));
#75230=CARTESIAN_POINT('',(-3.,-34.4742356128,16.5582997212));
#75231=CARTESIAN_POINT('Ctrl Pts',(-3.,-34.4742356128,16.1232751015419));
#75232=CARTESIAN_POINT('Ctrl Pts',(-3.08826358006266,-34.474235612801,16.1068522136037));
#75233=CARTESIAN_POINT('Ctrl Pts',(-3.182339037103,-34.491928240058,16.0885214326175));
#75234=CARTESIAN_POINT('Ctrl Pts',(-3.35547017666015,-34.5639636844578,
16.0533056885098));
#75235=CARTESIAN_POINT('Ctrl Pts',(-3.43453320463452,-34.618308389591,16.03646071159));
#75236=CARTESIAN_POINT('Ctrl Pts',(-3.55816883888233,-34.7429717428544,
16.0094769404987));
#75237=CARTESIAN_POINT('Ctrl Pts',(-3.61151559883288,-34.8211404463089,
15.9974459840977));
#75238=CARTESIAN_POINT('Ctrl Pts',(-3.68243855940585,-34.9928379015306,
15.9812693237053));
#75239=CARTESIAN_POINT('Ctrl Pts',(-3.7,-35.0863772305776,15.977171213954));
#75240=CARTESIAN_POINT('Ctrl Pts',(-3.7,-35.1742356128,15.977171213954));
#75241=CARTESIAN_POINT('Origin',(-3.5527136788E-15,-37.9242356128,-8.88178104417E-16));
#75242=CARTESIAN_POINT('',(3.,-34.4742356128,16.1232751015));
#75243=CARTESIAN_POINT('Origin',(-3.5527136788E-15,-34.4742356128,-8.88178104417E-16));
#75244=CARTESIAN_POINT('Ctrl Pts',(3.7,-35.1742356128,15.977171213954));
#75245=CARTESIAN_POINT('Ctrl Pts',(3.7,-35.0863772305776,15.977171213954));
#75246=CARTESIAN_POINT('Ctrl Pts',(3.68243855940585,-34.9928379015306,15.9812693237053));
#75247=CARTESIAN_POINT('Ctrl Pts',(3.61151559883287,-34.8211404463089,15.9974459840977));
#75248=CARTESIAN_POINT('Ctrl Pts',(3.55816883888233,-34.7429717428544,16.0094769404987));
#75249=CARTESIAN_POINT('Ctrl Pts',(3.43453320463452,-34.618308389591,16.03646071159));
#75250=CARTESIAN_POINT('Ctrl Pts',(3.35547017666015,-34.5639636844578,16.0533056885098));
#75251=CARTESIAN_POINT('Ctrl Pts',(3.182339037103,-34.491928240058,16.0885214326175));
#75252=CARTESIAN_POINT('Ctrl Pts',(3.08826358006266,-34.4742356128,16.1068522136038));
#75253=CARTESIAN_POINT('Ctrl Pts',(3.,-34.4742356128,16.1232751015419));
#75254=CARTESIAN_POINT('Origin',(-3.5527136788E-15,-37.2742356128,-8.88178104417E-16));
#75255=CARTESIAN_POINT('Origin',(-3.35265884719E-30,-38.2742356128,3.15283103411E-22));
#75256=CARTESIAN_POINT('',(-12.8848511691,-38.7742356128,8.43448933535));
#75257=CARTESIAN_POINT('',(-12.8848511691,-37.2742356128,8.43448933535));
#75258=CARTESIAN_POINT('',(-12.8848511691,-38.2742356128,8.43448933535));
#75259=CARTESIAN_POINT('Origin',(-3.35265884719E-30,-38.7742356128,3.15283103411E-22));
#75260=CARTESIAN_POINT('Origin',(-3.35265884719E-30,-37.2742356128,3.15283103411E-22));
#75261=CARTESIAN_POINT('Origin',(-3.35265884719E-30,-36.1242356128,3.15283103411E-22));
#75262=CARTESIAN_POINT('',(-9.94046468191,-38.7742356128,11.7621070351));
#75263=CARTESIAN_POINT('',(-12.1387953782,-38.7742356128,9.47679517369));
#75264=CARTESIAN_POINT('Origin',(-3.35265884719E-30,-38.7742356128,3.15283103411E-22));
#75265=CARTESIAN_POINT('',(-12.1387953782,-33.7742356128,9.47679517369));
#75266=CARTESIAN_POINT('',(-12.1387953782,-36.1242356128,9.47679517369));
#75267=CARTESIAN_POINT('',(-9.94046468191,-33.7742356128,11.7621070351));
#75268=CARTESIAN_POINT('Origin',(-3.35265884719E-30,-33.7742356128,3.15283103411E-22));
#75269=CARTESIAN_POINT('',(-9.94046468191,-36.1242356128,11.7621070351));
#75270=CARTESIAN_POINT('Origin',(-3.35265884719E-30,-38.2742356128,3.15283103411E-22));
#75271=CARTESIAN_POINT('',(-8.92662908173,-38.7742356128,12.5489160184));
#75272=CARTESIAN_POINT('',(-8.92662908173,-37.2742356128,12.5489160184));
#75273=CARTESIAN_POINT('',(-8.92662908173,-38.2742356128,12.5489160184));
#75274=CARTESIAN_POINT('',(-0.5,-37.2742356128,15.3918809766));
#75275=CARTESIAN_POINT('Origin',(-3.35265884719E-30,-37.2742356128,3.15283103411E-22));
#75276=CARTESIAN_POINT('',(-0.5,-38.7742356128,15.3918809766));
#75277=CARTESIAN_POINT('',(-0.5,-38.2742356128,15.3918809766));
#75278=CARTESIAN_POINT('Origin',(-3.35265884719E-30,-38.7742356128,3.15283103411E-22));
#75279=CARTESIAN_POINT('Origin',(-3.35265884719E-30,-38.2742356128,3.15283103411E-22));
#75280=CARTESIAN_POINT('',(9.33467257157,-38.7742356128,12.2484238978));
#75281=CARTESIAN_POINT('',(9.33467257157,-37.2742356128,12.2484238978));
#75282=CARTESIAN_POINT('',(9.33467257157,-38.2742356128,12.2484238978));
#75283=CARTESIAN_POINT('',(0.5,-38.7742356128,15.3918809766));
#75284=CARTESIAN_POINT('Origin',(-3.35265884719E-30,-38.7742356128,3.15283103411E-22));
#75285=CARTESIAN_POINT('',(0.5,-37.2742356128,15.3918809766));
#75286=CARTESIAN_POINT('',(0.5,-38.2742356128,15.3918809766));
#75287=CARTESIAN_POINT('Origin',(-3.35265884719E-30,-37.2742356128,3.15283103411E-22));
#75288=CARTESIAN_POINT('Origin',(-3.35265884719E-30,-36.1242356128,3.15283103411E-22));
#75289=CARTESIAN_POINT('',(11.816958431,-38.7742356128,9.87519586841));
#75290=CARTESIAN_POINT('',(10.3256459325,-38.7742356128,11.4254556179));
#75291=CARTESIAN_POINT('Origin',(-3.35265884719E-30,-38.7742356128,3.15283103411E-22));
#75292=CARTESIAN_POINT('',(10.3256459325,-33.7742356128,11.4254556179));
#75293=CARTESIAN_POINT('',(10.3256459325,-36.1242356128,11.4254556179));
#75294=CARTESIAN_POINT('',(11.816958431,-33.7742356128,9.87519586841));
#75295=CARTESIAN_POINT('Origin',(-3.35265884719E-30,-33.7742356128,3.15283103411E-22));
#75296=CARTESIAN_POINT('',(11.816958431,-36.1242356128,9.87519586841));
#75297=CARTESIAN_POINT('Origin',(-3.35265884719E-30,-38.2742356128,3.15283103411E-22));
#75298=CARTESIAN_POINT('',(12.5997104365,-38.7742356128,8.85478949011));
#75299=CARTESIAN_POINT('',(12.5997104365,-37.2742356128,8.85478949011));
#75300=CARTESIAN_POINT('',(12.5997104365,-38.2742356128,8.85478949011));
#75301=CARTESIAN_POINT('Origin',(-3.35265884719E-30,-37.2742356128,3.15283103411E-22));
#75302=CARTESIAN_POINT('Origin',(-3.35265884719E-30,-38.7742356128,3.15283103411E-22));
#75303=CARTESIAN_POINT('Origin',(-14.2514385284,-41.6742356128,2.4));
#75304=CARTESIAN_POINT('',(-14.2514385284,-33.4742356128,0.));
#75305=CARTESIAN_POINT('',(-14.2514385284,-38.7742356128,0.));
#75306=CARTESIAN_POINT('Origin',(-3.35265884719E-30,-33.4742356128,3.15283103411E-22));
#75307=CARTESIAN_POINT('Origin',(-3.35265884719E-30,-33.4742356128,3.15283103411E-22));
#75308=CARTESIAN_POINT('Origin',(-3.35265884719E-30,-38.1842356129,3.15283103411E-22));
#75309=CARTESIAN_POINT('Origin',(-3.35265884719E-30,-38.7742356128,3.15283103411E-22));
#75310=CARTESIAN_POINT('',(-9.33467257157,-38.7742356128,-12.2484238978));
#75311=CARTESIAN_POINT('',(-6.35435667676,-38.7742356128,-9.34315312398));
#75312=CARTESIAN_POINT('',(-9.33467257157,-38.7742356128,-12.2484238978));
#75313=CARTESIAN_POINT('',(-1.48259713265,-38.7742356128,-10.9268000942));
#75314=CARTESIAN_POINT('Ctrl Pts',(-1.48259713264981,-38.7742356128,-10.9268000941986));
#75315=CARTESIAN_POINT('Ctrl Pts',(-1.71328083841,-38.7742356128,-10.8948297336));
#75316=CARTESIAN_POINT('Ctrl Pts',(-1.91354623838,-38.7742356128,-10.8659465412));
#75317=CARTESIAN_POINT('Ctrl Pts',(-2.0855726443,-38.7742356128,-10.8395401686));
#75318=CARTESIAN_POINT('Ctrl Pts',(-3.07854611663017,-38.7742356128,-10.6733698534772));
#75319=CARTESIAN_POINT('Ctrl Pts',(-4.05813867421687,-38.7742356128,-10.4126758711406));
#75320=CARTESIAN_POINT('Ctrl Pts',(-4.86043811085114,-38.7742356128,-10.1190200263027));
#75321=CARTESIAN_POINT('Ctrl Pts',(-5.62475805695127,-38.7742356128,-9.76080244433856));
#75322=CARTESIAN_POINT('Ctrl Pts',(-6.35435667676406,-38.7742356128,-9.34315312398709));
#75323=CARTESIAN_POINT('',(-0.5,-38.7742356128,-11.0174674429));
#75324=CARTESIAN_POINT('Origin',(2.38004060904018E-14,-38.7742356128,-0.229047725439793));
#75325=CARTESIAN_POINT('',(-0.5,-38.7742356128,-15.3918809766));
#75326=CARTESIAN_POINT('',(-0.5,-38.7742356128,0.));
#75327=CARTESIAN_POINT('Origin',(2.22044604925031E-15,-38.7742356128,-2.88657986402541E-14));
#75328=CARTESIAN_POINT('Origin',(-3.35265884719E-30,-38.7742356128,3.15283103411E-22));
#75329=CARTESIAN_POINT('',(-11.816958431,-38.7742356128,-9.87519586841));
#75330=CARTESIAN_POINT('',(-10.3256459325,-38.7742356128,-11.4254556179));
#75331=CARTESIAN_POINT('Origin',(4.59632332194815E-13,-38.7742356128,3.530509218308E-13));
#75332=CARTESIAN_POINT('',(-11.7961681305,-38.7742356128,-9.46800252678));
#75333=CARTESIAN_POINT('Origin',(-11.586757942,-38.7742356128,-9.68282192292));
#75334=CARTESIAN_POINT('',(-9.33306511227,-38.7742356128,-7.06692107621));
#75335=CARTESIAN_POINT('',(-11.7961681305,-38.7742356128,-9.46800252678));
#75336=CARTESIAN_POINT('',(-7.22695685732,-38.7742356128,-8.79725906681));
#75337=CARTESIAN_POINT('Ctrl Pts',(-7.22695685732232,-38.7742356128,-8.79725906681339));
#75338=CARTESIAN_POINT('Ctrl Pts',(-7.28150888554724,-38.7742356128,-8.76017689804407));
#75339=CARTESIAN_POINT('Ctrl Pts',(-7.3358430836494,-38.7742356128,-8.72268025917252));
#75340=CARTESIAN_POINT('Ctrl Pts',(-7.3899712392707,-38.7742356128,-8.68477139569698));
#75341=CARTESIAN_POINT('Ctrl Pts',(-7.46720182448399,-38.7742356128,-8.63068265616057));
#75342=CARTESIAN_POINT('Ctrl Pts',(-7.54401747222364,-38.7742356128,-8.57575348443564));
#75343=CARTESIAN_POINT('Ctrl Pts',(-7.6205551490896,-38.7742356128,-8.51991134544531));
#75344=CARTESIAN_POINT('Ctrl Pts',(-7.69952766934175,-38.7742356128,-8.46229273676896));
#75345=CARTESIAN_POINT('Ctrl Pts',(-7.77820421333981,-38.7742356128,-8.40370214573728));
#75346=CARTESIAN_POINT('Ctrl Pts',(-7.85668116624427,-38.7742356128,-8.34407402226636));
#75347=CARTESIAN_POINT('Ctrl Pts',(-7.9369257319336,-38.7742356128,-8.28310283653978));
#75348=CARTESIAN_POINT('Ctrl Pts',(-8.01696145430612,-38.7742356128,-8.2210468784774));
#75349=CARTESIAN_POINT('Ctrl Pts',(-8.09683736040204,-38.7742356128,-8.15785041906033));
#75350=CARTESIAN_POINT('Ctrl Pts',(-8.17873759713216,-38.7742356128,-8.09305234364884));
#75351=CARTESIAN_POINT('Ctrl Pts',(-8.26046963077621,-38.7742356128,-8.02705525395073));
#75352=CARTESIAN_POINT('Ctrl Pts',(-8.34203275379583,-38.7742356128,-7.95981359656426));
#75353=CARTESIAN_POINT('Ctrl Pts',(-8.42751622477607,-38.7742356128,-7.88933995535172));
#75354=CARTESIAN_POINT('Ctrl Pts',(-8.51281409409125,-38.7742356128,-7.81749921791734));
#75355=CARTESIAN_POINT('Ctrl Pts',(-8.59786908945091,-38.7742356128,-7.74425465003792));
#75356=CARTESIAN_POINT('Ctrl Pts',(-8.68560880784547,-38.7742356128,-7.66869815000525));
#75357=CARTESIAN_POINT('Ctrl Pts',(-8.77308976965873,-38.7742356128,-7.59164784533776));
#75358=CARTESIAN_POINT('Ctrl Pts',(-8.86019351231532,-38.7742356128,-7.51307941783206));
#75359=CARTESIAN_POINT('Ctrl Pts',(-8.95286440609457,-38.7742356128,-7.42948936558264));
#75360=CARTESIAN_POINT('Ctrl Pts',(-9.04510813530844,-38.7742356128,-7.34418092104821));
#75361=CARTESIAN_POINT('Ctrl Pts',(-9.13672354646749,-38.7742356128,-7.257142461433));
#75362=CARTESIAN_POINT('Ctrl Pts',(-9.20252620421849,-38.7742356128,-7.1946271935673));
#75363=CARTESIAN_POINT('Ctrl Pts',(-9.26800342965979,-38.7742356128,-7.1312198308518));
#75364=CARTESIAN_POINT('Ctrl Pts',(-9.33306511226659,-38.7742356128,-7.06692107620598));
#75365=CARTESIAN_POINT('',(-9.91508679725,-38.7742356128,-11.4177012033));
#75366=CARTESIAN_POINT('',(-9.91508679725,-38.7742356128,-11.4177012033));
#75367=CARTESIAN_POINT('Origin',(-10.1244969857,-38.7742356128,-11.2028818071));
#75368=CARTESIAN_POINT('Origin',(-3.35265884719E-30,-38.7742356128,3.15283103411E-22));
#75369=CARTESIAN_POINT('',(-12.5997104365,-38.7742356128,-8.85478949011));
#75370=CARTESIAN_POINT('',(-10.0162216343,-38.7742356128,-6.33635360057));
#75371=CARTESIAN_POINT('',(-12.5997104365,-38.7742356128,-8.85478949011));
#75372=CARTESIAN_POINT('Origin',(2.44249065417534E-14,-38.7742356128,-4.38538094726937E-14));
#75373=CARTESIAN_POINT('',(-11.9679209449,-38.7742356128,7.54064765005));
#75374=CARTESIAN_POINT('',(-11.9679209449,-38.7742356128,7.54064765005));
#75375=CARTESIAN_POINT('',(-11.5436913602,-38.7742356128,7.54605685771));
#75376=CARTESIAN_POINT('Origin',(-11.7585107564,-38.7742356128,7.7554670462));
#75377=CARTESIAN_POINT('',(-11.2644777756,-38.7742356128,7.83248271924));
#75378=CARTESIAN_POINT('',(-11.5436913602,-38.7742356128,7.54605685771));
#75379=CARTESIAN_POINT('',(-11.2698869833,-38.7742356128,8.25671230387));
#75380=CARTESIAN_POINT('Origin',(-11.4792971717,-38.7742356128,8.04189290772));
#75381=CARTESIAN_POINT('',(-12.1117355269,-38.7742356128,9.07736288456));
#75382=CARTESIAN_POINT('',(-11.2698869833,-38.7742356128,8.25671230387));
#75383=CARTESIAN_POINT('Origin',(-11.9023253384,-38.7742356128,9.2921822807));
#75384=CARTESIAN_POINT('',(-9.53740907755,-38.7742356128,11.7477944761));
#75385=CARTESIAN_POINT('Origin',(-9.74681926603,-38.7742356128,11.5329750799));
#75386=CARTESIAN_POINT('',(-8.68076107776,-38.7742356128,10.9127170933));
#75387=CARTESIAN_POINT('',(-8.68076107776,-38.7742356128,10.9127170933));
#75388=CARTESIAN_POINT('',(-8.25653149313,-38.7742356128,10.918126301));
#75389=CARTESIAN_POINT('Origin',(-8.47135088927,-38.7742356128,11.1275364894));
#75390=CARTESIAN_POINT('',(-7.97731790849,-38.7742356128,11.2045521625));
#75391=CARTESIAN_POINT('',(-8.25653149313,-38.7742356128,10.918126301));
#75392=CARTESIAN_POINT('',(-7.98272711615,-38.7742356128,11.6287817471));
#75393=CARTESIAN_POINT('Origin',(-8.19213730463,-38.7742356128,11.413962351));
#75394=CARTESIAN_POINT('',(-7.98272711615,-38.7742356128,11.6287817471));
#75395=CARTESIAN_POINT('',(-0.5,-38.7742356128,12.4465469186));
#75396=CARTESIAN_POINT('',(-0.5,-38.7742356128,0.));
#75397=CARTESIAN_POINT('',(-7.04251644773,-38.7742356128,5.33751720019));
#75398=CARTESIAN_POINT('Origin',(0.000416107150123801,-38.7742356128,5.42091963994));
#75399=CARTESIAN_POINT('',(-7.16875088157,-38.7742356128,5.23983755655));
#75400=CARTESIAN_POINT('Origin',(-7.14250943682,-38.7742356128,5.33633308276));
#75401=CARTESIAN_POINT('',(-11.0086556946,-38.7742356128,3.43000353527));
#75402=CARTESIAN_POINT('Ctrl Pts',(-11.0086556946,-38.7742356128,3.43000353527));
#75403=CARTESIAN_POINT('Ctrl Pts',(-10.8267791086,-38.7742356128,3.7279970062));
#75404=CARTESIAN_POINT('Ctrl Pts',(-10.6180941124,-38.7742356128,4.02812460647));
#75405=CARTESIAN_POINT('Ctrl Pts',(-10.3610804417,-38.7742356128,4.34854162483));
#75406=CARTESIAN_POINT('Ctrl Pts',(-9.81894561437,-38.7742356128,4.82846996464));
#75407=CARTESIAN_POINT('Ctrl Pts',(-9.1449448519,-38.7742356128,5.15260465424));
#75408=CARTESIAN_POINT('Ctrl Pts',(-8.86735473037,-38.7742356128,5.24791616482));
#75409=CARTESIAN_POINT('Ctrl Pts',(-8.35592834321,-38.7742356128,5.35778460397));
#75410=CARTESIAN_POINT('Ctrl Pts',(-7.83459380784,-38.7742356128,5.3594412401));
#75411=CARTESIAN_POINT('Ctrl Pts',(-7.6075384225,-38.7742356128,5.33903210576));
#75412=CARTESIAN_POINT('Ctrl Pts',(-7.38481168145,-38.7742356128,5.2985941411));
#75413=CARTESIAN_POINT('Ctrl Pts',(-7.16875088157,-38.7742356128,5.23983755655));
#75414=CARTESIAN_POINT('',(-11.8354184104,-38.7742356128,0.924526608307));
#75415=CARTESIAN_POINT('Ctrl Pts',(-11.0086556946,-38.7742356128,3.43000353527));
#75416=CARTESIAN_POINT('Ctrl Pts',(-11.0817932058,-38.7742356128,3.31017227332));
#75417=CARTESIAN_POINT('Ctrl Pts',(-11.1567853729,-38.7742356128,3.18040212706));
#75418=CARTESIAN_POINT('Ctrl Pts',(-11.2288017566,-38.7742356128,3.0447194315));
#75419=CARTESIAN_POINT('Ctrl Pts',(-11.4529799792,-38.7742356128,2.57934328034));
#75420=CARTESIAN_POINT('Ctrl Pts',(-11.6140362762,-38.7742356128,2.09446235244));
#75421=CARTESIAN_POINT('Ctrl Pts',(-11.6871718767,-38.7742356128,1.76491172368));
#75422=CARTESIAN_POINT('Ctrl Pts',(-11.7534189237,-38.7742356128,1.41966067629));
#75423=CARTESIAN_POINT('Ctrl Pts',(-11.809039671,-38.7742356128,1.08859783468));
#75424=CARTESIAN_POINT('Ctrl Pts',(-11.8179542567,-38.7742356128,1.03442695212));
#75425=CARTESIAN_POINT('Ctrl Pts',(-11.8267316409,-38.7742356128,0.979949794408));
#75426=CARTESIAN_POINT('Ctrl Pts',(-11.8354184104,-38.7742356128,0.924526608307));
#75427=CARTESIAN_POINT('Ctrl Pts',(-10.0162216343,-38.7742356128,-6.33635360057));
#75428=CARTESIAN_POINT('Ctrl Pts',(-10.3224768783,-38.7742356128,-5.97981782527));
#75429=CARTESIAN_POINT('Ctrl Pts',(-10.6115458029,-38.7742356128,-5.60497678219));
#75430=CARTESIAN_POINT('Ctrl Pts',(-10.876460919,-38.7742356128,-5.21255294902));
#75431=CARTESIAN_POINT('Ctrl Pts',(-11.5273586686,-38.7742356128,-4.07233951466));
#75432=CARTESIAN_POINT('Ctrl Pts',(-11.912489836,-38.7742356128,-2.80791655207));
#75433=CARTESIAN_POINT('Ctrl Pts',(-12.0219871572,-38.7742356128,-1.97477394764));
#75434=CARTESIAN_POINT('Ctrl Pts',(-12.0360485934,-38.7742356128,-0.887789304964));
#75435=CARTESIAN_POINT('Ctrl Pts',(-11.941568867,-38.7742356128,0.143912935026));
#75436=CARTESIAN_POINT('Ctrl Pts',(-11.9112061973,-38.7742356128,0.407077462691));
#75437=CARTESIAN_POINT('Ctrl Pts',(-11.8758398702,-38.7742356128,0.666630263604));
#75438=CARTESIAN_POINT('Ctrl Pts',(-11.8354184104,-38.7742356128,0.924526608307));
#75439=CARTESIAN_POINT('Origin',(-3.35265884719E-30,-38.2742356128,3.15283103411E-22));
#75440=CARTESIAN_POINT('',(-12.5997104365,-37.2742356128,-8.85478949011));
#75441=CARTESIAN_POINT('',(-12.5997104365,-38.2742356128,-8.85478949011));
#75442=CARTESIAN_POINT('Origin',(-3.35265884719E-30,-37.2742356128,3.15283103411E-22));
#75443=CARTESIAN_POINT('Origin',(-3.35265884719E-30,-36.1242356128,3.15283103411E-22));
#75444=CARTESIAN_POINT('',(-10.3256459325,-33.7742356128,-11.4254556179));
#75445=CARTESIAN_POINT('',(-10.3256459325,-36.1242356128,-11.4254556179));
#75446=CARTESIAN_POINT('',(-11.816958431,-33.7742356128,-9.87519586841));
#75447=CARTESIAN_POINT('Origin',(-3.35265884719E-30,-33.7742356128,3.15283103411E-22));
#75448=CARTESIAN_POINT('',(-11.816958431,-36.1242356128,-9.87519586841));
#75449=CARTESIAN_POINT('Origin',(-3.35265884719E-30,-38.2742356128,3.15283103411E-22));
#75450=CARTESIAN_POINT('',(-9.33467257157,-37.2742356128,-12.2484238978));
#75451=CARTESIAN_POINT('',(-9.33467257157,-38.2742356128,-12.2484238978));
#75452=CARTESIAN_POINT('',(-0.5,-37.2742356128,-15.3918809766));
#75453=CARTESIAN_POINT('',(-0.5,-38.2742356128,-15.3918809766));
#75454=CARTESIAN_POINT('Origin',(-3.35265884719E-30,-37.2742356128,3.15283103411E-22));
#75455=CARTESIAN_POINT('Origin',(-3.35265884719E-30,-38.2742356128,3.15283103411E-22));
#75456=CARTESIAN_POINT('',(9.33467257157,-38.7742356128,-12.2484238978));
#75457=CARTESIAN_POINT('',(9.33467257157,-37.2742356128,-12.2484238978));
#75458=CARTESIAN_POINT('',(9.33467257157,-38.2742356128,-12.2484238978));
#75459=CARTESIAN_POINT('',(0.5,-37.2742356128,-15.3918809766));
#75460=CARTESIAN_POINT('Origin',(-3.35265884719E-30,-37.2742356128,3.15283103411E-22));
#75461=CARTESIAN_POINT('',(0.5,-38.7742356128,-15.3918809766));
#75462=CARTESIAN_POINT('',(0.5,-38.2742356128,-15.3918809766));
#75463=CARTESIAN_POINT('Origin',(-3.35265884719E-30,-38.7742356128,3.15283103411E-22));
#75464=CARTESIAN_POINT('Origin',(-3.35265884719E-30,-36.1242356128,3.15283103411E-22));
#75465=CARTESIAN_POINT('',(10.3256459325,-38.7742356128,-11.4254556179));
#75466=CARTESIAN_POINT('',(11.816958431,-38.7742356128,-9.87519586841));
#75467=CARTESIAN_POINT('Origin',(-3.35265884719E-30,-38.7742356128,3.15283103411E-22));
#75468=CARTESIAN_POINT('',(11.816958431,-33.7742356128,-9.87519586841));
#75469=CARTESIAN_POINT('',(11.816958431,-36.1242356128,-9.87519586841));
#75470=CARTESIAN_POINT('',(10.3256459325,-33.7742356128,-11.4254556179));
#75471=CARTESIAN_POINT('Origin',(-3.35265884719E-30,-33.7742356128,3.15283103411E-22));
#75472=CARTESIAN_POINT('',(10.3256459325,-36.1242356128,-11.4254556179));
#75473=CARTESIAN_POINT('Origin',(-3.35265884719E-30,-38.2742356128,3.15283103411E-22));
#75474=CARTESIAN_POINT('',(12.5997104365,-38.7742356128,-8.85478949011));
#75475=CARTESIAN_POINT('',(12.5997104365,-37.2742356128,-8.85478949011));
#75476=CARTESIAN_POINT('',(12.5997104365,-38.2742356128,-8.85478949011));
#75477=CARTESIAN_POINT('Origin',(-3.35265884719E-30,-38.7742356128,3.15283103411E-22));
#75478=CARTESIAN_POINT('Origin',(-3.35265884719E-30,-37.2742356128,3.15283103411E-22));
#75479=CARTESIAN_POINT('Origin',(-3.5527136788E-15,-37.9242356128,-8.88178104417E-16));
#75480=CARTESIAN_POINT('Origin',(-3.5527136788E-15,-37.2742356128,-8.88178104417E-16));
#75481=CARTESIAN_POINT('Origin',(-3.35265884719E-30,-34.4742356128,3.15283103411E-22));
#75482=CARTESIAN_POINT('',(3.,-34.4742356128,0.));
#75483=CARTESIAN_POINT('Origin',(3.,-35.1742356128,16.6523581407));
#75484=CARTESIAN_POINT('Origin',(-3.35265884719E-30,-38.1842356129,3.15283103411E-22));
#75485=CARTESIAN_POINT('Origin',(-3.35265884719E-30,-33.4742356128,3.15283103411E-22));
#75486=CARTESIAN_POINT('Origin',(-3.35265884719E-30,-33.4742356128,3.15283103411E-22));
#75487=CARTESIAN_POINT('',(14.2514385284,-33.4742356128,0.));
#75488=CARTESIAN_POINT('Origin',(14.2514385284,-41.6742356128,2.4));
#75489=CARTESIAN_POINT('',(14.2514385284,-38.7742356128,0.));
#75490=CARTESIAN_POINT('Origin',(-3.35265884719E-30,-38.7742356128,3.15283103411E-22));
#75491=CARTESIAN_POINT('',(0.5,-38.7742356128,-11.0174674429));
#75492=CARTESIAN_POINT('',(0.5,-38.7742356128,0.));
#75493=CARTESIAN_POINT('',(1.48259713265,-38.7742356128,-10.9268000942));
#75494=CARTESIAN_POINT('Origin',(-8.24340595784179E-14,-38.7742356128,-0.229047725441214));
#75495=CARTESIAN_POINT('',(6.35435667676,-38.7742356128,-9.34315312398));
#75496=CARTESIAN_POINT('Ctrl Pts',(1.48259713264981,-38.7742356128,-10.9268000941986));
#75497=CARTESIAN_POINT('Ctrl Pts',(1.71328083841,-38.7742356128,-10.8948297336));
#75498=CARTESIAN_POINT('Ctrl Pts',(1.91354623838,-38.7742356128,-10.8659465412));
#75499=CARTESIAN_POINT('Ctrl Pts',(2.0855726443,-38.7742356128,-10.8395401686));
#75500=CARTESIAN_POINT('Ctrl Pts',(3.07854611663014,-38.7742356128,-10.6733698534529));
#75501=CARTESIAN_POINT('Ctrl Pts',(4.05813867422129,-38.7742356128,-10.4126758711658));
#75502=CARTESIAN_POINT('Ctrl Pts',(4.86043811084938,-38.7742356128,-10.1190200262464));
#75503=CARTESIAN_POINT('Ctrl Pts',(5.62475805694812,-38.7742356128,-9.76080244433078));
#75504=CARTESIAN_POINT('Ctrl Pts',(6.35435667676222,-38.7742356128,-9.34315312398388));
#75505=CARTESIAN_POINT('',(9.33467257157,-38.7742356128,-12.2484238978));
#75506=CARTESIAN_POINT('Origin',(-3.35265884719E-30,-38.7742356128,3.15283103411E-22));
#75507=CARTESIAN_POINT('',(11.7961681305,-38.7742356128,-9.46800252678));
#75508=CARTESIAN_POINT('',(9.33306511227,-38.7742356128,-7.06692107621));
#75509=CARTESIAN_POINT('',(11.7961681305,-38.7742356128,-9.46800252678));
#75510=CARTESIAN_POINT('Origin',(11.586757942,-38.7742356128,-9.68282192292));
#75511=CARTESIAN_POINT('',(9.91508679725,-38.7742356128,-11.4177012033));
#75512=CARTESIAN_POINT('Origin',(10.1244969857,-38.7742356128,-11.2028818071));
#75513=CARTESIAN_POINT('',(7.22695685732,-38.7742356128,-8.79725906681));
#75514=CARTESIAN_POINT('',(9.91508679725,-38.7742356128,-11.4177012033));
#75515=CARTESIAN_POINT('Ctrl Pts',(7.22695685732231,-38.7742356128,-8.7972590668134));
#75516=CARTESIAN_POINT('Ctrl Pts',(7.28150888554723,-38.7742356128,-8.76017689804407));
#75517=CARTESIAN_POINT('Ctrl Pts',(7.3358430836494,-38.7742356128,-8.72268025917252));
#75518=CARTESIAN_POINT('Ctrl Pts',(7.3899712392707,-38.7742356128,-8.68477139569698));
#75519=CARTESIAN_POINT('Ctrl Pts',(7.467201824484,-38.7742356128,-8.63068265616057));
#75520=CARTESIAN_POINT('Ctrl Pts',(7.54401747222365,-38.7742356128,-8.57575348443563));
#75521=CARTESIAN_POINT('Ctrl Pts',(7.62055514908962,-38.7742356128,-8.5199113454453));
#75522=CARTESIAN_POINT('Ctrl Pts',(7.69952766934177,-38.7742356128,-8.46229273676895));
#75523=CARTESIAN_POINT('Ctrl Pts',(7.77820421333981,-38.7742356128,-8.40370214573728));
#75524=CARTESIAN_POINT('Ctrl Pts',(7.85668116624427,-38.7742356128,-8.34407402226636));
#75525=CARTESIAN_POINT('Ctrl Pts',(7.93692573193363,-38.7742356128,-8.28310283653976));
#75526=CARTESIAN_POINT('Ctrl Pts',(8.01696145430617,-38.7742356128,-8.22104687847736));
#75527=CARTESIAN_POINT('Ctrl Pts',(8.09683736040211,-38.7742356128,-8.15785041906028));
#75528=CARTESIAN_POINT('Ctrl Pts',(8.1787375971322,-38.7742356128,-8.09305234364882));
#75529=CARTESIAN_POINT('Ctrl Pts',(8.2604696307762,-38.7742356128,-8.02705525395073));
#75530=CARTESIAN_POINT('Ctrl Pts',(8.34203275379579,-38.7742356128,-7.9598135965643));
#75531=CARTESIAN_POINT('Ctrl Pts',(8.42751622477602,-38.7742356128,-7.88933995535176));
#75532=CARTESIAN_POINT('Ctrl Pts',(8.5128140940912,-38.7742356128,-7.81749921791738));
#75533=CARTESIAN_POINT('Ctrl Pts',(8.59786908945085,-38.7742356128,-7.74425465003797));
#75534=CARTESIAN_POINT('Ctrl Pts',(8.68560880784544,-38.7742356128,-7.66869815000527));
#75535=CARTESIAN_POINT('Ctrl Pts',(8.77308976965874,-38.7742356128,-7.59164784533776));
#75536=CARTESIAN_POINT('Ctrl Pts',(8.86019351231535,-38.7742356128,-7.51307941783203));
#75537=CARTESIAN_POINT('Ctrl Pts',(8.9528644060946,-38.7742356128,-7.42948936558261));
#75538=CARTESIAN_POINT('Ctrl Pts',(9.04510813530846,-38.7742356128,-7.34418092104819));
#75539=CARTESIAN_POINT('Ctrl Pts',(9.1367235464675,-38.7742356128,-7.25714246143299));
#75540=CARTESIAN_POINT('Ctrl Pts',(9.2025262042184,-38.7742356128,-7.19462719356739));
#75541=CARTESIAN_POINT('Ctrl Pts',(9.2680034296596,-38.7742356128,-7.13121983085198));
#75542=CARTESIAN_POINT('Ctrl Pts',(9.3330651122663,-38.7742356128,-7.06692107620626));
#75543=CARTESIAN_POINT('Origin',(-3.35265884719E-30,-38.7742356128,3.15283103411E-22));
#75544=CARTESIAN_POINT('',(11.7961681305,-38.7742356128,9.46800252678));
#75545=CARTESIAN_POINT('Origin',(11.586757942,-38.7742356128,9.68282192292));
#75546=CARTESIAN_POINT('',(10.9208700025,-38.7742356128,8.61474463077));
#75547=CARTESIAN_POINT('',(10.9208700025,-38.7742356128,8.61474463077));
#75548=CARTESIAN_POINT('',(10.9154607948,-38.7742356128,8.19051504615));
#75549=CARTESIAN_POINT('Origin',(11.1302801909,-38.7742356128,8.39992523463));
#75550=CARTESIAN_POINT('',(11.1946743794,-38.7742356128,7.90408918462));
#75551=CARTESIAN_POINT('',(11.1946743794,-38.7742356128,7.90408918462));
#75552=CARTESIAN_POINT('',(11.6189039641,-38.7742356128,7.89867997696));
#75553=CARTESIAN_POINT('Origin',(11.4094937756,-38.7742356128,8.1134993731));
#75554=CARTESIAN_POINT('',(11.6189039641,-38.7742356128,7.89867997696));
#75555=CARTESIAN_POINT('',(10.0162216343,-38.7742356128,-6.33635360057));
#75556=CARTESIAN_POINT('',(12.5997104365,-38.7742356128,-8.85478949011));
#75557=CARTESIAN_POINT('',(11.8354184104,-38.7742356128,0.924526608307));
#75558=CARTESIAN_POINT('Ctrl Pts',(10.0162216343,-38.7742356128,-6.33635360057));
#75559=CARTESIAN_POINT('Ctrl Pts',(10.3224768783,-38.7742356128,-5.97981782527));
#75560=CARTESIAN_POINT('Ctrl Pts',(10.6115458029,-38.7742356128,-5.60497678219));
#75561=CARTESIAN_POINT('Ctrl Pts',(10.876460919,-38.7742356128,-5.21255294902));
#75562=CARTESIAN_POINT('Ctrl Pts',(11.5273586686,-38.7742356128,-4.07233951466));
#75563=CARTESIAN_POINT('Ctrl Pts',(11.912489836,-38.7742356128,-2.80791655207));
#75564=CARTESIAN_POINT('Ctrl Pts',(12.0219871572,-38.7742356128,-1.97477394764));
#75565=CARTESIAN_POINT('Ctrl Pts',(12.0360485934,-38.7742356128,-0.887789304964));
#75566=CARTESIAN_POINT('Ctrl Pts',(11.941568867,-38.7742356128,0.143912935026));
#75567=CARTESIAN_POINT('Ctrl Pts',(11.9112061973,-38.7742356128,0.407077462691));
#75568=CARTESIAN_POINT('Ctrl Pts',(11.8758398702,-38.7742356128,0.666630263604));
#75569=CARTESIAN_POINT('Ctrl Pts',(11.8354184104,-38.7742356128,0.924526608307));
#75570=CARTESIAN_POINT('',(11.0086556946,-38.7742356128,3.43000353527));
#75571=CARTESIAN_POINT('Ctrl Pts',(11.0086556946,-38.7742356128,3.43000353527));
#75572=CARTESIAN_POINT('Ctrl Pts',(11.0817932058,-38.7742356128,3.31017227332));
#75573=CARTESIAN_POINT('Ctrl Pts',(11.1567853729,-38.7742356128,3.18040212706));
#75574=CARTESIAN_POINT('Ctrl Pts',(11.2288017566,-38.7742356128,3.0447194315));
#75575=CARTESIAN_POINT('Ctrl Pts',(11.4529799792,-38.7742356128,2.57934328034));
#75576=CARTESIAN_POINT('Ctrl Pts',(11.6140362762,-38.7742356128,2.09446235244));
#75577=CARTESIAN_POINT('Ctrl Pts',(11.6871718767,-38.7742356128,1.76491172368));
#75578=CARTESIAN_POINT('Ctrl Pts',(11.7534189237,-38.7742356128,1.41966067629));
#75579=CARTESIAN_POINT('Ctrl Pts',(11.809039671,-38.7742356128,1.08859783468));
#75580=CARTESIAN_POINT('Ctrl Pts',(11.8179542567,-38.7742356128,1.03442695212));
#75581=CARTESIAN_POINT('Ctrl Pts',(11.8267316409,-38.7742356128,0.979949794408));
#75582=CARTESIAN_POINT('Ctrl Pts',(11.8354184104,-38.7742356128,0.924526608307));
#75583=CARTESIAN_POINT('',(7.16875088157,-38.7742356128,5.23983755655));
#75584=CARTESIAN_POINT('Ctrl Pts',(11.0086556946,-38.7742356128,3.43000353527));
#75585=CARTESIAN_POINT('Ctrl Pts',(10.8267791086,-38.7742356128,3.7279970062));
#75586=CARTESIAN_POINT('Ctrl Pts',(10.6180941124,-38.7742356128,4.02812460647));
#75587=CARTESIAN_POINT('Ctrl Pts',(10.3610804417,-38.7742356128,4.34854162483));
#75588=CARTESIAN_POINT('Ctrl Pts',(9.81894561437,-38.7742356128,4.82846996464));
#75589=CARTESIAN_POINT('Ctrl Pts',(9.1449448519,-38.7742356128,5.15260465424));
#75590=CARTESIAN_POINT('Ctrl Pts',(8.86735473037,-38.7742356128,5.24791616482));
#75591=CARTESIAN_POINT('Ctrl Pts',(8.35592834321,-38.7742356128,5.35778460397));
#75592=CARTESIAN_POINT('Ctrl Pts',(7.83459380784,-38.7742356128,5.3594412401));
#75593=CARTESIAN_POINT('Ctrl Pts',(7.6075384225,-38.7742356128,5.33903210576));
#75594=CARTESIAN_POINT('Ctrl Pts',(7.38481168145,-38.7742356128,5.2985941411));
#75595=CARTESIAN_POINT('Ctrl Pts',(7.16875088157,-38.7742356128,5.23983755655));
#75596=CARTESIAN_POINT('',(7.04251644773,-38.7742356128,5.33751720019));
#75597=CARTESIAN_POINT('Origin',(7.14250943682,-38.7742356128,5.33633308276));
#75598=CARTESIAN_POINT('',(0.5,-38.7742356128,12.4465469186));
#75599=CARTESIAN_POINT('Origin',(-0.00041610715012616,-38.7742356128,5.42091963994));
#75600=CARTESIAN_POINT('',(0.5,-38.7742356128,0.));
#75601=CARTESIAN_POINT('',(8.33174409695,-38.7742356128,11.2707494202));
#75602=CARTESIAN_POINT('',(8.33174409695,-38.7742356128,11.2707494202));
#75603=CARTESIAN_POINT('',(8.32633488929,-38.7742356128,10.8465198356));
#75604=CARTESIAN_POINT('Origin',(8.54115428543,-38.7742356128,11.0559300241));
#75605=CARTESIAN_POINT('',(8.60554847393,-38.7742356128,10.560093974));
#75606=CARTESIAN_POINT('',(8.60554847393,-38.7742356128,10.560093974));
#75607=CARTESIAN_POINT('',(9.02977805856,-38.7742356128,10.5546847664));
#75608=CARTESIAN_POINT('Origin',(8.82036787008,-38.7742356128,10.7695041625));
#75609=CARTESIAN_POINT('',(9.91508679725,-38.7742356128,11.4177012033));
#75610=CARTESIAN_POINT('',(9.02977805856,-38.7742356128,10.5546847664));
#75611=CARTESIAN_POINT('Origin',(10.1244969857,-38.7742356128,11.2028818071));
#75612=CARTESIAN_POINT('Origin',(-3.35265884719E-30,-44.4742356128,3.15283103411E-22));
#75613=CARTESIAN_POINT('',(-8.73272894647,-44.4742356128,11.6412701168));
#75614=CARTESIAN_POINT('Origin',(-7.48272894647,-44.4742356128,11.6412701168));
#75615=CARTESIAN_POINT('Origin',(4.74384247076,-41.1742356128,3.12351150632));
#75616=CARTESIAN_POINT('',(5.24384247076,-41.6742356128,3.12351150632));
#75617=CARTESIAN_POINT('',(5.24384247076,-41.1742356128,3.12351150632));
#75618=CARTESIAN_POINT('',(4.89234685393,-41.6742356128,2.64607413014));
#75619=CARTESIAN_POINT('Origin',(4.74384247076,-41.6742356128,3.12351150632));
#75620=CARTESIAN_POINT('',(4.89234685393,-41.1742356128,2.64607413014));
#75621=CARTESIAN_POINT('Origin',(6.82290383517,-40.1142356128,-3.56061176027));
#75622=CARTESIAN_POINT('',(0.48735027394,-41.6742356128,-2.10776590718));
#75623=CARTESIAN_POINT('Origin',(6.82290383517,-41.6742356128,-3.56061176027));
#75624=CARTESIAN_POINT('',(0.48735027394,-40.1142356128,-2.10776590718));
#75625=CARTESIAN_POINT('Origin',(-4.99600361081E-16,-41.1742356128,-1.99600853387));
#75626=CARTESIAN_POINT('',(-0.48735027394,-41.6742356128,-2.10776590718));
#75627=CARTESIAN_POINT('Origin',(-4.99600361081E-16,-41.6742356128,-1.99600853387));
#75628=CARTESIAN_POINT('',(-0.48735027394,-41.1742356128,-2.10776590718));
#75629=CARTESIAN_POINT('Origin',(-6.82290383517,-40.1142356128,-3.56061176027));
#75630=CARTESIAN_POINT('',(-4.89234685393,-41.6742356128,2.64607413014));
#75631=CARTESIAN_POINT('',(-4.89234685393,-40.1142356128,2.64607413014));
#75632=CARTESIAN_POINT('Origin',(-6.82290383517,-41.6742356128,-3.56061176027));
#75633=CARTESIAN_POINT('Origin',(-4.74384247076,-41.1742356128,3.12351150632));
#75634=CARTESIAN_POINT('',(-5.24384247076,-41.6742356128,3.12351150632));
#75635=CARTESIAN_POINT('Origin',(-4.74384247076,-41.6742356128,3.12351150632));
#75636=CARTESIAN_POINT('',(-5.24384247076,-41.1742356128,3.12351150632));
#75637=CARTESIAN_POINT('Origin',(-5.24384247076,-41.6742356128,6.92091963994));
#75638=CARTESIAN_POINT('',(-5.24384247076,-41.6742356128,6.92091963994));
#75639=CARTESIAN_POINT('',(-5.24384247076,-41.6742356128,5.02221557313));
#75640=CARTESIAN_POINT('',(-5.24384247076,-41.1742356128,6.92091963994));
#75641=CARTESIAN_POINT('Origin',(-0.000416107150126,-40.1142356128,6.92091963994));
#75642=CARTESIAN_POINT('',(-0.000416107143134986,-41.6742356128,12.1643459815524));
#75643=CARTESIAN_POINT('Origin',(-0.000416107150126,-41.6742356128,6.92091963994));
#75644=CARTESIAN_POINT('',(-0.000416107150124,-40.1142356128,12.1643460036));
#75645=CARTESIAN_POINT('Origin',(0.000416107150126,-40.1142356128,6.92091963994));
#75646=CARTESIAN_POINT('',(5.24384247076,-41.6742356128,6.92091963994));
#75647=CARTESIAN_POINT('Origin',(0.000416107150126,-41.6742356128,6.92091963994));
#75648=CARTESIAN_POINT('',(5.24384247076,-40.1142356128,6.92091963994));
#75649=CARTESIAN_POINT('Origin',(5.24384247076,-41.6742356128,6.92091963994));
#75650=CARTESIAN_POINT('',(5.24384247076,-41.6742356128,5.02221557313));
#75651=CARTESIAN_POINT('Origin',(6.82290383517,-40.1142356128,-3.56061176027));
#75652=CARTESIAN_POINT('',(12.3229038352,-41.6742356128,-3.56061176027));
#75653=CARTESIAN_POINT('',(12.32290383517,-40.1142356128,-3.56061176027));
#75654=CARTESIAN_POINT('Origin',(6.82290383517,-41.6742356128,-3.56061176027));
#75655=CARTESIAN_POINT('Origin',(-6.82290383517,-40.1142356128,-3.56061176027));
#75656=CARTESIAN_POINT('',(-12.3229038352,-41.6742356128,-3.56061176027));
#75657=CARTESIAN_POINT('Origin',(-6.82290383517,-41.6742356128,-3.56061176027));
#75658=CARTESIAN_POINT('',(-12.32290383517,-40.1142356128,-3.56061176027));
#75659=CARTESIAN_POINT('Origin',(-3.35265884719E-30,-44.4742356128,3.15283103411E-22));
#75660=CARTESIAN_POINT('',(8.73272894647,-44.4742356128,11.6412701168));
#75661=CARTESIAN_POINT('Origin',(7.48272894647,-44.4742356128,11.6412701168));
#75662=CARTESIAN_POINT('Origin',(0.000416107150126,-37.6642356128,5.42091963994));
#75663=CARTESIAN_POINT('',(-0.5,-37.2742356128,12.4465469186));
#75664=CARTESIAN_POINT('',(-7.04251644773,-37.2742356128,5.33751720019));
#75665=CARTESIAN_POINT('Origin',(0.000416107150126,-37.2742356128,5.42091963994));
#75666=CARTESIAN_POINT('',(-7.04251644773,-37.6642356128,5.33751720019));
#75667=CARTESIAN_POINT('',(-0.5,-37.6642356128,12.4465469186));
#75668=CARTESIAN_POINT('Origin',(-7.14250943682,-38.2742356128,5.33633308276));
#75669=CARTESIAN_POINT('',(-7.16875088104636,-37.2742356128,5.23983755640952));
#75670=CARTESIAN_POINT('Origin',(-7.14250943682,-37.2742356128,5.33633308276));
#75671=CARTESIAN_POINT('',(-7.16875088157,-38.2742356128,5.23983755655));
#75672=CARTESIAN_POINT('Ctrl Pts',(-11.0086556946,-38.7742356128,3.43000353527));
#75673=CARTESIAN_POINT('Ctrl Pts',(-11.0086556946,-36.9742356128,3.43000353527));
#75674=CARTESIAN_POINT('Ctrl Pts',(-10.8267791086,-38.7742356128,3.7279970062));
#75675=CARTESIAN_POINT('Ctrl Pts',(-10.8267791086,-36.9742356128,3.7279970062));
#75676=CARTESIAN_POINT('Ctrl Pts',(-10.6180941124,-38.7742356128,4.02812460647));
#75677=CARTESIAN_POINT('Ctrl Pts',(-10.6180941124,-36.9742356128,4.02812460647));
#75678=CARTESIAN_POINT('Ctrl Pts',(-10.3610804417,-38.7742356128,4.34854162483));
#75679=CARTESIAN_POINT('Ctrl Pts',(-10.3610804417,-36.9742356128,4.34854162483));
#75680=CARTESIAN_POINT('Ctrl Pts',(-9.81894561437,-38.7742356128,4.82846996464));
#75681=CARTESIAN_POINT('Ctrl Pts',(-9.81894561437,-36.9742356128,4.82846996464));
#75682=CARTESIAN_POINT('Ctrl Pts',(-9.1449448519,-38.7742356128,5.15260465424));
#75683=CARTESIAN_POINT('Ctrl Pts',(-9.1449448519,-36.9742356128,5.15260465424));
#75684=CARTESIAN_POINT('Ctrl Pts',(-8.86735473037,-38.7742356128,5.24791616482));
#75685=CARTESIAN_POINT('Ctrl Pts',(-8.86735473037,-36.9742356128,5.24791616482));
#75686=CARTESIAN_POINT('Ctrl Pts',(-8.35592834321,-38.7742356128,5.35778460397));
#75687=CARTESIAN_POINT('Ctrl Pts',(-8.35592834321,-36.9742356128,5.35778460397));
#75688=CARTESIAN_POINT('Ctrl Pts',(-7.83459380784,-38.7742356128,5.3594412401));
#75689=CARTESIAN_POINT('Ctrl Pts',(-7.83459380784,-36.9742356128,5.3594412401));
#75690=CARTESIAN_POINT('Ctrl Pts',(-7.6075384225,-38.7742356128,5.33903210576));
#75691=CARTESIAN_POINT('Ctrl Pts',(-7.6075384225,-36.9742356128,5.33903210576));
#75692=CARTESIAN_POINT('Ctrl Pts',(-7.38481168145,-38.7742356128,5.2985941411));
#75693=CARTESIAN_POINT('Ctrl Pts',(-7.38481168145,-36.9742356128,5.2985941411));
#75694=CARTESIAN_POINT('Ctrl Pts',(-7.16875088157,-38.7742356128,5.23983755655));
#75695=CARTESIAN_POINT('Ctrl Pts',(-7.16875088157,-36.9742356128,5.23983755655));
#75696=CARTESIAN_POINT('',(-11.0086556946,-37.2742356128,3.43000353527));
#75697=CARTESIAN_POINT('',(-11.0086556946,-37.6642356128,3.43000353527));
#75698=CARTESIAN_POINT('Ctrl Pts',(-11.0086556946,-37.2742356128,3.43000353527));
#75699=CARTESIAN_POINT('Ctrl Pts',(-10.8267791086,-37.2742356128,3.7279970062));
#75700=CARTESIAN_POINT('Ctrl Pts',(-10.6180941124,-37.2742356128,4.02812460647));
#75701=CARTESIAN_POINT('Ctrl Pts',(-10.3610804417,-37.2742356128,4.34854162483));
#75702=CARTESIAN_POINT('Ctrl Pts',(-9.81894561437,-37.2742356128,4.82846996464));
#75703=CARTESIAN_POINT('Ctrl Pts',(-9.1449448519,-37.2742356128,5.15260465424));
#75704=CARTESIAN_POINT('Ctrl Pts',(-8.86735473037,-37.2742356128,5.24791616482));
#75705=CARTESIAN_POINT('Ctrl Pts',(-8.35592834321,-37.2742356128,5.35778460397));
#75706=CARTESIAN_POINT('Ctrl Pts',(-7.83459380784,-37.2742356128,5.3594412401));
#75707=CARTESIAN_POINT('Ctrl Pts',(-7.6075384225,-37.2742356128,5.33903210576));
#75708=CARTESIAN_POINT('Ctrl Pts',(-7.38481168145,-37.2742356128,5.2985941411));
#75709=CARTESIAN_POINT('Ctrl Pts',(-7.16875088157,-37.2742356128,5.23983755655));
#75710=CARTESIAN_POINT('Ctrl Pts',(-11.0086556946,-38.7742356128,3.43000353527));
#75711=CARTESIAN_POINT('Ctrl Pts',(-11.0086556946,-36.9742356128,3.43000353527));
#75712=CARTESIAN_POINT('Ctrl Pts',(-11.0817932058,-38.7742356128,3.31017227332));
#75713=CARTESIAN_POINT('Ctrl Pts',(-11.0817932058,-36.9742356128,3.31017227332));
#75714=CARTESIAN_POINT('Ctrl Pts',(-11.1567853729,-38.7742356128,3.18040212706));
#75715=CARTESIAN_POINT('Ctrl Pts',(-11.1567853729,-36.9742356128,3.18040212706));
#75716=CARTESIAN_POINT('Ctrl Pts',(-11.2288017566,-38.7742356128,3.0447194315));
#75717=CARTESIAN_POINT('Ctrl Pts',(-11.2288017566,-36.9742356128,3.0447194315));
#75718=CARTESIAN_POINT('Ctrl Pts',(-11.4529799792,-38.7742356128,2.57934328034));
#75719=CARTESIAN_POINT('Ctrl Pts',(-11.4529799792,-36.9742356128,2.57934328034));
#75720=CARTESIAN_POINT('Ctrl Pts',(-11.6140362762,-38.7742356128,2.09446235244));
#75721=CARTESIAN_POINT('Ctrl Pts',(-11.6140362762,-36.9742356128,2.09446235244));
#75722=CARTESIAN_POINT('Ctrl Pts',(-11.6871718767,-38.7742356128,1.76491172368));
#75723=CARTESIAN_POINT('Ctrl Pts',(-11.6871718767,-36.9742356128,1.76491172368));
#75724=CARTESIAN_POINT('Ctrl Pts',(-11.7534189237,-38.7742356128,1.41966067629));
#75725=CARTESIAN_POINT('Ctrl Pts',(-11.7534189237,-36.9742356128,1.41966067629));
#75726=CARTESIAN_POINT('Ctrl Pts',(-11.809039671,-38.7742356128,1.08859783468));
#75727=CARTESIAN_POINT('Ctrl Pts',(-11.809039671,-36.9742356128,1.08859783468));
#75728=CARTESIAN_POINT('Ctrl Pts',(-11.8179542567,-38.7742356128,1.03442695212));
#75729=CARTESIAN_POINT('Ctrl Pts',(-11.8179542567,-36.9742356128,1.03442695212));
#75730=CARTESIAN_POINT('Ctrl Pts',(-11.8267316409,-38.7742356128,0.979949794408));
#75731=CARTESIAN_POINT('Ctrl Pts',(-11.8267316409,-36.9742356128,0.979949794408));
#75732=CARTESIAN_POINT('Ctrl Pts',(-11.8354184104,-38.7742356128,0.924526608307));
#75733=CARTESIAN_POINT('Ctrl Pts',(-11.8354184104,-36.9742356128,0.924526608307));
#75734=CARTESIAN_POINT('',(-11.8354184104,-37.2742356128,0.924526608307));
#75735=CARTESIAN_POINT('Ctrl Pts',(-11.0086556946,-37.2742356128,3.43000353527));
#75736=CARTESIAN_POINT('Ctrl Pts',(-11.0817932058,-37.2742356128,3.31017227332));
#75737=CARTESIAN_POINT('Ctrl Pts',(-11.1567853729,-37.2742356128,3.18040212706));
#75738=CARTESIAN_POINT('Ctrl Pts',(-11.2288017566,-37.2742356128,3.0447194315));
#75739=CARTESIAN_POINT('Ctrl Pts',(-11.4529799792,-37.2742356128,2.57934328034));
#75740=CARTESIAN_POINT('Ctrl Pts',(-11.6140362762,-37.2742356128,2.09446235244));
#75741=CARTESIAN_POINT('Ctrl Pts',(-11.6871718767,-37.2742356128,1.76491172368));
#75742=CARTESIAN_POINT('Ctrl Pts',(-11.7534189237,-37.2742356128,1.41966067629));
#75743=CARTESIAN_POINT('Ctrl Pts',(-11.809039671,-37.2742356128,1.08859783468));
#75744=CARTESIAN_POINT('Ctrl Pts',(-11.8179542567,-37.2742356128,1.03442695212));
#75745=CARTESIAN_POINT('Ctrl Pts',(-11.8267316409,-37.2742356128,0.979949794408));
#75746=CARTESIAN_POINT('Ctrl Pts',(-11.8354184104,-37.2742356128,0.924526608307));
#75747=CARTESIAN_POINT('',(-11.8354184104,-37.6642356128,0.924526608307));
#75748=CARTESIAN_POINT('Ctrl Pts',(-10.0162216343,-38.7742356128,-6.33635360057));
#75749=CARTESIAN_POINT('Ctrl Pts',(-10.0162216343,-36.9742356128,-6.33635360057));
#75750=CARTESIAN_POINT('Ctrl Pts',(-10.3224768783,-38.7742356128,-5.97981782527));
#75751=CARTESIAN_POINT('Ctrl Pts',(-10.3224768783,-36.9742356128,-5.97981782527));
#75752=CARTESIAN_POINT('Ctrl Pts',(-10.6115458029,-38.7742356128,-5.60497678219));
#75753=CARTESIAN_POINT('Ctrl Pts',(-10.6115458029,-36.9742356128,-5.60497678219));
#75754=CARTESIAN_POINT('Ctrl Pts',(-10.876460919,-38.7742356128,-5.21255294902));
#75755=CARTESIAN_POINT('Ctrl Pts',(-10.876460919,-36.9742356128,-5.21255294902));
#75756=CARTESIAN_POINT('Ctrl Pts',(-11.5273586686,-38.7742356128,-4.07233951466));
#75757=CARTESIAN_POINT('Ctrl Pts',(-11.5273586686,-36.9742356128,-4.07233951466));
#75758=CARTESIAN_POINT('Ctrl Pts',(-11.912489836,-38.7742356128,-2.80791655207));
#75759=CARTESIAN_POINT('Ctrl Pts',(-11.912489836,-36.9742356128,-2.80791655207));
#75760=CARTESIAN_POINT('Ctrl Pts',(-12.0219871572,-38.7742356128,-1.97477394764));
#75761=CARTESIAN_POINT('Ctrl Pts',(-12.0219871572,-36.9742356128,-1.97477394764));
#75762=CARTESIAN_POINT('Ctrl Pts',(-12.0360485934,-38.7742356128,-0.887789304964));
#75763=CARTESIAN_POINT('Ctrl Pts',(-12.0360485934,-36.9742356128,-0.887789304964));
#75764=CARTESIAN_POINT('Ctrl Pts',(-11.941568867,-38.7742356128,0.143912935026));
#75765=CARTESIAN_POINT('Ctrl Pts',(-11.941568867,-36.9742356128,0.143912935026));
#75766=CARTESIAN_POINT('Ctrl Pts',(-11.9112061973,-38.7742356128,0.407077462691));
#75767=CARTESIAN_POINT('Ctrl Pts',(-11.9112061973,-36.9742356128,0.407077462691));
#75768=CARTESIAN_POINT('Ctrl Pts',(-11.8758398702,-38.7742356128,0.666630263604));
#75769=CARTESIAN_POINT('Ctrl Pts',(-11.8758398702,-36.9742356128,0.666630263604));
#75770=CARTESIAN_POINT('Ctrl Pts',(-11.8354184104,-38.7742356128,0.924526608307));
#75771=CARTESIAN_POINT('Ctrl Pts',(-11.8354184104,-36.9742356128,0.924526608307));
#75772=CARTESIAN_POINT('',(-10.0162216343,-37.2742356128,-6.33635360057));
#75773=CARTESIAN_POINT('Ctrl Pts',(-10.0162216343,-37.2742356128,-6.33635360057));
#75774=CARTESIAN_POINT('Ctrl Pts',(-10.3224768783,-37.2742356128,-5.97981782527));
#75775=CARTESIAN_POINT('Ctrl Pts',(-10.6115458029,-37.2742356128,-5.60497678219));
#75776=CARTESIAN_POINT('Ctrl Pts',(-10.876460919,-37.2742356128,-5.21255294902));
#75777=CARTESIAN_POINT('Ctrl Pts',(-11.5273586686,-37.2742356128,-4.07233951466));
#75778=CARTESIAN_POINT('Ctrl Pts',(-11.912489836,-37.2742356128,-2.80791655207));
#75779=CARTESIAN_POINT('Ctrl Pts',(-12.0219871572,-37.2742356128,-1.97477394764));
#75780=CARTESIAN_POINT('Ctrl Pts',(-12.0360485934,-37.2742356128,-0.887789304964));
#75781=CARTESIAN_POINT('Ctrl Pts',(-11.941568867,-37.2742356128,0.143912935026));
#75782=CARTESIAN_POINT('Ctrl Pts',(-11.9112061973,-37.2742356128,0.407077462691));
#75783=CARTESIAN_POINT('Ctrl Pts',(-11.8758398702,-37.2742356128,0.666630263604));
#75784=CARTESIAN_POINT('Ctrl Pts',(-11.8354184104,-37.2742356128,0.924526608307));
#75785=CARTESIAN_POINT('',(-10.0162216343,-37.6642356128,-6.33635360057));
#75786=CARTESIAN_POINT('Ctrl Pts',(-7.22695646354,-38.7742356128,-8.79725933449));
#75787=CARTESIAN_POINT('Ctrl Pts',(-7.22695646354,-36.9742356128,-8.79725933449));
#75788=CARTESIAN_POINT('Ctrl Pts',(-7.25968775986,-38.7742356128,-8.77500998089));
#75789=CARTESIAN_POINT('Ctrl Pts',(-7.25968775986,-36.9742356128,-8.77500998089));
#75790=CARTESIAN_POINT('Ctrl Pts',(-7.29235374605,-38.7742356128,-8.75263626704));
#75791=CARTESIAN_POINT('Ctrl Pts',(-7.29235374605,-36.9742356128,-8.75263626704));
#75792=CARTESIAN_POINT('Ctrl Pts',(-7.3249555226,-38.7742356128,-8.73013845435));
#75793=CARTESIAN_POINT('Ctrl Pts',(-7.3249555226,-36.9742356128,-8.73013845435));
#75794=CARTESIAN_POINT('Ctrl Pts',(-7.75723078658,-38.7742356128,-8.42961072436));
#75795=CARTESIAN_POINT('Ctrl Pts',(-7.75723078658,-36.9742356128,-8.42961072436));
#75796=CARTESIAN_POINT('Ctrl Pts',(-8.17860364499,-38.7742356128,-8.10725352709));
#75797=CARTESIAN_POINT('Ctrl Pts',(-8.17860364499,-36.9742356128,-8.10725352709));
#75798=CARTESIAN_POINT('Ctrl Pts',(-8.5693207085,-38.7742356128,-7.78543946907));
#75799=CARTESIAN_POINT('Ctrl Pts',(-8.5693207085,-36.9742356128,-7.78543946907));
#75800=CARTESIAN_POINT('Ctrl Pts',(-8.95699215017,-38.7742356128,-7.43858429643));
#75801=CARTESIAN_POINT('Ctrl Pts',(-8.95699215017,-36.9742356128,-7.43858429643));
#75802=CARTESIAN_POINT('Ctrl Pts',(-9.33306737369,-38.7742356128,-7.0669188413));
#75803=CARTESIAN_POINT('Ctrl Pts',(-9.33306737369,-36.9742356128,-7.0669188413));
#75804=CARTESIAN_POINT('',(-9.33306511227,-37.2742356128,-7.06692107621));
#75805=CARTESIAN_POINT('',(-9.33306511227,-37.6642356128,-7.06692107621));
#75806=CARTESIAN_POINT('',(-7.22695685732,-37.2742356128,-8.79725906681));
#75807=CARTESIAN_POINT('Ctrl Pts',(-7.22695685732231,-37.2742356128,-8.7972590668134));
#75808=CARTESIAN_POINT('Ctrl Pts',(-7.28150888554724,-37.2742356128,-8.76017689804407));
#75809=CARTESIAN_POINT('Ctrl Pts',(-7.3358430836494,-37.2742356128,-8.72268025917252));
#75810=CARTESIAN_POINT('Ctrl Pts',(-7.3899712392707,-37.2742356128,-8.68477139569698));
#75811=CARTESIAN_POINT('Ctrl Pts',(-7.46720182448402,-37.2742356128,-8.63068265616056));
#75812=CARTESIAN_POINT('Ctrl Pts',(-7.54401747222369,-37.2742356128,-8.5757534844356));
#75813=CARTESIAN_POINT('Ctrl Pts',(-7.62055514908967,-37.2742356128,-8.51991134544526));
#75814=CARTESIAN_POINT('Ctrl Pts',(-7.69952766934181,-37.2742356128,-8.46229273676892));
#75815=CARTESIAN_POINT('Ctrl Pts',(-7.77820421333984,-37.2742356128,-8.40370214573726));
#75816=CARTESIAN_POINT('Ctrl Pts',(-7.85668116624429,-37.2742356128,-8.34407402226635));
#75817=CARTESIAN_POINT('Ctrl Pts',(-7.93692573193362,-37.2742356128,-8.28310283653977));
#75818=CARTESIAN_POINT('Ctrl Pts',(-8.01696145430614,-37.2742356128,-8.22104687847739));
#75819=CARTESIAN_POINT('Ctrl Pts',(-8.09683736040206,-37.2742356128,-8.15785041906032));
#75820=CARTESIAN_POINT('Ctrl Pts',(-8.17873759713219,-37.2742356128,-8.09305234364882));
#75821=CARTESIAN_POINT('Ctrl Pts',(-8.26046963077625,-37.2742356128,-8.0270552539507));
#75822=CARTESIAN_POINT('Ctrl Pts',(-8.34203275379588,-37.2742356128,-7.95981359656422));
#75823=CARTESIAN_POINT('Ctrl Pts',(-8.42751622477611,-37.2742356128,-7.88933995535169));
#75824=CARTESIAN_POINT('Ctrl Pts',(-8.51281409409128,-37.2742356128,-7.81749921791731));
#75825=CARTESIAN_POINT('Ctrl Pts',(-8.59786908945093,-37.2742356128,-7.7442546500379));
#75826=CARTESIAN_POINT('Ctrl Pts',(-8.68560880784551,-37.2742356128,-7.66869815000521));
#75827=CARTESIAN_POINT('Ctrl Pts',(-8.77308976965879,-37.2742356128,-7.59164784533771));
#75828=CARTESIAN_POINT('Ctrl Pts',(-8.86019351231539,-37.2742356128,-7.513079417832));
#75829=CARTESIAN_POINT('Ctrl Pts',(-8.95286440609459,-37.2742356128,-7.42948936558262));
#75830=CARTESIAN_POINT('Ctrl Pts',(-9.04510813530841,-37.2742356128,-7.34418092104824));
#75831=CARTESIAN_POINT('Ctrl Pts',(-9.13672354646741,-37.2742356128,-7.25714246143308));
#75832=CARTESIAN_POINT('Ctrl Pts',(-9.20252620421834,-37.2742356128,-7.19462719356745));
#75833=CARTESIAN_POINT('Ctrl Pts',(-9.26800342965957,-37.2742356128,-7.13121983085201));
#75834=CARTESIAN_POINT('Ctrl Pts',(-9.3330651122663,-37.2742356128,-7.06692107620626));
#75835=CARTESIAN_POINT('',(-7.22695685732,-37.6642356128,-8.79725906681));
#75836=CARTESIAN_POINT('Ctrl Pts',(-1.48259713264,-38.7742356128,-10.9268000942));
#75837=CARTESIAN_POINT('Ctrl Pts',(-1.48259713264,-36.9742356128,-10.9268000942));
#75838=CARTESIAN_POINT('Ctrl Pts',(-1.71328083841,-38.7742356128,-10.8948297336));
#75839=CARTESIAN_POINT('Ctrl Pts',(-1.71328083841,-36.9742356128,-10.8948297336));
#75840=CARTESIAN_POINT('Ctrl Pts',(-1.91354623838,-38.7742356128,-10.8659465412));
#75841=CARTESIAN_POINT('Ctrl Pts',(-1.91354623838,-36.9742356128,-10.8659465412));
#75842=CARTESIAN_POINT('Ctrl Pts',(-2.0855726443,-38.7742356128,-10.8395401686));
#75843=CARTESIAN_POINT('Ctrl Pts',(-2.0855726443,-36.9742356128,-10.8395401686));
#75844=CARTESIAN_POINT('Ctrl Pts',(-3.07854615175,-38.7742356128,-10.6733698476));
#75845=CARTESIAN_POINT('Ctrl Pts',(-3.07854615175,-36.9742356128,-10.6733698476));
#75846=CARTESIAN_POINT('Ctrl Pts',(-4.05813874351,-38.7742356128,-10.4126758527));
#75847=CARTESIAN_POINT('Ctrl Pts',(-4.05813874351,-36.9742356128,-10.4126758527));
#75848=CARTESIAN_POINT('Ctrl Pts',(-4.8604382114,-38.7742356128,-10.1190199895));
#75849=CARTESIAN_POINT('Ctrl Pts',(-4.8604382114,-36.9742356128,-10.1190199895));
#75850=CARTESIAN_POINT('Ctrl Pts',(-5.62475818467,-38.7742356128,-9.76080238448));
#75851=CARTESIAN_POINT('Ctrl Pts',(-5.62475818467,-36.9742356128,-9.76080238448));
#75852=CARTESIAN_POINT('Ctrl Pts',(-6.35435682916,-38.7742356128,-9.34315303675));
#75853=CARTESIAN_POINT('Ctrl Pts',(-6.35435682916,-36.9742356128,-9.34315303675));
#75854=CARTESIAN_POINT('',(-1.48259713217599,-37.2742356128,-10.9268000942492));
#75855=CARTESIAN_POINT('',(-6.35435667676,-37.2742356128,-9.34315312398));
#75856=CARTESIAN_POINT('Ctrl Pts',(-1.48259713264,-37.2742356128,-10.9268000942));
#75857=CARTESIAN_POINT('Ctrl Pts',(-1.71328083841,-37.2742356128,-10.8948297336));
#75858=CARTESIAN_POINT('Ctrl Pts',(-1.91354623838,-37.2742356128,-10.8659465412));
#75859=CARTESIAN_POINT('Ctrl Pts',(-2.0855726443,-37.2742356128,-10.8395401686));
#75860=CARTESIAN_POINT('Ctrl Pts',(-3.07854611663017,-37.2742356128,-10.6733698534772));
#75861=CARTESIAN_POINT('Ctrl Pts',(-4.05813867421687,-37.2742356128,-10.4126758711406));
#75862=CARTESIAN_POINT('Ctrl Pts',(-4.86043811085114,-37.2742356128,-10.1190200263027));
#75863=CARTESIAN_POINT('Ctrl Pts',(-5.62475805695127,-37.2742356128,-9.76080244433856));
#75864=CARTESIAN_POINT('Ctrl Pts',(-6.35435667676406,-37.2742356128,-9.34315312398709));
#75865=CARTESIAN_POINT('',(-1.48259713265,-37.6642356128,-10.9268000942));
#75866=CARTESIAN_POINT('',(-6.35435667676,-37.6642356128,-9.34315312398));
#75867=CARTESIAN_POINT('Origin',(-7.77156117238E-15,-38.2742356128,-0.229047725441));
#75868=CARTESIAN_POINT('',(-0.5,-37.2742356128,-11.0174674429));
#75869=CARTESIAN_POINT('Origin',(-7.77156117238E-15,-37.2742356128,-0.229047725441));
#75870=CARTESIAN_POINT('',(-0.5,-38.2742356128,-11.0174674429));
#75871=CARTESIAN_POINT('Origin',(-7.77156117238E-15,-38.2742356128,-0.229047725441));
#75872=CARTESIAN_POINT('',(0.5,-37.2742356128,-11.0174674429));
#75873=CARTESIAN_POINT('',(1.48259713217599,-37.2742356128,-10.9268000942492));
#75874=CARTESIAN_POINT('Origin',(-7.77156117238E-15,-37.2742356128,-0.229047725441));
#75875=CARTESIAN_POINT('',(1.48259713265,-38.2742356128,-10.9268000942));
#75876=CARTESIAN_POINT('',(0.5,-38.2742356128,-11.0174674429));
#75877=CARTESIAN_POINT('Ctrl Pts',(1.48259713264,-38.7742356128,-10.9268000942));
#75878=CARTESIAN_POINT('Ctrl Pts',(1.48259713264,-36.9742356128,-10.9268000942));
#75879=CARTESIAN_POINT('Ctrl Pts',(1.71328083841,-38.7742356128,-10.8948297336));
#75880=CARTESIAN_POINT('Ctrl Pts',(1.71328083841,-36.9742356128,-10.8948297336));
#75881=CARTESIAN_POINT('Ctrl Pts',(1.91354623838,-38.7742356128,-10.8659465412));
#75882=CARTESIAN_POINT('Ctrl Pts',(1.91354623838,-36.9742356128,-10.8659465412));
#75883=CARTESIAN_POINT('Ctrl Pts',(2.0855726443,-38.7742356128,-10.8395401686));
#75884=CARTESIAN_POINT('Ctrl Pts',(2.0855726443,-36.9742356128,-10.8395401686));
#75885=CARTESIAN_POINT('Ctrl Pts',(3.07854619941,-38.7742356128,-10.6733698396));
#75886=CARTESIAN_POINT('Ctrl Pts',(3.07854619941,-36.9742356128,-10.6733698396));
#75887=CARTESIAN_POINT('Ctrl Pts',(4.05813883755,-38.7742356128,-10.4126758277));
#75888=CARTESIAN_POINT('Ctrl Pts',(4.05813883755,-36.9742356128,-10.4126758277));
#75889=CARTESIAN_POINT('Ctrl Pts',(4.86043834785,-38.7742356128,-10.1190199395));
#75890=CARTESIAN_POINT('Ctrl Pts',(4.86043834785,-36.9742356128,-10.1190199395));
#75891=CARTESIAN_POINT('Ctrl Pts',(5.62475835799,-38.7742356128,-9.76080230324));
#75892=CARTESIAN_POINT('Ctrl Pts',(5.62475835799,-36.9742356128,-9.76080230324));
#75893=CARTESIAN_POINT('Ctrl Pts',(6.35435703597,-38.7742356128,-9.34315291836));
#75894=CARTESIAN_POINT('Ctrl Pts',(6.35435703597,-36.9742356128,-9.34315291836));
#75895=CARTESIAN_POINT('',(6.35435667676,-37.2742356128,-9.34315312398));
#75896=CARTESIAN_POINT('',(6.35435667676,-37.6642356128,-9.34315312398));
#75897=CARTESIAN_POINT('Ctrl Pts',(1.48259713264,-37.2742356128,-10.9268000942));
#75898=CARTESIAN_POINT('Ctrl Pts',(1.71328083841,-37.2742356128,-10.8948297336));
#75899=CARTESIAN_POINT('Ctrl Pts',(1.91354623838,-37.2742356128,-10.8659465412));
#75900=CARTESIAN_POINT('Ctrl Pts',(2.0855726443,-37.2742356128,-10.8395401686));
#75901=CARTESIAN_POINT('Ctrl Pts',(3.07854611663014,-37.2742356128,-10.6733698534529));
#75902=CARTESIAN_POINT('Ctrl Pts',(4.05813867422129,-37.2742356128,-10.4126758711658));
#75903=CARTESIAN_POINT('Ctrl Pts',(4.86043811084938,-37.2742356128,-10.1190200262464));
#75904=CARTESIAN_POINT('Ctrl Pts',(5.62475805694812,-37.2742356128,-9.76080244433078));
#75905=CARTESIAN_POINT('Ctrl Pts',(6.35435667676222,-37.2742356128,-9.34315312398388));
#75906=CARTESIAN_POINT('Ctrl Pts',(7.22695646354,-38.7742356128,-8.79725933449));
#75907=CARTESIAN_POINT('Ctrl Pts',(7.22695646354,-36.9742356128,-8.79725933449));
#75908=CARTESIAN_POINT('Ctrl Pts',(7.25968775986,-38.7742356128,-8.77500998089));
#75909=CARTESIAN_POINT('Ctrl Pts',(7.25968775986,-36.9742356128,-8.77500998089));
#75910=CARTESIAN_POINT('Ctrl Pts',(7.29235374605,-38.7742356128,-8.75263626704));
#75911=CARTESIAN_POINT('Ctrl Pts',(7.29235374605,-36.9742356128,-8.75263626704));
#75912=CARTESIAN_POINT('Ctrl Pts',(7.3249555226,-38.7742356128,-8.73013845435));
#75913=CARTESIAN_POINT('Ctrl Pts',(7.3249555226,-36.9742356128,-8.73013845435));
#75914=CARTESIAN_POINT('Ctrl Pts',(7.75723078658,-38.7742356128,-8.42961072436));
#75915=CARTESIAN_POINT('Ctrl Pts',(7.75723078658,-36.9742356128,-8.42961072436));
#75916=CARTESIAN_POINT('Ctrl Pts',(8.17860364499,-38.7742356128,-8.10725352709));
#75917=CARTESIAN_POINT('Ctrl Pts',(8.17860364499,-36.9742356128,-8.10725352709));
#75918=CARTESIAN_POINT('Ctrl Pts',(8.5693207085,-38.7742356128,-7.78543946907));
#75919=CARTESIAN_POINT('Ctrl Pts',(8.5693207085,-36.9742356128,-7.78543946907));
#75920=CARTESIAN_POINT('Ctrl Pts',(8.95699215017,-38.7742356128,-7.43858429643));
#75921=CARTESIAN_POINT('Ctrl Pts',(8.95699215017,-36.9742356128,-7.43858429643));
#75922=CARTESIAN_POINT('Ctrl Pts',(9.33306737369,-38.7742356128,-7.0669188413));
#75923=CARTESIAN_POINT('Ctrl Pts',(9.33306737369,-36.9742356128,-7.0669188413));
#75924=CARTESIAN_POINT('',(9.33306511227,-37.2742356128,-7.06692107621));
#75925=CARTESIAN_POINT('',(9.33306511227,-37.6642356128,-7.06692107621));
#75926=CARTESIAN_POINT('',(7.22695685732,-37.2742356128,-8.79725906681));
#75927=CARTESIAN_POINT('',(7.22695685732,-37.6642356128,-8.79725906681));
#75928=CARTESIAN_POINT('Ctrl Pts',(7.22695685732231,-37.2742356128,-8.7972590668134));
#75929=CARTESIAN_POINT('Ctrl Pts',(7.28150888554723,-37.2742356128,-8.76017689804407));
#75930=CARTESIAN_POINT('Ctrl Pts',(7.3358430836494,-37.2742356128,-8.72268025917252));
#75931=CARTESIAN_POINT('Ctrl Pts',(7.3899712392707,-37.2742356128,-8.68477139569698));
#75932=CARTESIAN_POINT('Ctrl Pts',(7.46720182448396,-37.2742356128,-8.6306826561606));
#75933=CARTESIAN_POINT('Ctrl Pts',(7.54401747222357,-37.2742356128,-8.57575348443569));
#75934=CARTESIAN_POINT('Ctrl Pts',(7.62055514908949,-37.2742356128,-8.51991134544539));
#75935=CARTESIAN_POINT('Ctrl Pts',(7.69952766934165,-37.2742356128,-8.46229273676904));
#75936=CARTESIAN_POINT('Ctrl Pts',(7.77820421333969,-37.2742356128,-8.40370214573737));
#75937=CARTESIAN_POINT('Ctrl Pts',(7.85668116624415,-37.2742356128,-8.34407402226645));
#75938=CARTESIAN_POINT('Ctrl Pts',(7.93692573193349,-37.2742356128,-8.28310283653987));
#75939=CARTESIAN_POINT('Ctrl Pts',(8.01696145430602,-37.2742356128,-8.22104687847748));
#75940=CARTESIAN_POINT('Ctrl Pts',(8.09683736040194,-37.2742356128,-8.15785041906041));
#75941=CARTESIAN_POINT('Ctrl Pts',(8.17873759713205,-37.2742356128,-8.09305234364894));
#75942=CARTESIAN_POINT('Ctrl Pts',(8.26046963077608,-37.2742356128,-8.02705525395084));
#75943=CARTESIAN_POINT('Ctrl Pts',(8.34203275379568,-37.2742356128,-7.95981359656439));
#75944=CARTESIAN_POINT('Ctrl Pts',(8.42751622477591,-37.2742356128,-7.88933995535186));
#75945=CARTESIAN_POINT('Ctrl Pts',(8.51281409409109,-37.2742356128,-7.81749921791748));
#75946=CARTESIAN_POINT('Ctrl Pts',(8.59786908945074,-37.2742356128,-7.74425465003807));
#75947=CARTESIAN_POINT('Ctrl Pts',(8.68560880784532,-37.2742356128,-7.66869815000537));
#75948=CARTESIAN_POINT('Ctrl Pts',(8.77308976965861,-37.2742356128,-7.59164784533787));
#75949=CARTESIAN_POINT('Ctrl Pts',(8.86019351231522,-37.2742356128,-7.51307941783215));
#75950=CARTESIAN_POINT('Ctrl Pts',(8.95286440609447,-37.2742356128,-7.42948936558273));
#75951=CARTESIAN_POINT('Ctrl Pts',(9.04510813530834,-37.2742356128,-7.3441809210483));
#75952=CARTESIAN_POINT('Ctrl Pts',(9.13672354646738,-37.2742356128,-7.25714246143311));
#75953=CARTESIAN_POINT('Ctrl Pts',(9.20252620421832,-37.2742356128,-7.19462719356746));
#75954=CARTESIAN_POINT('Ctrl Pts',(9.26800342965956,-37.2742356128,-7.13121983085202));
#75955=CARTESIAN_POINT('Ctrl Pts',(9.3330651122663,-37.2742356128,-7.06692107620626));
#75956=CARTESIAN_POINT('Ctrl Pts',(10.0162216343,-38.7742356128,-6.33635360057));
#75957=CARTESIAN_POINT('Ctrl Pts',(10.0162216343,-36.9742356128,-6.33635360057));
#75958=CARTESIAN_POINT('Ctrl Pts',(10.3224768783,-38.7742356128,-5.97981782527));
#75959=CARTESIAN_POINT('Ctrl Pts',(10.3224768783,-36.9742356128,-5.97981782527));
#75960=CARTESIAN_POINT('Ctrl Pts',(10.6115458029,-38.7742356128,-5.60497678219));
#75961=CARTESIAN_POINT('Ctrl Pts',(10.6115458029,-36.9742356128,-5.60497678219));
#75962=CARTESIAN_POINT('Ctrl Pts',(10.876460919,-38.7742356128,-5.21255294902));
#75963=CARTESIAN_POINT('Ctrl Pts',(10.876460919,-36.9742356128,-5.21255294902));
#75964=CARTESIAN_POINT('Ctrl Pts',(11.5273586686,-38.7742356128,-4.07233951466));
#75965=CARTESIAN_POINT('Ctrl Pts',(11.5273586686,-36.9742356128,-4.07233951466));
#75966=CARTESIAN_POINT('Ctrl Pts',(11.912489836,-38.7742356128,-2.80791655207));
#75967=CARTESIAN_POINT('Ctrl Pts',(11.912489836,-36.9742356128,-2.80791655207));
#75968=CARTESIAN_POINT('Ctrl Pts',(12.0219871572,-38.7742356128,-1.97477394764));
#75969=CARTESIAN_POINT('Ctrl Pts',(12.0219871572,-36.9742356128,-1.97477394764));
#75970=CARTESIAN_POINT('Ctrl Pts',(12.0360485934,-38.7742356128,-0.887789304964));
#75971=CARTESIAN_POINT('Ctrl Pts',(12.0360485934,-36.9742356128,-0.887789304964));
#75972=CARTESIAN_POINT('Ctrl Pts',(11.941568867,-38.7742356128,0.143912935026));
#75973=CARTESIAN_POINT('Ctrl Pts',(11.941568867,-36.9742356128,0.143912935026));
#75974=CARTESIAN_POINT('Ctrl Pts',(11.9112061973,-38.7742356128,0.407077462691));
#75975=CARTESIAN_POINT('Ctrl Pts',(11.9112061973,-36.9742356128,0.407077462691));
#75976=CARTESIAN_POINT('Ctrl Pts',(11.8758398702,-38.7742356128,0.666630263604));
#75977=CARTESIAN_POINT('Ctrl Pts',(11.8758398702,-36.9742356128,0.666630263604));
#75978=CARTESIAN_POINT('Ctrl Pts',(11.8354184104,-38.7742356128,0.924526608307));
#75979=CARTESIAN_POINT('Ctrl Pts',(11.8354184104,-36.9742356128,0.924526608307));
#75980=CARTESIAN_POINT('',(10.0162216343,-37.2742356128,-6.33635360057));
#75981=CARTESIAN_POINT('',(10.0162216343,-37.6642356128,-6.33635360057));
#75982=CARTESIAN_POINT('',(11.8354184104,-37.2742356128,0.924526608307));
#75983=CARTESIAN_POINT('Ctrl Pts',(10.0162216343,-37.2742356128,-6.33635360057));
#75984=CARTESIAN_POINT('Ctrl Pts',(10.3224768783,-37.2742356128,-5.97981782527));
#75985=CARTESIAN_POINT('Ctrl Pts',(10.6115458029,-37.2742356128,-5.60497678219));
#75986=CARTESIAN_POINT('Ctrl Pts',(10.876460919,-37.2742356128,-5.21255294902));
#75987=CARTESIAN_POINT('Ctrl Pts',(11.5273586686,-37.2742356128,-4.07233951466));
#75988=CARTESIAN_POINT('Ctrl Pts',(11.912489836,-37.2742356128,-2.80791655207));
#75989=CARTESIAN_POINT('Ctrl Pts',(12.0219871572,-37.2742356128,-1.97477394764));
#75990=CARTESIAN_POINT('Ctrl Pts',(12.0360485934,-37.2742356128,-0.887789304964));
#75991=CARTESIAN_POINT('Ctrl Pts',(11.941568867,-37.2742356128,0.143912935026));
#75992=CARTESIAN_POINT('Ctrl Pts',(11.9112061973,-37.2742356128,0.407077462691));
#75993=CARTESIAN_POINT('Ctrl Pts',(11.8758398702,-37.2742356128,0.666630263604));
#75994=CARTESIAN_POINT('Ctrl Pts',(11.8354184104,-37.2742356128,0.924526608307));
#75995=CARTESIAN_POINT('',(11.8354184104,-37.6642356128,0.924526608307));
#75996=CARTESIAN_POINT('Ctrl Pts',(11.0086556946,-38.7742356128,3.43000353527));
#75997=CARTESIAN_POINT('Ctrl Pts',(11.0086556946,-36.9742356128,3.43000353527));
#75998=CARTESIAN_POINT('Ctrl Pts',(11.0817932058,-38.7742356128,3.31017227332));
#75999=CARTESIAN_POINT('Ctrl Pts',(11.0817932058,-36.9742356128,3.31017227332));
#76000=CARTESIAN_POINT('Ctrl Pts',(11.1567853729,-38.7742356128,3.18040212706));
#76001=CARTESIAN_POINT('Ctrl Pts',(11.1567853729,-36.9742356128,3.18040212706));
#76002=CARTESIAN_POINT('Ctrl Pts',(11.2288017566,-38.7742356128,3.0447194315));
#76003=CARTESIAN_POINT('Ctrl Pts',(11.2288017566,-36.9742356128,3.0447194315));
#76004=CARTESIAN_POINT('Ctrl Pts',(11.4529799792,-38.7742356128,2.57934328034));
#76005=CARTESIAN_POINT('Ctrl Pts',(11.4529799792,-36.9742356128,2.57934328034));
#76006=CARTESIAN_POINT('Ctrl Pts',(11.6140362762,-38.7742356128,2.09446235244));
#76007=CARTESIAN_POINT('Ctrl Pts',(11.6140362762,-36.9742356128,2.09446235244));
#76008=CARTESIAN_POINT('Ctrl Pts',(11.6871718767,-38.7742356128,1.76491172368));
#76009=CARTESIAN_POINT('Ctrl Pts',(11.6871718767,-36.9742356128,1.76491172368));
#76010=CARTESIAN_POINT('Ctrl Pts',(11.7534189237,-38.7742356128,1.41966067629));
#76011=CARTESIAN_POINT('Ctrl Pts',(11.7534189237,-36.9742356128,1.41966067629));
#76012=CARTESIAN_POINT('Ctrl Pts',(11.809039671,-38.7742356128,1.08859783468));
#76013=CARTESIAN_POINT('Ctrl Pts',(11.809039671,-36.9742356128,1.08859783468));
#76014=CARTESIAN_POINT('Ctrl Pts',(11.8179542567,-38.7742356128,1.03442695212));
#76015=CARTESIAN_POINT('Ctrl Pts',(11.8179542567,-36.9742356128,1.03442695212));
#76016=CARTESIAN_POINT('Ctrl Pts',(11.8267316409,-38.7742356128,0.979949794408));
#76017=CARTESIAN_POINT('Ctrl Pts',(11.8267316409,-36.9742356128,0.979949794408));
#76018=CARTESIAN_POINT('Ctrl Pts',(11.8354184104,-38.7742356128,0.924526608307));
#76019=CARTESIAN_POINT('Ctrl Pts',(11.8354184104,-36.9742356128,0.924526608307));
#76020=CARTESIAN_POINT('',(11.0086556946,-37.2742356128,3.43000353527));
#76021=CARTESIAN_POINT('',(11.0086556946,-37.6642356128,3.43000353527));
#76022=CARTESIAN_POINT('Ctrl Pts',(11.0086556946,-37.2742356128,3.43000353527));
#76023=CARTESIAN_POINT('Ctrl Pts',(11.0817932058,-37.2742356128,3.31017227332));
#76024=CARTESIAN_POINT('Ctrl Pts',(11.1567853729,-37.2742356128,3.18040212706));
#76025=CARTESIAN_POINT('Ctrl Pts',(11.2288017566,-37.2742356128,3.0447194315));
#76026=CARTESIAN_POINT('Ctrl Pts',(11.4529799792,-37.2742356128,2.57934328034));
#76027=CARTESIAN_POINT('Ctrl Pts',(11.6140362762,-37.2742356128,2.09446235244));
#76028=CARTESIAN_POINT('Ctrl Pts',(11.6871718767,-37.2742356128,1.76491172368));
#76029=CARTESIAN_POINT('Ctrl Pts',(11.7534189237,-37.2742356128,1.41966067629));
#76030=CARTESIAN_POINT('Ctrl Pts',(11.809039671,-37.2742356128,1.08859783468));
#76031=CARTESIAN_POINT('Ctrl Pts',(11.8179542567,-37.2742356128,1.03442695212));
#76032=CARTESIAN_POINT('Ctrl Pts',(11.8267316409,-37.2742356128,0.979949794408));
#76033=CARTESIAN_POINT('Ctrl Pts',(11.8354184104,-37.2742356128,0.924526608307));
#76034=CARTESIAN_POINT('Ctrl Pts',(11.0086556946,-38.7742356128,3.43000353527));
#76035=CARTESIAN_POINT('Ctrl Pts',(11.0086556946,-36.9742356128,3.43000353527));
#76036=CARTESIAN_POINT('Ctrl Pts',(10.8267791086,-38.7742356128,3.7279970062));
#76037=CARTESIAN_POINT('Ctrl Pts',(10.8267791086,-36.9742356128,3.7279970062));
#76038=CARTESIAN_POINT('Ctrl Pts',(10.6180941124,-38.7742356128,4.02812460647));
#76039=CARTESIAN_POINT('Ctrl Pts',(10.6180941124,-36.9742356128,4.02812460647));
#76040=CARTESIAN_POINT('Ctrl Pts',(10.3610804417,-38.7742356128,4.34854162483));
#76041=CARTESIAN_POINT('Ctrl Pts',(10.3610804417,-36.9742356128,4.34854162483));
#76042=CARTESIAN_POINT('Ctrl Pts',(9.81894561437,-38.7742356128,4.82846996464));
#76043=CARTESIAN_POINT('Ctrl Pts',(9.81894561437,-36.9742356128,4.82846996464));
#76044=CARTESIAN_POINT('Ctrl Pts',(9.1449448519,-38.7742356128,5.15260465424));
#76045=CARTESIAN_POINT('Ctrl Pts',(9.1449448519,-36.9742356128,5.15260465424));
#76046=CARTESIAN_POINT('Ctrl Pts',(8.86735473037,-38.7742356128,5.24791616482));
#76047=CARTESIAN_POINT('Ctrl Pts',(8.86735473037,-36.9742356128,5.24791616482));
#76048=CARTESIAN_POINT('Ctrl Pts',(8.35592834321,-38.7742356128,5.35778460397));
#76049=CARTESIAN_POINT('Ctrl Pts',(8.35592834321,-36.9742356128,5.35778460397));
#76050=CARTESIAN_POINT('Ctrl Pts',(7.83459380784,-38.7742356128,5.3594412401));
#76051=CARTESIAN_POINT('Ctrl Pts',(7.83459380784,-36.9742356128,5.3594412401));
#76052=CARTESIAN_POINT('Ctrl Pts',(7.6075384225,-38.7742356128,5.33903210576));
#76053=CARTESIAN_POINT('Ctrl Pts',(7.6075384225,-36.9742356128,5.33903210576));
#76054=CARTESIAN_POINT('Ctrl Pts',(7.38481168145,-38.7742356128,5.2985941411));
#76055=CARTESIAN_POINT('Ctrl Pts',(7.38481168145,-36.9742356128,5.2985941411));
#76056=CARTESIAN_POINT('Ctrl Pts',(7.16875088157,-38.7742356128,5.23983755655));
#76057=CARTESIAN_POINT('Ctrl Pts',(7.16875088157,-36.9742356128,5.23983755655));
#76058=CARTESIAN_POINT('',(7.16875088104636,-37.2742356128,5.23983755640952));
#76059=CARTESIAN_POINT('Ctrl Pts',(11.0086556946,-37.2742356128,3.43000353527));
#76060=CARTESIAN_POINT('Ctrl Pts',(10.8267791086,-37.2742356128,3.7279970062));
#76061=CARTESIAN_POINT('Ctrl Pts',(10.6180941124,-37.2742356128,4.02812460647));
#76062=CARTESIAN_POINT('Ctrl Pts',(10.3610804417,-37.2742356128,4.34854162483));
#76063=CARTESIAN_POINT('Ctrl Pts',(9.81894561437,-37.2742356128,4.82846996464));
#76064=CARTESIAN_POINT('Ctrl Pts',(9.1449448519,-37.2742356128,5.15260465424));
#76065=CARTESIAN_POINT('Ctrl Pts',(8.86735473037,-37.2742356128,5.24791616482));
#76066=CARTESIAN_POINT('Ctrl Pts',(8.35592834321,-37.2742356128,5.35778460397));
#76067=CARTESIAN_POINT('Ctrl Pts',(7.83459380784,-37.2742356128,5.3594412401));
#76068=CARTESIAN_POINT('Ctrl Pts',(7.6075384225,-37.2742356128,5.33903210576));
#76069=CARTESIAN_POINT('Ctrl Pts',(7.38481168145,-37.2742356128,5.2985941411));
#76070=CARTESIAN_POINT('Ctrl Pts',(7.16875088157,-37.2742356128,5.23983755655));
#76071=CARTESIAN_POINT('',(7.16875088157,-37.6642356128,5.23983755655));
#76072=CARTESIAN_POINT('Origin',(7.14250943682,-38.2742356128,5.33633308276));
#76073=CARTESIAN_POINT('',(7.04251644773,-37.2742356128,5.33751720019));
#76074=CARTESIAN_POINT('Origin',(7.14250943682,-37.2742356128,5.33633308276));
#76075=CARTESIAN_POINT('',(7.04251644773,-38.2742356128,5.33751720019));
#76076=CARTESIAN_POINT('Origin',(-0.000416107150126,-37.6642356128,5.42091963994));
#76077=CARTESIAN_POINT('',(0.5,-37.2742356128,12.4465469186));
#76078=CARTESIAN_POINT('Origin',(-0.000416107150126,-37.2742356128,5.42091963994));
#76079=CARTESIAN_POINT('',(0.5,-37.6642356128,12.4465469186));
#76080=CARTESIAN_POINT('Origin',(-7.48272894647,-41.3342356129,11.6412701168));
#76081=CARTESIAN_POINT('',(-8.73272894647,-40.7742356128,11.6412701168));
#76082=CARTESIAN_POINT('Origin',(-7.48272894647,-40.7742356128,11.6412701168));
#76083=CARTESIAN_POINT('',(-8.73272894647,-41.3342356129,11.6412701168));
#76084=CARTESIAN_POINT('Origin',(-3.35265884719E-30,-41.6742356128,3.15283103411E-22));
#76085=CARTESIAN_POINT('',(-4.44384247076,-41.6742356128,6.92091963994));
#76086=CARTESIAN_POINT('Origin',(-0.000416107150126,-41.6742356128,6.92091963994));
#76087=CARTESIAN_POINT('',(4.44384247076,-41.6742356128,3.34084221874));
#76088=CARTESIAN_POINT('',(4.44384247076,-41.6742356128,5.13088092934));
#76089=CARTESIAN_POINT('',(2.13594446644908E-16,-41.6742356128,-0.964849202557427));
#76090=CARTESIAN_POINT('Origin',(6.82290383517,-41.6742356128,-3.56061176027));
#76091=CARTESIAN_POINT('',(-4.44384247076,-41.6742356128,3.34084221874));
#76092=CARTESIAN_POINT('Origin',(-6.82290383517,-41.6742356128,-3.56061176027));
#76093=CARTESIAN_POINT('',(-4.44384247076,-41.6742356128,5.13088092934));
#76094=CARTESIAN_POINT('Origin',(-3.35265884719E-30,-41.6742356128,3.15283103411E-22));
#76095=CARTESIAN_POINT('',(11.5229038352,-41.6742356128,-3.56061176027));
#76096=CARTESIAN_POINT('Origin',(6.82290383517,-41.6742356128,-3.56061176027));
#76097=CARTESIAN_POINT('Origin',(-3.35265884719E-30,-41.6742356128,3.15283103411E-22));
#76098=CARTESIAN_POINT('',(-11.5229038352,-41.6742356128,-3.56061176027));
#76099=CARTESIAN_POINT('Origin',(-6.82290383517,-41.6742356128,-3.56061176027));
#76100=CARTESIAN_POINT('Origin',(7.48272894647,-41.3342356129,11.6412701168));
#76101=CARTESIAN_POINT('',(8.73272894647,-40.7742356128,11.6412701168));
#76102=CARTESIAN_POINT('',(8.73272894647,-41.3342356129,11.6412701168));
#76103=CARTESIAN_POINT('Origin',(7.48272894647,-40.7742356128,11.6412701168));
#76104=CARTESIAN_POINT('Origin',(-3.35265884719E-30,-40.7742356128,3.15283103411E-22));
#76105=CARTESIAN_POINT('Origin',(-0.000416107150126,-40.1142356128,6.92091963994));
#76106=CARTESIAN_POINT('',(-4.44384247076,-39.7742356128,6.92091963994));
#76107=CARTESIAN_POINT('',(-4.44384247076,-40.1142356128,6.92091963994));
#76108=CARTESIAN_POINT('',(-3.64378781517,-39.7742356128,9.46451560746));
#76109=CARTESIAN_POINT('Origin',(-0.000416107150126,-39.7742356128,6.92091963994));
#76110=CARTESIAN_POINT('Origin',(-0.000416107150126,-39.7742356128,6.92091963994));
#76111=CARTESIAN_POINT('Origin',(4.44384247076,-41.6742356128,6.92091963994));
#76112=CARTESIAN_POINT('',(4.44384253205641,-39.7742356128,5.42595709132001));
#76113=CARTESIAN_POINT('',(4.44384247076,-39.7742356128,6.17343837159));
#76114=CARTESIAN_POINT('',(4.44384264824955,-39.7742356128,5.30375137006997));
#76115=CARTESIAN_POINT('Ctrl Pts',(4.44384282525,-39.7742356128,5.30375137007));
#76116=CARTESIAN_POINT('Ctrl Pts',(4.44414005184279,-39.7742356128,5.32817576412788));
#76117=CARTESIAN_POINT('Ctrl Pts',(4.44428140248426,-39.7742356128,5.35261020505899));
#76118=CARTESIAN_POINT('Ctrl Pts',(4.44427352568687,-39.7742356128,5.37705311235898));
#76119=CARTESIAN_POINT('Ctrl Pts',(4.44412423208254,-39.7742356128,5.40150273088309));
#76120=CARTESIAN_POINT('Ctrl Pts',(4.44384259285,-39.7742356128,5.42595709132));
#76121=CARTESIAN_POINT('',(4.44384247076,-39.7742356128,3.34084221874));
#76122=CARTESIAN_POINT('',(4.44384247076,-39.7742356128,4.32229681001));
#76123=CARTESIAN_POINT('',(4.44384247076,-40.7242356128,3.34084221874));
#76124=CARTESIAN_POINT('Origin',(6.82290383517,-40.1142356128,-3.56061176027));
#76125=CARTESIAN_POINT('',(3.94523376325645,-39.7742356128,3.14826407381823));
#76126=CARTESIAN_POINT('Origin',(6.82290383517,-39.7742356128,-3.56061176027));
#76127=CARTESIAN_POINT('',(2.13594446644908E-16,-39.7742356128,-0.964849202557427));
#76128=CARTESIAN_POINT('Origin',(6.82290383517,-39.7742356128,-3.56061176027));
#76129=CARTESIAN_POINT('',(0.,-40.1142356128,-0.964849202557427));
#76130=CARTESIAN_POINT('Origin',(-6.82290383517,-40.1142356128,-3.56061176027));
#76131=CARTESIAN_POINT('',(-3.94523376325647,-39.7742356128,3.14826407381824));
#76132=CARTESIAN_POINT('Origin',(-6.82290383517,-39.7742356128,-3.56061176027));
#76133=CARTESIAN_POINT('',(-4.44384247076,-39.7742356128,3.34084221874));
#76134=CARTESIAN_POINT('Origin',(-6.82290383517,-39.7742356128,-3.56061176027));
#76135=CARTESIAN_POINT('',(-4.44384247076,-40.1142356128,3.34084221874));
#76136=CARTESIAN_POINT('Origin',(-4.44384247076,-41.6742356128,6.92091963994));
#76137=CARTESIAN_POINT('',(-4.44384264824955,-39.7742356128,5.30375137006997));
#76138=CARTESIAN_POINT('',(-4.44384247076,-39.7742356128,4.32229681001));
#76139=CARTESIAN_POINT('',(-4.44384253205641,-39.7742356128,5.42595709132));
#76140=CARTESIAN_POINT('',(-4.44384282525,-39.7742356128,5.30375137007));
#76141=CARTESIAN_POINT('',(-4.44384247076,-39.7742356128,6.17343837159));
#76142=CARTESIAN_POINT('Origin',(6.82290383517,-40.1142356128,-3.56061176027));
#76143=CARTESIAN_POINT('',(11.52290383517,-39.7742356128,-3.56061176027));
#76144=CARTESIAN_POINT('',(11.52290383517,-40.1142356128,-3.56061176027));
#76145=CARTESIAN_POINT('',(4.25781969055054,-39.7742356128,-7.49892908595644));
#76146=CARTESIAN_POINT('Origin',(6.82290383517,-39.7742356128,-3.56061176027));
#76147=CARTESIAN_POINT('',(2.26246783444344,-39.7742356128,-4.69745981422045));
#76148=CARTESIAN_POINT('Origin',(6.82290383517,-39.7742356128,-3.56061176027));
#76149=CARTESIAN_POINT('',(2.12330457313532,-39.7742356128,-3.4993320503742));
#76150=CARTESIAN_POINT('Origin',(6.82290383517,-39.7742356128,-3.56061176027));
#76151=CARTESIAN_POINT('',(6.02437852526,-39.7742356128,1.07105719697));
#76152=CARTESIAN_POINT('Origin',(6.82290383517,-39.7742356128,-3.56061176027));
#76153=CARTESIAN_POINT('',(7.04639034599947,-39.7742356128,1.1340718008604));
#76154=CARTESIAN_POINT('Origin',(6.82290383517,-39.7742356128,-3.56061176027));
#76155=CARTESIAN_POINT('',(9.24345637220266,-39.7742356128,0.468150497498442));
#76156=CARTESIAN_POINT('Origin',(6.82290383517,-39.7742356128,-3.56061176027));
#76157=CARTESIAN_POINT('Origin',(6.82290383517,-39.7742356128,-3.56061176027));
#76158=CARTESIAN_POINT('Origin',(-6.82290383517,-40.1142356128,-3.56061176027));
#76159=CARTESIAN_POINT('',(-4.25781969055053,-39.7742356128,-7.49892908595644));
#76160=CARTESIAN_POINT('',(-11.52290383517,-39.7742356128,-3.56061176027));
#76161=CARTESIAN_POINT('Origin',(-6.82290383517,-39.7742356128,-3.56061176027));
#76162=CARTESIAN_POINT('',(-11.52290383517,-40.1142356128,-3.56061176027));
#76163=CARTESIAN_POINT('',(-9.24345637220266,-39.7742356128,0.468150497498443));
#76164=CARTESIAN_POINT('Origin',(-6.82290383517,-39.7742356128,-3.56061176027));
#76165=CARTESIAN_POINT('',(-7.04639034599947,-39.7742356128,1.1340718008604));
#76166=CARTESIAN_POINT('Origin',(-6.82290383517,-39.7742356128,-3.56061176027));
#76167=CARTESIAN_POINT('',(-6.02437852526,-39.7742356128,1.07105719696));
#76168=CARTESIAN_POINT('Origin',(-6.82290383517,-39.7742356128,-3.56061176027));
#76169=CARTESIAN_POINT('',(-2.12330457313532,-39.7742356128,-3.4993320503742));
#76170=CARTESIAN_POINT('Origin',(-6.82290383517,-39.7742356128,-3.56061176027));
#76171=CARTESIAN_POINT('',(-2.26246783444344,-39.7742356128,-4.69745981422044));
#76172=CARTESIAN_POINT('Origin',(-6.82290383517,-39.7742356128,-3.56061176027));
#76173=CARTESIAN_POINT('Origin',(-6.82290383517,-39.7742356128,-3.56061176027));
#76174=CARTESIAN_POINT('Origin',(-3.35265884719E-30,-40.7742356128,3.15283103411E-22));
#76175=CARTESIAN_POINT('Origin',(0.000416107150126,-37.6642356128,5.42091963994));
#76176=CARTESIAN_POINT('',(2.84060969191E-17,-37.2742356128,11.6643459897));
#76177=CARTESIAN_POINT('',(-6.16208308783,-37.2742356128,4.4189333977));
#76178=CARTESIAN_POINT('Origin',(0.000416107150126,-37.2742356128,5.42091963994));
#76179=CARTESIAN_POINT('',(-1.41472120477E-15,-38.2742356128,11.6643459897));
#76180=CARTESIAN_POINT('',(-1.41472120477E-15,-37.6642356128,11.6643459897));
#76181=CARTESIAN_POINT('',(-6.16208308783,-38.2742356128,4.4189333977));
#76182=CARTESIAN_POINT('Origin',(0.000416107150126,-38.2742356128,5.42091963994));
#76183=CARTESIAN_POINT('',(-6.16208308783,-37.6642356128,4.4189333977));
#76184=CARTESIAN_POINT('Origin',(-6.45819449379,-38.2742356128,4.370787419));
#76185=CARTESIAN_POINT('',(-6.62478636305302,-37.2742356128,4.12129363273029));
#76186=CARTESIAN_POINT('',(-6.62478636278,-38.2742356128,4.12129363314));
#76187=CARTESIAN_POINT('',(-6.62478636278,-38.2742356128,4.12129363314));
#76188=CARTESIAN_POINT('Origin',(-6.45819449379,-37.2742356128,4.370787419));
#76189=CARTESIAN_POINT('Origin',(-6.45819449379,-38.2742356128,4.370787419));
#76190=CARTESIAN_POINT('Ctrl Pts',(-10.3257952821,-38.2742356128,3.01322822759));
#76191=CARTESIAN_POINT('Ctrl Pts',(-10.3257952821,-37.0742356128,3.01322822759));
#76192=CARTESIAN_POINT('Ctrl Pts',(-10.1889067725,-38.2742356128,3.23751153419));
#76193=CARTESIAN_POINT('Ctrl Pts',(-10.1889067725,-37.0742356128,3.23751153419));
#76194=CARTESIAN_POINT('Ctrl Pts',(-10.0345376971,-38.2742356128,3.46376526851));
#76195=CARTESIAN_POINT('Ctrl Pts',(-10.0345376971,-37.0742356128,3.46376526851));
#76196=CARTESIAN_POINT('Ctrl Pts',(-9.84518696085,-38.2742356128,3.7116414664));
#76197=CARTESIAN_POINT('Ctrl Pts',(-9.84518696085,-37.0742356128,3.7116414664));
#76198=CARTESIAN_POINT('Ctrl Pts',(-9.43247784233,-38.2742356128,4.11040580001));
#76199=CARTESIAN_POINT('Ctrl Pts',(-9.43247784233,-37.0742356128,4.11040580001));
#76200=CARTESIAN_POINT('Ctrl Pts',(-8.89477751089,-38.2742356128,4.39069936375));
#76201=CARTESIAN_POINT('Ctrl Pts',(-8.89477751089,-37.0742356128,4.39069936375));
#76202=CARTESIAN_POINT('Ctrl Pts',(-8.65375386005,-38.2742356128,4.47753838835));
#76203=CARTESIAN_POINT('Ctrl Pts',(-8.65375386005,-37.0742356128,4.47753838835));
#76204=CARTESIAN_POINT('Ctrl Pts',(-8.18724170147,-38.2742356128,4.57349385703));
#76205=CARTESIAN_POINT('Ctrl Pts',(-8.18724170147,-37.0742356128,4.57349385703));
#76206=CARTESIAN_POINT('Ctrl Pts',(-7.71488023342,-38.2742356128,4.54915455659));
#76207=CARTESIAN_POINT('Ctrl Pts',(-7.71488023342,-37.0742356128,4.54915455659));
#76208=CARTESIAN_POINT('Ctrl Pts',(-7.50094363126,-38.2742356128,4.51252661069));
#76209=CARTESIAN_POINT('Ctrl Pts',(-7.50094363126,-37.0742356128,4.51252661069));
#76210=CARTESIAN_POINT('Ctrl Pts',(-7.18780951373,-38.2742356128,4.42164672508));
#76211=CARTESIAN_POINT('Ctrl Pts',(-7.18780951373,-37.0742356128,4.42164672508));
#76212=CARTESIAN_POINT('Ctrl Pts',(-6.90087465334,-38.2742356128,4.28688202824));
#76213=CARTESIAN_POINT('Ctrl Pts',(-6.90087465334,-37.0742356128,4.28688202824));
#76214=CARTESIAN_POINT('Ctrl Pts',(-6.80533495241,-38.2742356128,4.23572805208));
#76215=CARTESIAN_POINT('Ctrl Pts',(-6.80533495241,-37.0742356128,4.23572805208));
#76216=CARTESIAN_POINT('Ctrl Pts',(-6.71329436634,-38.2742356128,4.1803921541));
#76217=CARTESIAN_POINT('Ctrl Pts',(-6.71329436634,-37.0742356128,4.1803921541));
#76218=CARTESIAN_POINT('Ctrl Pts',(-6.62478636278,-38.2742356128,4.12129363314));
#76219=CARTESIAN_POINT('Ctrl Pts',(-6.62478636278,-37.0742356128,4.12129363314));
#76220=CARTESIAN_POINT('',(-10.3257952821,-38.2742356128,3.01322822759));
#76221=CARTESIAN_POINT('Ctrl Pts',(-10.3257952821,-38.2742356128,3.01322822759));
#76222=CARTESIAN_POINT('Ctrl Pts',(-10.1889067725,-38.2742356128,3.23751153419));
#76223=CARTESIAN_POINT('Ctrl Pts',(-10.0345376971,-38.2742356128,3.46376526851));
#76224=CARTESIAN_POINT('Ctrl Pts',(-9.84518696085,-38.2742356128,3.7116414664));
#76225=CARTESIAN_POINT('Ctrl Pts',(-9.43247784233,-38.2742356128,4.11040580001));
#76226=CARTESIAN_POINT('Ctrl Pts',(-8.89477751089,-38.2742356128,4.39069936375));
#76227=CARTESIAN_POINT('Ctrl Pts',(-8.65375386005,-38.2742356128,4.47753838835));
#76228=CARTESIAN_POINT('Ctrl Pts',(-8.18724170147,-38.2742356128,4.57349385703));
#76229=CARTESIAN_POINT('Ctrl Pts',(-7.71488023342,-38.2742356128,4.54915455659));
#76230=CARTESIAN_POINT('Ctrl Pts',(-7.50094363126,-38.2742356128,4.51252661069));
#76231=CARTESIAN_POINT('Ctrl Pts',(-7.18780951373,-38.2742356128,4.42164672508));
#76232=CARTESIAN_POINT('Ctrl Pts',(-6.90087465334,-38.2742356128,4.28688202824));
#76233=CARTESIAN_POINT('Ctrl Pts',(-6.80533495241,-38.2742356128,4.23572805208));
#76234=CARTESIAN_POINT('Ctrl Pts',(-6.71329436634,-38.2742356128,4.1803921541));
#76235=CARTESIAN_POINT('Ctrl Pts',(-6.62478636278,-38.2742356128,4.12129363314));
#76236=CARTESIAN_POINT('',(-10.3257952821,-37.2742356128,3.01322822759));
#76237=CARTESIAN_POINT('',(-10.3257952821,-37.6642356128,3.01322822759));
#76238=CARTESIAN_POINT('Ctrl Pts',(-10.3257952821,-37.2742356128,3.01322822759));
#76239=CARTESIAN_POINT('Ctrl Pts',(-10.1889067725,-37.2742356128,3.23751153419));
#76240=CARTESIAN_POINT('Ctrl Pts',(-10.0345376971,-37.2742356128,3.46376526851));
#76241=CARTESIAN_POINT('Ctrl Pts',(-9.84518696085,-37.2742356128,3.7116414664));
#76242=CARTESIAN_POINT('Ctrl Pts',(-9.43247784233,-37.2742356128,4.11040580001));
#76243=CARTESIAN_POINT('Ctrl Pts',(-8.89477751089,-37.2742356128,4.39069936375));
#76244=CARTESIAN_POINT('Ctrl Pts',(-8.65375386005,-37.2742356128,4.47753838835));
#76245=CARTESIAN_POINT('Ctrl Pts',(-8.18724170147,-37.2742356128,4.57349385703));
#76246=CARTESIAN_POINT('Ctrl Pts',(-7.71488023342,-37.2742356128,4.54915455659));
#76247=CARTESIAN_POINT('Ctrl Pts',(-7.50094363126,-37.2742356128,4.51252661069));
#76248=CARTESIAN_POINT('Ctrl Pts',(-7.18780951373,-37.2742356128,4.42164672508));
#76249=CARTESIAN_POINT('Ctrl Pts',(-6.90087465334,-37.2742356128,4.28688202824));
#76250=CARTESIAN_POINT('Ctrl Pts',(-6.80533495241,-37.2742356128,4.23572805208));
#76251=CARTESIAN_POINT('Ctrl Pts',(-6.71329436634,-37.2742356128,4.1803921541));
#76252=CARTESIAN_POINT('Ctrl Pts',(-6.62478636278,-37.2742356128,4.12129363314));
#76253=CARTESIAN_POINT('Ctrl Pts',(-10.3257952821,-38.2742356128,3.01322822759));
#76254=CARTESIAN_POINT('Ctrl Pts',(-10.3257952821,-37.0742356128,3.01322822759));
#76255=CARTESIAN_POINT('Ctrl Pts',(-10.3936895385,-38.2742356128,2.90198771249));
#76256=CARTESIAN_POINT('Ctrl Pts',(-10.3936895385,-37.0742356128,2.90198771249));
#76257=CARTESIAN_POINT('Ctrl Pts',(-10.4633847104,-38.2742356128,2.78112368582));
#76258=CARTESIAN_POINT('Ctrl Pts',(-10.4633847104,-37.0742356128,2.78112368582));
#76259=CARTESIAN_POINT('Ctrl Pts',(-10.529369928,-38.2742356128,2.6551197645));
#76260=CARTESIAN_POINT('Ctrl Pts',(-10.529369928,-37.0742356128,2.6551197645));
#76261=CARTESIAN_POINT('Ctrl Pts',(-10.7481461165,-38.2742356128,2.18905363863));
#76262=CARTESIAN_POINT('Ctrl Pts',(-10.7481461165,-37.0742356128,2.18905363863));
#76263=CARTESIAN_POINT('Ctrl Pts',(-10.8940097918,-38.2742356128,1.69832265276));
#76264=CARTESIAN_POINT('Ctrl Pts',(-10.8940097918,-37.0742356128,1.69832265276));
#76265=CARTESIAN_POINT('Ctrl Pts',(-10.9488467638,-38.2742356128,1.36851337106));
#76266=CARTESIAN_POINT('Ctrl Pts',(-10.9488467638,-37.0742356128,1.36851337106));
#76267=CARTESIAN_POINT('Ctrl Pts',(-10.9986655796,-38.2742356128,1.09670268406));
#76268=CARTESIAN_POINT('Ctrl Pts',(-10.9986655796,-37.0742356128,1.09670268406));
#76269=CARTESIAN_POINT('Ctrl Pts',(-11.0450673741,-38.2742356128,0.800650704934));
#76270=CARTESIAN_POINT('Ctrl Pts',(-11.0450673741,-37.0742356128,0.800650704934));
#76271=CARTESIAN_POINT('',(-11.0450673741,-38.2742356128,0.800650704934));
#76272=CARTESIAN_POINT('',(-11.0450673741,-37.2742356128,0.800650704934));
#76273=CARTESIAN_POINT('',(-11.0450673741,-37.6642356128,0.800650704934));
#76274=CARTESIAN_POINT('Ctrl Pts',(-10.3257952821,-37.2742356128,3.01322822759));
#76275=CARTESIAN_POINT('Ctrl Pts',(-10.3936895385,-37.2742356128,2.90198771249));
#76276=CARTESIAN_POINT('Ctrl Pts',(-10.4633847104,-37.2742356128,2.78112368582));
#76277=CARTESIAN_POINT('Ctrl Pts',(-10.529369928,-37.2742356128,2.6551197645));
#76278=CARTESIAN_POINT('Ctrl Pts',(-10.7481461165,-37.2742356128,2.18905363863));
#76279=CARTESIAN_POINT('Ctrl Pts',(-10.8940097918,-37.2742356128,1.69832265276));
#76280=CARTESIAN_POINT('Ctrl Pts',(-10.9488467638,-37.2742356128,1.36851337106));
#76281=CARTESIAN_POINT('Ctrl Pts',(-10.9986655796,-37.2742356128,1.09670268406));
#76282=CARTESIAN_POINT('Ctrl Pts',(-11.0450673741,-37.2742356128,0.800650704934));
#76283=CARTESIAN_POINT('Ctrl Pts',(-10.3257952821,-38.2742356128,3.01322822759));
#76284=CARTESIAN_POINT('Ctrl Pts',(-10.3936895385,-38.2742356128,2.90198771249));
#76285=CARTESIAN_POINT('Ctrl Pts',(-10.4633847104,-38.2742356128,2.78112368582));
#76286=CARTESIAN_POINT('Ctrl Pts',(-10.529369928,-38.2742356128,2.6551197645));
#76287=CARTESIAN_POINT('Ctrl Pts',(-10.7481461165,-38.2742356128,2.18905363863));
#76288=CARTESIAN_POINT('Ctrl Pts',(-10.8940097918,-38.2742356128,1.69832265276));
#76289=CARTESIAN_POINT('Ctrl Pts',(-10.9488467638,-38.2742356128,1.36851337106));
#76290=CARTESIAN_POINT('Ctrl Pts',(-10.9986655796,-38.2742356128,1.09670268406));
#76291=CARTESIAN_POINT('Ctrl Pts',(-11.0450673741,-38.2742356128,0.800650704934));
#76292=CARTESIAN_POINT('Ctrl Pts',(-1.38699292007,-38.2742356128,-10.1328356959));
#76293=CARTESIAN_POINT('Ctrl Pts',(-1.38699292007,-37.0742356128,-10.1328356959));
#76294=CARTESIAN_POINT('Ctrl Pts',(-1.5965448998,-38.2742356128,-10.1034873192));
#76295=CARTESIAN_POINT('Ctrl Pts',(-1.5965448998,-37.0742356128,-10.1034873192));
#76296=CARTESIAN_POINT('Ctrl Pts',(-1.7801692912,-38.2742356128,-10.0769073631));
#76297=CARTESIAN_POINT('Ctrl Pts',(-1.7801692912,-37.0742356128,-10.0769073631));
#76298=CARTESIAN_POINT('Ctrl Pts',(-1.93876160799,-38.2742356128,-10.0526765385));
#76299=CARTESIAN_POINT('Ctrl Pts',(-1.93876160799,-37.0742356128,-10.0526765385));
#76300=CARTESIAN_POINT('Ctrl Pts',(-2.99097855121,-38.2742356128,-9.87862177772));
#76301=CARTESIAN_POINT('Ctrl Pts',(-2.99097855121,-37.0742356128,-9.87862177772));
#76302=CARTESIAN_POINT('Ctrl Pts',(-4.02327852642,-38.2742356128,-9.59280526012));
#76303=CARTESIAN_POINT('Ctrl Pts',(-4.02327852642,-37.0742356128,-9.59280526012));
#76304=CARTESIAN_POINT('Ctrl Pts',(-4.87817843107,-38.2742356128,-9.25578182833));
#76305=CARTESIAN_POINT('Ctrl Pts',(-4.87817843107,-37.0742356128,-9.25578182833));
#76306=CARTESIAN_POINT('Ctrl Pts',(-6.60543506376,-38.2742356128,-8.36113191267));
#76307=CARTESIAN_POINT('Ctrl Pts',(-6.60543506376,-37.0742356128,-8.36113191267));
#76308=CARTESIAN_POINT('Ctrl Pts',(-8.13232532707,-38.2742356128,-7.15483556723));
#76309=CARTESIAN_POINT('Ctrl Pts',(-8.13232532707,-37.0742356128,-7.15483556723));
#76310=CARTESIAN_POINT('Ctrl Pts',(-8.9654395686,-38.2742356128,-6.4061359759));
#76311=CARTESIAN_POINT('Ctrl Pts',(-8.9654395686,-37.0742356128,-6.4061359759));
#76312=CARTESIAN_POINT('Ctrl Pts',(-10.2944051979,-38.2742356128,-4.9247261457));
#76313=CARTESIAN_POINT('Ctrl Pts',(-10.2944051979,-37.0742356128,-4.9247261457));
#76314=CARTESIAN_POINT('Ctrl Pts',(-11.0595201702,-38.2742356128,-3.0374430354));
#76315=CARTESIAN_POINT('Ctrl Pts',(-11.0595201702,-37.0742356128,-3.0374430354));
#76316=CARTESIAN_POINT('Ctrl Pts',(-11.2122743937,-38.2742356128,-2.16854923298));
#76317=CARTESIAN_POINT('Ctrl Pts',(-11.2122743937,-37.0742356128,-2.16854923298));
#76318=CARTESIAN_POINT('Ctrl Pts',(-11.2441303156,-38.2742356128,-1.03705260495));
#76319=CARTESIAN_POINT('Ctrl Pts',(-11.2441303156,-37.0742356128,-1.03705260495));
#76320=CARTESIAN_POINT('Ctrl Pts',(-11.1482748814,-38.2742356128,0.0384368560119));
#76321=CARTESIAN_POINT('Ctrl Pts',(-11.1482748814,-37.0742356128,0.0384368560119));
#76322=CARTESIAN_POINT('Ctrl Pts',(-11.1189319926,-38.2742356128,0.295374077233));
#76323=CARTESIAN_POINT('Ctrl Pts',(-11.1189319926,-37.0742356128,0.295374077233));
#76324=CARTESIAN_POINT('Ctrl Pts',(-11.0845422068,-38.2742356128,0.548794015622));
#76325=CARTESIAN_POINT('Ctrl Pts',(-11.0845422068,-37.0742356128,0.548794015622));
#76326=CARTESIAN_POINT('Ctrl Pts',(-11.0450673741,-38.2742356128,0.800650704934));
#76327=CARTESIAN_POINT('Ctrl Pts',(-11.0450673741,-37.0742356128,0.800650704934));
#76328=CARTESIAN_POINT('',(-1.3869929218376,-37.2742356128,-10.132835695642));
#76329=CARTESIAN_POINT('Ctrl Pts',(-1.38699292183902,-37.2742356128,-10.1328356956522));
#76330=CARTESIAN_POINT('Ctrl Pts',(-1.59654490104011,-37.2742356128,-10.1034873190205));
#76331=CARTESIAN_POINT('Ctrl Pts',(-1.7801692920033,-37.2742356128,-10.0769073629773));
#76332=CARTESIAN_POINT('Ctrl Pts',(-1.93876160846405,-37.2742356128,-10.0526765384216));
#76333=CARTESIAN_POINT('Ctrl Pts',(-2.99097855144254,-37.2742356128,-9.87862177765562));
#76334=CARTESIAN_POINT('Ctrl Pts',(-4.02327852642,-37.2742356128,-9.59280526012));
#76335=CARTESIAN_POINT('Ctrl Pts',(-4.87817843107,-37.2742356128,-9.25578182833));
#76336=CARTESIAN_POINT('Ctrl Pts',(-6.60543506376,-37.2742356128,-8.36113191267));
#76337=CARTESIAN_POINT('Ctrl Pts',(-8.13232532707,-37.2742356128,-7.15483556723));
#76338=CARTESIAN_POINT('Ctrl Pts',(-8.9654395686,-37.2742356128,-6.4061359759));
#76339=CARTESIAN_POINT('Ctrl Pts',(-10.2944051979,-37.2742356128,-4.9247261457));
#76340=CARTESIAN_POINT('Ctrl Pts',(-11.0595201702,-37.2742356128,-3.0374430354));
#76341=CARTESIAN_POINT('Ctrl Pts',(-11.2122743937,-37.2742356128,-2.16854923298));
#76342=CARTESIAN_POINT('Ctrl Pts',(-11.2441303156,-37.2742356128,-1.03705260495));
#76343=CARTESIAN_POINT('Ctrl Pts',(-11.1482748814,-37.2742356128,0.0384368560119));
#76344=CARTESIAN_POINT('Ctrl Pts',(-11.1189319926,-37.2742356128,0.295374077233));
#76345=CARTESIAN_POINT('Ctrl Pts',(-11.0845422068,-37.2742356128,0.548794015622));
#76346=CARTESIAN_POINT('Ctrl Pts',(-11.0450673741,-37.2742356128,0.800650704934));
#76347=CARTESIAN_POINT('',(-1.38699292008,-38.2742356128,-10.1328356959));
#76348=CARTESIAN_POINT('Ctrl Pts',(-1.38699292007981,-38.2742356128,-10.1328356958986));
#76349=CARTESIAN_POINT('Ctrl Pts',(-1.5965448998,-38.2742356128,-10.1034873192));
#76350=CARTESIAN_POINT('Ctrl Pts',(-1.7801692912,-38.2742356128,-10.0769073631));
#76351=CARTESIAN_POINT('Ctrl Pts',(-1.93876160799,-38.2742356128,-10.0526765385));
#76352=CARTESIAN_POINT('Ctrl Pts',(-2.99097855121,-38.2742356128,-9.87862177772));
#76353=CARTESIAN_POINT('Ctrl Pts',(-4.02327852642,-38.2742356128,-9.59280526012));
#76354=CARTESIAN_POINT('Ctrl Pts',(-4.87817843107,-38.2742356128,-9.25578182833));
#76355=CARTESIAN_POINT('Ctrl Pts',(-6.60543506376,-38.2742356128,-8.36113191267));
#76356=CARTESIAN_POINT('Ctrl Pts',(-8.13232532707,-38.2742356128,-7.15483556723));
#76357=CARTESIAN_POINT('Ctrl Pts',(-8.9654395686,-38.2742356128,-6.4061359759));
#76358=CARTESIAN_POINT('Ctrl Pts',(-10.2944051979,-38.2742356128,-4.9247261457));
#76359=CARTESIAN_POINT('Ctrl Pts',(-11.0595201702,-38.2742356128,-3.0374430354));
#76360=CARTESIAN_POINT('Ctrl Pts',(-11.2122743937,-38.2742356128,-2.16854923298));
#76361=CARTESIAN_POINT('Ctrl Pts',(-11.2441303156,-38.2742356128,-1.03705260495));
#76362=CARTESIAN_POINT('Ctrl Pts',(-11.1482748814,-38.2742356128,0.0384368560119));
#76363=CARTESIAN_POINT('Ctrl Pts',(-11.1189319926,-38.2742356128,0.295374077233));
#76364=CARTESIAN_POINT('Ctrl Pts',(-11.0845422068,-38.2742356128,0.548794015622));
#76365=CARTESIAN_POINT('Ctrl Pts',(-11.0450673741,-38.2742356128,0.800650704934));
#76366=CARTESIAN_POINT('',(-1.38699292008,-37.6642356128,-10.1328356959));
#76367=CARTESIAN_POINT('Origin',(1.35447209004E-14,-38.2742356128,-0.229490269211));
#76368=CARTESIAN_POINT('',(1.3869929218376,-37.2742356128,-10.132835695642));
#76369=CARTESIAN_POINT('Origin',(1.35447209004E-14,-37.2742356128,-0.229490269211));
#76370=CARTESIAN_POINT('',(1.38699292008,-38.2742356128,-10.1328356959));
#76371=CARTESIAN_POINT('Origin',(1.35447209004E-14,-38.2742356128,-0.229490269211));
#76372=CARTESIAN_POINT('',(1.38699292008,-38.2742356128,-10.1328356959));
#76373=CARTESIAN_POINT('Ctrl Pts',(1.38699292007,-38.2742356128,-10.1328356959));
#76374=CARTESIAN_POINT('Ctrl Pts',(1.38699292007,-37.0742356128,-10.1328356959));
#76375=CARTESIAN_POINT('Ctrl Pts',(1.5965448998,-38.2742356128,-10.1034873192));
#76376=CARTESIAN_POINT('Ctrl Pts',(1.5965448998,-37.0742356128,-10.1034873192));
#76377=CARTESIAN_POINT('Ctrl Pts',(1.7801692912,-38.2742356128,-10.0769073631));
#76378=CARTESIAN_POINT('Ctrl Pts',(1.7801692912,-37.0742356128,-10.0769073631));
#76379=CARTESIAN_POINT('Ctrl Pts',(1.93876160799,-38.2742356128,-10.0526765385));
#76380=CARTESIAN_POINT('Ctrl Pts',(1.93876160799,-37.0742356128,-10.0526765385));
#76381=CARTESIAN_POINT('Ctrl Pts',(2.99097855121,-38.2742356128,-9.87862177772));
#76382=CARTESIAN_POINT('Ctrl Pts',(2.99097855121,-37.0742356128,-9.87862177772));
#76383=CARTESIAN_POINT('Ctrl Pts',(4.02327852642,-38.2742356128,-9.59280526012));
#76384=CARTESIAN_POINT('Ctrl Pts',(4.02327852642,-37.0742356128,-9.59280526012));
#76385=CARTESIAN_POINT('Ctrl Pts',(4.87817843107,-38.2742356128,-9.25578182833));
#76386=CARTESIAN_POINT('Ctrl Pts',(4.87817843107,-37.0742356128,-9.25578182833));
#76387=CARTESIAN_POINT('Ctrl Pts',(6.60543506376,-38.2742356128,-8.36113191267));
#76388=CARTESIAN_POINT('Ctrl Pts',(6.60543506376,-37.0742356128,-8.36113191267));
#76389=CARTESIAN_POINT('Ctrl Pts',(8.13232532707,-38.2742356128,-7.15483556723));
#76390=CARTESIAN_POINT('Ctrl Pts',(8.13232532707,-37.0742356128,-7.15483556723));
#76391=CARTESIAN_POINT('Ctrl Pts',(8.9654395686,-38.2742356128,-6.4061359759));
#76392=CARTESIAN_POINT('Ctrl Pts',(8.9654395686,-37.0742356128,-6.4061359759));
#76393=CARTESIAN_POINT('Ctrl Pts',(10.2944051979,-38.2742356128,-4.9247261457));
#76394=CARTESIAN_POINT('Ctrl Pts',(10.2944051979,-37.0742356128,-4.9247261457));
#76395=CARTESIAN_POINT('Ctrl Pts',(11.0595201702,-38.2742356128,-3.0374430354));
#76396=CARTESIAN_POINT('Ctrl Pts',(11.0595201702,-37.0742356128,-3.0374430354));
#76397=CARTESIAN_POINT('Ctrl Pts',(11.2122743937,-38.2742356128,-2.16854923298));
#76398=CARTESIAN_POINT('Ctrl Pts',(11.2122743937,-37.0742356128,-2.16854923298));
#76399=CARTESIAN_POINT('Ctrl Pts',(11.2441303156,-38.2742356128,-1.03705260495));
#76400=CARTESIAN_POINT('Ctrl Pts',(11.2441303156,-37.0742356128,-1.03705260495));
#76401=CARTESIAN_POINT('Ctrl Pts',(11.1482748814,-38.2742356128,0.0384368560119));
#76402=CARTESIAN_POINT('Ctrl Pts',(11.1482748814,-37.0742356128,0.0384368560119));
#76403=CARTESIAN_POINT('Ctrl Pts',(11.1189319926,-38.2742356128,0.295374077233));
#76404=CARTESIAN_POINT('Ctrl Pts',(11.1189319926,-37.0742356128,0.295374077233));
#76405=CARTESIAN_POINT('Ctrl Pts',(11.0845422068,-38.2742356128,0.548794015622));
#76406=CARTESIAN_POINT('Ctrl Pts',(11.0845422068,-37.0742356128,0.548794015622));
#76407=CARTESIAN_POINT('Ctrl Pts',(11.0450673741,-38.2742356128,0.800650704934));
#76408=CARTESIAN_POINT('Ctrl Pts',(11.0450673741,-37.0742356128,0.800650704934));
#76409=CARTESIAN_POINT('',(11.0450673741,-38.2742356128,0.800650704934));
#76410=CARTESIAN_POINT('',(11.0450673741,-37.2742356128,0.800650704934));
#76411=CARTESIAN_POINT('',(11.0450673741,-37.6642356128,0.800650704934));
#76412=CARTESIAN_POINT('Ctrl Pts',(1.38699292183902,-37.2742356128,-10.1328356956522));
#76413=CARTESIAN_POINT('Ctrl Pts',(1.59654490104011,-37.2742356128,-10.1034873190205));
#76414=CARTESIAN_POINT('Ctrl Pts',(1.78016929200329,-37.2742356128,-10.0769073629773));
#76415=CARTESIAN_POINT('Ctrl Pts',(1.93876160846405,-37.2742356128,-10.0526765384216));
#76416=CARTESIAN_POINT('Ctrl Pts',(2.99097855144254,-37.2742356128,-9.87862177765562));
#76417=CARTESIAN_POINT('Ctrl Pts',(4.02327852642,-37.2742356128,-9.59280526012));
#76418=CARTESIAN_POINT('Ctrl Pts',(4.87817843107,-37.2742356128,-9.25578182833));
#76419=CARTESIAN_POINT('Ctrl Pts',(6.60543506376,-37.2742356128,-8.36113191267));
#76420=CARTESIAN_POINT('Ctrl Pts',(8.13232532707,-37.2742356128,-7.15483556723));
#76421=CARTESIAN_POINT('Ctrl Pts',(8.9654395686,-37.2742356128,-6.4061359759));
#76422=CARTESIAN_POINT('Ctrl Pts',(10.2944051979,-37.2742356128,-4.9247261457));
#76423=CARTESIAN_POINT('Ctrl Pts',(11.0595201702,-37.2742356128,-3.0374430354));
#76424=CARTESIAN_POINT('Ctrl Pts',(11.2122743937,-37.2742356128,-2.16854923298));
#76425=CARTESIAN_POINT('Ctrl Pts',(11.2441303156,-37.2742356128,-1.03705260495));
#76426=CARTESIAN_POINT('Ctrl Pts',(11.1482748814,-37.2742356128,0.0384368560119));
#76427=CARTESIAN_POINT('Ctrl Pts',(11.1189319926,-37.2742356128,0.295374077233));
#76428=CARTESIAN_POINT('Ctrl Pts',(11.0845422068,-37.2742356128,0.548794015622));
#76429=CARTESIAN_POINT('Ctrl Pts',(11.0450673741,-37.2742356128,0.800650704934));
#76430=CARTESIAN_POINT('Ctrl Pts',(1.38699292008,-38.2742356128,-10.1328356959));
#76431=CARTESIAN_POINT('Ctrl Pts',(1.5965448998,-38.2742356128,-10.1034873192));
#76432=CARTESIAN_POINT('Ctrl Pts',(1.7801692912,-38.2742356128,-10.0769073631));
#76433=CARTESIAN_POINT('Ctrl Pts',(1.93876160799,-38.2742356128,-10.0526765385));
#76434=CARTESIAN_POINT('Ctrl Pts',(2.99097855121,-38.2742356128,-9.87862177772));
#76435=CARTESIAN_POINT('Ctrl Pts',(4.02327852642,-38.2742356128,-9.59280526012));
#76436=CARTESIAN_POINT('Ctrl Pts',(4.87817843107,-38.2742356128,-9.25578182833));
#76437=CARTESIAN_POINT('Ctrl Pts',(6.60543506376,-38.2742356128,-8.36113191267));
#76438=CARTESIAN_POINT('Ctrl Pts',(8.13232532707,-38.2742356128,-7.15483556723));
#76439=CARTESIAN_POINT('Ctrl Pts',(8.9654395686,-38.2742356128,-6.4061359759));
#76440=CARTESIAN_POINT('Ctrl Pts',(10.2944051979,-38.2742356128,-4.9247261457));
#76441=CARTESIAN_POINT('Ctrl Pts',(11.0595201702,-38.2742356128,-3.0374430354));
#76442=CARTESIAN_POINT('Ctrl Pts',(11.2122743937,-38.2742356128,-2.16854923298));
#76443=CARTESIAN_POINT('Ctrl Pts',(11.2441303156,-38.2742356128,-1.03705260495));
#76444=CARTESIAN_POINT('Ctrl Pts',(11.1482748814,-38.2742356128,0.0384368560119));
#76445=CARTESIAN_POINT('Ctrl Pts',(11.1189319926,-38.2742356128,0.295374077233));
#76446=CARTESIAN_POINT('Ctrl Pts',(11.0845422068,-38.2742356128,0.548794015622));
#76447=CARTESIAN_POINT('Ctrl Pts',(11.0450673741,-38.2742356128,0.800650704934));
#76448=CARTESIAN_POINT('Ctrl Pts',(10.3257952821,-38.2742356128,3.01322822759));
#76449=CARTESIAN_POINT('Ctrl Pts',(10.3257952821,-37.0742356128,3.01322822759));
#76450=CARTESIAN_POINT('Ctrl Pts',(10.3936895385,-38.2742356128,2.90198771249));
#76451=CARTESIAN_POINT('Ctrl Pts',(10.3936895385,-37.0742356128,2.90198771249));
#76452=CARTESIAN_POINT('Ctrl Pts',(10.4633847104,-38.2742356128,2.78112368582));
#76453=CARTESIAN_POINT('Ctrl Pts',(10.4633847104,-37.0742356128,2.78112368582));
#76454=CARTESIAN_POINT('Ctrl Pts',(10.529369928,-38.2742356128,2.6551197645));
#76455=CARTESIAN_POINT('Ctrl Pts',(10.529369928,-37.0742356128,2.6551197645));
#76456=CARTESIAN_POINT('Ctrl Pts',(10.7481461165,-38.2742356128,2.18905363863));
#76457=CARTESIAN_POINT('Ctrl Pts',(10.7481461165,-37.0742356128,2.18905363863));
#76458=CARTESIAN_POINT('Ctrl Pts',(10.8940097918,-38.2742356128,1.69832265276));
#76459=CARTESIAN_POINT('Ctrl Pts',(10.8940097918,-37.0742356128,1.69832265276));
#76460=CARTESIAN_POINT('Ctrl Pts',(10.9488467638,-38.2742356128,1.36851337106));
#76461=CARTESIAN_POINT('Ctrl Pts',(10.9488467638,-37.0742356128,1.36851337106));
#76462=CARTESIAN_POINT('Ctrl Pts',(10.9986655796,-38.2742356128,1.09670268406));
#76463=CARTESIAN_POINT('Ctrl Pts',(10.9986655796,-37.0742356128,1.09670268406));
#76464=CARTESIAN_POINT('Ctrl Pts',(11.0450673741,-38.2742356128,0.800650704934));
#76465=CARTESIAN_POINT('Ctrl Pts',(11.0450673741,-37.0742356128,0.800650704934));
#76466=CARTESIAN_POINT('',(10.3257952821,-37.2742356128,3.01322822759));
#76467=CARTESIAN_POINT('Ctrl Pts',(10.3257952821,-37.2742356128,3.01322822759));
#76468=CARTESIAN_POINT('Ctrl Pts',(10.3936895385,-37.2742356128,2.90198771249));
#76469=CARTESIAN_POINT('Ctrl Pts',(10.4633847104,-37.2742356128,2.78112368582));
#76470=CARTESIAN_POINT('Ctrl Pts',(10.529369928,-37.2742356128,2.6551197645));
#76471=CARTESIAN_POINT('Ctrl Pts',(10.7481461165,-37.2742356128,2.18905363863));
#76472=CARTESIAN_POINT('Ctrl Pts',(10.8940097918,-37.2742356128,1.69832265276));
#76473=CARTESIAN_POINT('Ctrl Pts',(10.9488467638,-37.2742356128,1.36851337106));
#76474=CARTESIAN_POINT('Ctrl Pts',(10.9986655796,-37.2742356128,1.09670268406));
#76475=CARTESIAN_POINT('Ctrl Pts',(11.0450673741,-37.2742356128,0.800650704934));
#76476=CARTESIAN_POINT('',(10.3257952821,-38.2742356128,3.01322822759));
#76477=CARTESIAN_POINT('Ctrl Pts',(10.3257952821,-38.2742356128,3.01322822759));
#76478=CARTESIAN_POINT('Ctrl Pts',(10.3936895385,-38.2742356128,2.90198771249));
#76479=CARTESIAN_POINT('Ctrl Pts',(10.4633847104,-38.2742356128,2.78112368582));
#76480=CARTESIAN_POINT('Ctrl Pts',(10.529369928,-38.2742356128,2.6551197645));
#76481=CARTESIAN_POINT('Ctrl Pts',(10.7481461165,-38.2742356128,2.18905363863));
#76482=CARTESIAN_POINT('Ctrl Pts',(10.8940097918,-38.2742356128,1.69832265276));
#76483=CARTESIAN_POINT('Ctrl Pts',(10.9488467638,-38.2742356128,1.36851337106));
#76484=CARTESIAN_POINT('Ctrl Pts',(10.9986655796,-38.2742356128,1.09670268406));
#76485=CARTESIAN_POINT('Ctrl Pts',(11.0450673741,-38.2742356128,0.800650704934));
#76486=CARTESIAN_POINT('',(10.3257952821,-37.6642356128,3.01322822759));
#76487=CARTESIAN_POINT('Ctrl Pts',(10.3257952821,-38.2742356128,3.01322822759));
#76488=CARTESIAN_POINT('Ctrl Pts',(10.3257952821,-37.0742356128,3.01322822759));
#76489=CARTESIAN_POINT('Ctrl Pts',(10.1889067725,-38.2742356128,3.23751153419));
#76490=CARTESIAN_POINT('Ctrl Pts',(10.1889067725,-37.0742356128,3.23751153419));
#76491=CARTESIAN_POINT('Ctrl Pts',(10.0345376971,-38.2742356128,3.46376526851));
#76492=CARTESIAN_POINT('Ctrl Pts',(10.0345376971,-37.0742356128,3.46376526851));
#76493=CARTESIAN_POINT('Ctrl Pts',(9.84518696085,-38.2742356128,3.7116414664));
#76494=CARTESIAN_POINT('Ctrl Pts',(9.84518696085,-37.0742356128,3.7116414664));
#76495=CARTESIAN_POINT('Ctrl Pts',(9.43247784233,-38.2742356128,4.11040580001));
#76496=CARTESIAN_POINT('Ctrl Pts',(9.43247784233,-37.0742356128,4.11040580001));
#76497=CARTESIAN_POINT('Ctrl Pts',(8.89477751089,-38.2742356128,4.39069936375));
#76498=CARTESIAN_POINT('Ctrl Pts',(8.89477751089,-37.0742356128,4.39069936375));
#76499=CARTESIAN_POINT('Ctrl Pts',(8.65375386005,-38.2742356128,4.47753838835));
#76500=CARTESIAN_POINT('Ctrl Pts',(8.65375386005,-37.0742356128,4.47753838835));
#76501=CARTESIAN_POINT('Ctrl Pts',(8.18724170147,-38.2742356128,4.57349385703));
#76502=CARTESIAN_POINT('Ctrl Pts',(8.18724170147,-37.0742356128,4.57349385703));
#76503=CARTESIAN_POINT('Ctrl Pts',(7.71488023342,-38.2742356128,4.54915455659));
#76504=CARTESIAN_POINT('Ctrl Pts',(7.71488023342,-37.0742356128,4.54915455659));
#76505=CARTESIAN_POINT('Ctrl Pts',(7.50094363126,-38.2742356128,4.51252661069));
#76506=CARTESIAN_POINT('Ctrl Pts',(7.50094363126,-37.0742356128,4.51252661069));
#76507=CARTESIAN_POINT('Ctrl Pts',(7.18780951373,-38.2742356128,4.42164672508));
#76508=CARTESIAN_POINT('Ctrl Pts',(7.18780951373,-37.0742356128,4.42164672508));
#76509=CARTESIAN_POINT('Ctrl Pts',(6.90087465334,-38.2742356128,4.28688202824));
#76510=CARTESIAN_POINT('Ctrl Pts',(6.90087465334,-37.0742356128,4.28688202824));
#76511=CARTESIAN_POINT('Ctrl Pts',(6.80533495241,-38.2742356128,4.23572805208));
#76512=CARTESIAN_POINT('Ctrl Pts',(6.80533495241,-37.0742356128,4.23572805208));
#76513=CARTESIAN_POINT('Ctrl Pts',(6.71329436634,-38.2742356128,4.1803921541));
#76514=CARTESIAN_POINT('Ctrl Pts',(6.71329436634,-37.0742356128,4.1803921541));
#76515=CARTESIAN_POINT('Ctrl Pts',(6.62478636278,-38.2742356128,4.12129363314));
#76516=CARTESIAN_POINT('Ctrl Pts',(6.62478636278,-37.0742356128,4.12129363314));
#76517=CARTESIAN_POINT('',(6.62478636278,-38.2742356128,4.12129363314));
#76518=CARTESIAN_POINT('',(6.62478636305302,-37.2742356128,4.12129363273029));
#76519=CARTESIAN_POINT('',(6.62478636278,-37.6642356128,4.12129363314));
#76520=CARTESIAN_POINT('Ctrl Pts',(10.3257952821,-37.2742356128,3.01322822759));
#76521=CARTESIAN_POINT('Ctrl Pts',(10.1889067725,-37.2742356128,3.23751153419));
#76522=CARTESIAN_POINT('Ctrl Pts',(10.0345376971,-37.2742356128,3.46376526851));
#76523=CARTESIAN_POINT('Ctrl Pts',(9.84518696085,-37.2742356128,3.7116414664));
#76524=CARTESIAN_POINT('Ctrl Pts',(9.43247784233,-37.2742356128,4.11040580001));
#76525=CARTESIAN_POINT('Ctrl Pts',(8.89477751089,-37.2742356128,4.39069936375));
#76526=CARTESIAN_POINT('Ctrl Pts',(8.65375386005,-37.2742356128,4.47753838835));
#76527=CARTESIAN_POINT('Ctrl Pts',(8.18724170147,-37.2742356128,4.57349385703));
#76528=CARTESIAN_POINT('Ctrl Pts',(7.71488023342,-37.2742356128,4.54915455659));
#76529=CARTESIAN_POINT('Ctrl Pts',(7.50094363126,-37.2742356128,4.51252661069));
#76530=CARTESIAN_POINT('Ctrl Pts',(7.18780951373,-37.2742356128,4.42164672508));
#76531=CARTESIAN_POINT('Ctrl Pts',(6.90087465334,-37.2742356128,4.28688202824));
#76532=CARTESIAN_POINT('Ctrl Pts',(6.80533495241,-37.2742356128,4.23572805208));
#76533=CARTESIAN_POINT('Ctrl Pts',(6.71329436634,-37.2742356128,4.1803921541));
#76534=CARTESIAN_POINT('Ctrl Pts',(6.62478636278,-37.2742356128,4.12129363314));
#76535=CARTESIAN_POINT('Ctrl Pts',(10.3257952821,-38.2742356128,3.01322822759));
#76536=CARTESIAN_POINT('Ctrl Pts',(10.1889067725,-38.2742356128,3.23751153419));
#76537=CARTESIAN_POINT('Ctrl Pts',(10.0345376971,-38.2742356128,3.46376526851));
#76538=CARTESIAN_POINT('Ctrl Pts',(9.84518696085,-38.2742356128,3.7116414664));
#76539=CARTESIAN_POINT('Ctrl Pts',(9.43247784233,-38.2742356128,4.11040580001));
#76540=CARTESIAN_POINT('Ctrl Pts',(8.89477751089,-38.2742356128,4.39069936375));
#76541=CARTESIAN_POINT('Ctrl Pts',(8.65375386005,-38.2742356128,4.47753838835));
#76542=CARTESIAN_POINT('Ctrl Pts',(8.18724170147,-38.2742356128,4.57349385703));
#76543=CARTESIAN_POINT('Ctrl Pts',(7.71488023342,-38.2742356128,4.54915455659));
#76544=CARTESIAN_POINT('Ctrl Pts',(7.50094363126,-38.2742356128,4.51252661069));
#76545=CARTESIAN_POINT('Ctrl Pts',(7.18780951373,-38.2742356128,4.42164672508));
#76546=CARTESIAN_POINT('Ctrl Pts',(6.90087465334,-38.2742356128,4.28688202824));
#76547=CARTESIAN_POINT('Ctrl Pts',(6.80533495241,-38.2742356128,4.23572805208));
#76548=CARTESIAN_POINT('Ctrl Pts',(6.71329436634,-38.2742356128,4.1803921541));
#76549=CARTESIAN_POINT('Ctrl Pts',(6.62478636278,-38.2742356128,4.12129363314));
#76550=CARTESIAN_POINT('Origin',(6.45819449379,-38.2742356128,4.370787419));
#76551=CARTESIAN_POINT('',(6.16208308783,-38.2742356128,4.4189333977));
#76552=CARTESIAN_POINT('',(6.16208308783,-37.2742356128,4.4189333977));
#76553=CARTESIAN_POINT('',(6.16208308783,-38.2742356128,4.4189333977));
#76554=CARTESIAN_POINT('Origin',(6.45819449379,-37.2742356128,4.370787419));
#76555=CARTESIAN_POINT('Origin',(6.45819449379,-38.2742356128,4.370787419));
#76556=CARTESIAN_POINT('Origin',(-0.000416107150126,-37.6642356128,5.42091963994));
#76557=CARTESIAN_POINT('Origin',(-0.000416107150126,-37.2742356128,5.42091963994));
#76558=CARTESIAN_POINT('Origin',(-0.000416107150126,-38.2742356128,5.42091963994));
#76559=CARTESIAN_POINT('Origin',(-3.35265884719E-30,-39.7742356128,3.15283103411E-22));
#76560=CARTESIAN_POINT('',(-9.36455599938E-5,-39.7742356128,10.8643459797));
#76561=CARTESIAN_POINT('Origin',(0.0108494330597224,-39.7742356128,5.39376217080941));
#76562=CARTESIAN_POINT('Origin',(-0.0118852773128557,-39.7742356128,5.39166608075836));
#76563=CARTESIAN_POINT('Origin',(-3.35265884719E-30,-39.7742356128,3.15283103411E-22));
#76564=CARTESIAN_POINT('',(-4.44050669832,-39.7742356128,5.57005878528));
#76565=CARTESIAN_POINT('Ctrl Pts',(-4.44050669832,-39.7742356128,5.57005878528));
#76566=CARTESIAN_POINT('Ctrl Pts',(-4.44147453346363,-39.7742356128,5.54123951619091));
#76567=CARTESIAN_POINT('Ctrl Pts',(-4.44231065914721,-39.7742356128,5.51241582391387));
#76568=CARTESIAN_POINT('Ctrl Pts',(-4.44299515202408,-39.7742356128,5.48359182392916));
#76569=CARTESIAN_POINT('Ctrl Pts',(-4.44351074301195,-39.7742356128,5.45477116963976));
#76570=CARTESIAN_POINT('Ctrl Pts',(-4.4438425928504,-39.7742356128,5.42595709132));
#76571=CARTESIAN_POINT('',(3.98812927127E-15,-39.7742356128,9.86434598407));
#76572=CARTESIAN_POINT('Origin',(0.000416107150120569,-39.7742356128,5.42091963994));
#76573=CARTESIAN_POINT('',(4.44050669832,-39.7742356128,5.57005878528));
#76574=CARTESIAN_POINT('Origin',(-0.000416107150128624,-39.7742356128,5.42091963994));
#76575=CARTESIAN_POINT('Ctrl Pts',(4.44050669832,-39.7742356128,5.57005878528));
#76576=CARTESIAN_POINT('Ctrl Pts',(4.44147453346363,-39.7742356128,5.54123951619091));
#76577=CARTESIAN_POINT('Ctrl Pts',(4.44231065914721,-39.7742356128,5.51241582391387));
#76578=CARTESIAN_POINT('Ctrl Pts',(4.44299515202408,-39.7742356128,5.48359182392916));
#76579=CARTESIAN_POINT('Ctrl Pts',(4.44351074301195,-39.7742356128,5.45477116963976));
#76580=CARTESIAN_POINT('Ctrl Pts',(4.4438425928504,-39.7742356128,5.42595709132));
#76581=CARTESIAN_POINT('Origin',(-3.35265884719E-30,-39.7742356128,3.15283103411E-22));
#76582=CARTESIAN_POINT('Ctrl Pts',(4.44384282525284,-39.7742356128,5.30375137006997));
#76583=CARTESIAN_POINT('Ctrl Pts',(4.43847639264561,-39.7742356128,4.86276818888142));
#76584=CARTESIAN_POINT('Ctrl Pts',(4.3822968816921,-39.7742356128,4.42505108085605));
#76585=CARTESIAN_POINT('Ctrl Pts',(4.23617161309801,-39.7742356128,3.99973909354992));
#76586=CARTESIAN_POINT('Ctrl Pts',(4.084425172493,-39.7742356128,3.57446610480042));
#76587=CARTESIAN_POINT('Ctrl Pts',(3.94523376325647,-39.7742356128,3.14826407381826));
#76588=CARTESIAN_POINT('Ctrl Pts',(4.44050669832,-39.7742356128,5.57005878528));
#76589=CARTESIAN_POINT('Ctrl Pts',(4.44050669832,-36.7742356128,5.57005878528));
#76590=CARTESIAN_POINT('Ctrl Pts',(4.46448048797,-39.7742356128,4.85619021008));
#76591=CARTESIAN_POINT('Ctrl Pts',(4.46448048797,-36.7742356128,4.85619021008));
#76592=CARTESIAN_POINT('Ctrl Pts',(4.40764009695,-39.7742356128,4.1396076589));
#76593=CARTESIAN_POINT('Ctrl Pts',(4.40764009695,-36.7742356128,4.1396076589));
#76594=CARTESIAN_POINT('Ctrl Pts',(3.96717692929,-39.7742356128,3.48286100495));
#76595=CARTESIAN_POINT('Ctrl Pts',(3.96717692929,-36.7742356128,3.48286100495));
#76596=CARTESIAN_POINT('Ctrl Pts',(3.83955824331,-39.7742356128,2.77453753392));
#76597=CARTESIAN_POINT('Ctrl Pts',(3.83955824331,-36.7742356128,2.77453753392));
#76598=CARTESIAN_POINT('Ctrl Pts',(3.62746705121,-39.7742356128,2.09248151608));
#76599=CARTESIAN_POINT('Ctrl Pts',(3.62746705121,-36.7742356128,2.09248151608));
#76600=CARTESIAN_POINT('',(4.44050669832,-37.2742356128,5.57005878528));
#76601=CARTESIAN_POINT('',(3.62746705121,-37.2742356128,2.09248151608));
#76602=CARTESIAN_POINT('Ctrl Pts',(4.44050669832,-37.2742356128,5.57005878528));
#76603=CARTESIAN_POINT('Ctrl Pts',(4.46448048797,-37.2742356128,4.85619021008));
#76604=CARTESIAN_POINT('Ctrl Pts',(4.40764009695,-37.2742356128,4.1396076589));
#76605=CARTESIAN_POINT('Ctrl Pts',(3.96717692929,-37.2742356128,3.48286100495));
#76606=CARTESIAN_POINT('Ctrl Pts',(3.83955824331,-37.2742356128,2.77453753392));
#76607=CARTESIAN_POINT('Ctrl Pts',(3.62746705121,-37.2742356128,2.09248151608));
#76608=CARTESIAN_POINT('',(3.62746705121,-39.7742356128,2.09248151608));
#76609=CARTESIAN_POINT('',(3.62746705121,-39.6642356128,2.09248151608));
#76610=CARTESIAN_POINT('Ctrl Pts',(3.94523376325647,-39.7742356128,3.14826407381826));
#76611=CARTESIAN_POINT('Ctrl Pts',(3.87620988630884,-39.7742356128,2.93691398617489));
#76612=CARTESIAN_POINT('Ctrl Pts',(3.81027340038231,-39.7742356128,2.72533543899502));
#76613=CARTESIAN_POINT('Ctrl Pts',(3.74964078603135,-39.7742356128,2.5134103854269));
#76614=CARTESIAN_POINT('Ctrl Pts',(3.69252846020896,-39.7742356128,2.30171003282089));
#76615=CARTESIAN_POINT('Ctrl Pts',(3.62746705121,-39.7742356128,2.09248151608));
#76616=CARTESIAN_POINT('',(4.44050669832,-39.6642356128,5.57005878528));
#76617=CARTESIAN_POINT('Origin',(-3.35265884719E-30,-39.7742356128,3.15283103411E-22));
#76618=CARTESIAN_POINT('',(0.772076508426,-39.7742356128,-1.09035382089));
#76619=CARTESIAN_POINT('Ctrl Pts',(0.772076508426,-39.7742356128,-1.09035382089));
#76620=CARTESIAN_POINT('Ctrl Pts',(0.886178610516,-39.7742356128,-1.05996501737));
#76621=CARTESIAN_POINT('Ctrl Pts',(0.999471783383,-39.7742356128,-1.02648938573));
#76622=CARTESIAN_POINT('Ctrl Pts',(1.28376436686776,-39.7742356128,-0.933262719920861));
#76623=CARTESIAN_POINT('Ctrl Pts',(1.55846384573443,-39.7742356128,-0.816903495533422));
#76624=CARTESIAN_POINT('Ctrl Pts',(1.99336348977486,-39.7742356128,-0.570669430159104));
#76625=CARTESIAN_POINT('Ctrl Pts',(2.3976244972855,-39.7742356128,-0.230794401633491));
#76626=CARTESIAN_POINT('Ctrl Pts',(2.71790928753969,-39.7742356128,0.199910378054401));
#76627=CARTESIAN_POINT('Ctrl Pts',(3.04613205154736,-39.7742356128,0.706586155851523));
#76628=CARTESIAN_POINT('Ctrl Pts',(3.3135563642201,-39.7742356128,1.24160867153818));
#76629=CARTESIAN_POINT('Ctrl Pts',(3.46527948246,-39.7742356128,1.60915269898));
#76630=CARTESIAN_POINT('Ctrl Pts',(3.55147728822,-39.7742356128,1.84810892036));
#76631=CARTESIAN_POINT('Ctrl Pts',(3.62746705121,-39.7742356128,2.09248151608));
#76632=CARTESIAN_POINT('',(-0.772076508426,-39.7742356128,-1.09035382089));
#76633=CARTESIAN_POINT('Origin',(-3.57491813929E-14,-39.7742356128,1.80859389597));
#76634=CARTESIAN_POINT('',(-3.62746705121,-39.7742356128,2.09248151608));
#76635=CARTESIAN_POINT('Ctrl Pts',(-0.772076508424,-39.7742356128,-1.09035382089));
#76636=CARTESIAN_POINT('Ctrl Pts',(-0.886178610516,-39.7742356128,-1.05996501737));
#76637=CARTESIAN_POINT('Ctrl Pts',(-0.999471783383,-39.7742356128,-1.02648938573));
#76638=CARTESIAN_POINT('Ctrl Pts',(-1.11165616418,-39.7742356128,-0.989701314619));
#76639=CARTESIAN_POINT('Ctrl Pts',(-1.3921632233,-39.7742356128,-0.887346335547));
#76640=CARTESIAN_POINT('Ctrl Pts',(-1.65990259641,-39.7742356128,-0.759470300753));
#76641=CARTESIAN_POINT('Ctrl Pts',(-1.81552533939,-39.7742356128,-0.67135889116));
#76642=CARTESIAN_POINT('Ctrl Pts',(-2.13001246648,-39.7742356128,-0.455784308931));
#76643=CARTESIAN_POINT('Ctrl Pts',(-2.40225756964,-39.7742356128,-0.187376365848));
#76644=CARTESIAN_POINT('Ctrl Pts',(-2.53491876149,-39.7742356128,-0.0306790811922));
#76645=CARTESIAN_POINT('Ctrl Pts',(-2.74588721076,-39.7742356128,0.250416153254));
#76646=CARTESIAN_POINT('Ctrl Pts',(-2.93290680803,-39.7742356128,0.545770364295));
#76647=CARTESIAN_POINT('Ctrl Pts',(-3.00715366555,-39.7742356128,0.670355528577));
#76648=CARTESIAN_POINT('Ctrl Pts',(-3.20108514097,-39.7742356128,1.0165930916));
#76649=CARTESIAN_POINT('Ctrl Pts',(-3.36887363395,-39.7742356128,1.37561285195));
#76650=CARTESIAN_POINT('Ctrl Pts',(-3.46527948246,-39.7742356128,1.60915269898));
#76651=CARTESIAN_POINT('Ctrl Pts',(-3.55147728822,-39.7742356128,1.84810892036));
#76652=CARTESIAN_POINT('Ctrl Pts',(-3.62746705121,-39.7742356128,2.09248151608));
#76653=CARTESIAN_POINT('Ctrl Pts',(-3.94523376325647,-39.7742356128,3.14826407381827));
#76654=CARTESIAN_POINT('Ctrl Pts',(-3.87620988630884,-39.7742356128,2.9369139861749));
#76655=CARTESIAN_POINT('Ctrl Pts',(-3.81027340038232,-39.7742356128,2.72533543899502));
#76656=CARTESIAN_POINT('Ctrl Pts',(-3.74964078603135,-39.7742356128,2.5134103854269));
#76657=CARTESIAN_POINT('Ctrl Pts',(-3.69252846020896,-39.7742356128,2.30171003282089));
#76658=CARTESIAN_POINT('Ctrl Pts',(-3.62746705121,-39.7742356128,2.09248151608));
#76659=CARTESIAN_POINT('Origin',(-3.35265884719E-30,-39.7742356128,3.15283103411E-22));
#76660=CARTESIAN_POINT('Ctrl Pts',(-4.44384282525284,-39.7742356128,5.30375137006997));
#76661=CARTESIAN_POINT('Ctrl Pts',(-4.43847639264561,-39.7742356128,4.86276818888142));
#76662=CARTESIAN_POINT('Ctrl Pts',(-4.3822968816921,-39.7742356128,4.42505108085606));
#76663=CARTESIAN_POINT('Ctrl Pts',(-4.23617161309801,-39.7742356128,3.99973909354993));
#76664=CARTESIAN_POINT('Ctrl Pts',(-4.084425172493,-39.7742356128,3.57446610480043));
#76665=CARTESIAN_POINT('Ctrl Pts',(-3.94523376325647,-39.7742356128,3.14826407381827));
#76666=CARTESIAN_POINT('Ctrl Pts',(-4.44050669832,-39.7742356128,5.57005878528));
#76667=CARTESIAN_POINT('Ctrl Pts',(-4.44050669832,-36.7742356128,5.57005878528));
#76668=CARTESIAN_POINT('Ctrl Pts',(-4.46448048797,-39.7742356128,4.85619021008));
#76669=CARTESIAN_POINT('Ctrl Pts',(-4.46448048797,-36.7742356128,4.85619021008));
#76670=CARTESIAN_POINT('Ctrl Pts',(-4.40764009695,-39.7742356128,4.1396076589));
#76671=CARTESIAN_POINT('Ctrl Pts',(-4.40764009695,-36.7742356128,4.1396076589));
#76672=CARTESIAN_POINT('Ctrl Pts',(-3.96717692929,-39.7742356128,3.48286100495));
#76673=CARTESIAN_POINT('Ctrl Pts',(-3.96717692929,-36.7742356128,3.48286100495));
#76674=CARTESIAN_POINT('Ctrl Pts',(-3.83955824331,-39.7742356128,2.77453753392));
#76675=CARTESIAN_POINT('Ctrl Pts',(-3.83955824331,-36.7742356128,2.77453753392));
#76676=CARTESIAN_POINT('Ctrl Pts',(-3.62746705121,-39.7742356128,2.09248151608));
#76677=CARTESIAN_POINT('Ctrl Pts',(-3.62746705121,-36.7742356128,2.09248151608));
#76678=CARTESIAN_POINT('',(-4.44050669832,-37.2742356128,5.57005878528));
#76679=CARTESIAN_POINT('',(-4.44050669832,-39.6642356128,5.57005878528));
#76680=CARTESIAN_POINT('',(-3.62746705121,-37.2742356128,2.09248151608));
#76681=CARTESIAN_POINT('',(-3.62746705121,-39.6642356128,2.09248151608));
#76682=CARTESIAN_POINT('Ctrl Pts',(-4.44050669832,-37.2742356128,5.57005878528));
#76683=CARTESIAN_POINT('Ctrl Pts',(-4.46448048797,-37.2742356128,4.85619021008));
#76684=CARTESIAN_POINT('Ctrl Pts',(-4.40764009695,-37.2742356128,4.1396076589));
#76685=CARTESIAN_POINT('Ctrl Pts',(-3.96717692929,-37.2742356128,3.48286100495));
#76686=CARTESIAN_POINT('Ctrl Pts',(-3.83955824331,-37.2742356128,2.77453753392));
#76687=CARTESIAN_POINT('Ctrl Pts',(-3.62746705121,-37.2742356128,2.09248151608));
#76688=CARTESIAN_POINT('Origin',(-3.35265884719E-30,-39.7742356128,3.15283103411E-22));
#76689=CARTESIAN_POINT('',(3.51985615629,-39.7742356128,-3.20601908088));
#76690=CARTESIAN_POINT('Origin',(-1143.38887689168,-39.774235612772,1093.0893729638));
#76691=CARTESIAN_POINT('',(3.67755401867,-39.7742356128,-3.05915055738));
#76692=CARTESIAN_POINT('Origin',(3.78952269078,-39.7742356128,-3.33747234321));
#76693=CARTESIAN_POINT('Ctrl Pts',(7.04639034878034,-39.7742356128,1.13407180047521));
#76694=CARTESIAN_POINT('Ctrl Pts',(6.98577032985781,-39.7742356128,0.696425342316252));
#76695=CARTESIAN_POINT('Ctrl Pts',(6.89012094467166,-39.7742356128,0.272653387012416));
#76696=CARTESIAN_POINT('Ctrl Pts',(6.75651149488734,-39.7742356128,-0.133493132432014));
#76697=CARTESIAN_POINT('Ctrl Pts',(6.39374256643522,-39.7742356128,-0.93640428199725));
#76698=CARTESIAN_POINT('Ctrl Pts',(5.86106085412,-39.7742356128,-1.62790491519));
#76699=CARTESIAN_POINT('Ctrl Pts',(5.53842443335,-39.7742356128,-1.95360958375));
#76700=CARTESIAN_POINT('Ctrl Pts',(4.98933040959,-39.7742356128,-2.39194593497));
#76701=CARTESIAN_POINT('Ctrl Pts',(4.36273333629,-39.7742356128,-2.74903878258));
#76702=CARTESIAN_POINT('Ctrl Pts',(4.14078300625,-39.7742356128,-2.86156599489));
#76703=CARTESIAN_POINT('Ctrl Pts',(3.91246466012,-39.7742356128,-2.96464616022));
#76704=CARTESIAN_POINT('Ctrl Pts',(3.67755401867,-39.7742356128,-3.05915055738));
#76705=CARTESIAN_POINT('',(3.30432511166,-39.7742356128,-2.13141127128));
#76706=CARTESIAN_POINT('Ctrl Pts',(6.02437852526,-39.7742356128,1.07105719697));
#76707=CARTESIAN_POINT('Ctrl Pts',(5.86422039559,-39.7742356128,0.163050845024));
#76708=CARTESIAN_POINT('Ctrl Pts',(5.51798981241,-39.7742356128,-0.6356582873));
#76709=CARTESIAN_POINT('Ctrl Pts',(4.97390737876,-39.7742356128,-1.26910580103));
#76710=CARTESIAN_POINT('Ctrl Pts',(4.20012016579,-39.7742356128,-1.77103350786));
#76711=CARTESIAN_POINT('Ctrl Pts',(3.30432511166,-39.7742356128,-2.13141127128));
#76712=CARTESIAN_POINT('',(2.62096770799,-39.7742356128,-2.76784153979));
#76713=CARTESIAN_POINT('Origin',(3.57176864033797,-39.7742356128,-3.1036622151543));
#76714=CARTESIAN_POINT('Ctrl Pts',(2.62096770799,-39.7742356128,-2.76784153979));
#76715=CARTESIAN_POINT('Ctrl Pts',(2.48674506753,-39.7742356128,-3.04318924635));
#76716=CARTESIAN_POINT('Ctrl Pts',(2.32123277945,-39.7742356128,-3.28726285739));
#76717=CARTESIAN_POINT('Ctrl Pts',(2.12330703536,-39.7742356128,-3.49933208248));
#76718=CARTESIAN_POINT('Origin',(-3.35265884719E-30,-39.7742356128,3.15283103411E-22));
#76719=CARTESIAN_POINT('Origin',(-3.35265884719E-30,-39.7742356128,3.15283103411E-22));
#76720=CARTESIAN_POINT('',(7.07911993306,-39.7742356128,1.41233341424));
#76721=CARTESIAN_POINT('Ctrl Pts',(7.07911993306,-39.7742356128,1.41233341424));
#76722=CARTESIAN_POINT('Ctrl Pts',(7.07459783011676,-39.7742356128,1.36585334327933));
#76723=CARTESIAN_POINT('Ctrl Pts',(7.06961906998812,-39.7742356128,1.31941671396487));
#76724=CARTESIAN_POINT('Ctrl Pts',(7.05871909787096,-39.7742356128,1.22665564708758));
#76725=CARTESIAN_POINT('Ctrl Pts',(7.05279772717288,-39.7742356128,1.18032989304728));
#76726=CARTESIAN_POINT('Ctrl Pts',(7.04639034822407,-39.7742356128,1.1340717964593));
#76727=CARTESIAN_POINT('',(7.21384189758,-39.7742356128,2.18958432614));
#76728=CARTESIAN_POINT('Ctrl Pts',(7.21384189758,-39.7742356128,2.18958432614));
#76729=CARTESIAN_POINT('Ctrl Pts',(7.13908599018,-39.7742356128,2.05065155888));
#76730=CARTESIAN_POINT('Ctrl Pts',(7.08905059141,-39.7742356128,1.8984189694));
#76731=CARTESIAN_POINT('Ctrl Pts',(7.1053290044,-39.7742356128,1.72681022597));
#76732=CARTESIAN_POINT('Ctrl Pts',(7.09439724612,-39.7742356128,1.56936004643));
#76733=CARTESIAN_POINT('Ctrl Pts',(7.07911993306,-39.7742356128,1.41233341424));
#76734=CARTESIAN_POINT('',(8.75956299023,-39.7742356128,2.0634404101));
#76735=CARTESIAN_POINT('Ctrl Pts',(8.75956299023,-39.7742356128,2.0634404101));
#76736=CARTESIAN_POINT('Ctrl Pts',(8.67258032609,-39.7742356128,2.20595609378));
#76737=CARTESIAN_POINT('Ctrl Pts',(8.57679326147,-39.7742356128,2.34786591099));
#76738=CARTESIAN_POINT('Ctrl Pts',(8.46448329596,-39.7742356128,2.49604426586));
#76739=CARTESIAN_POINT('Ctrl Pts',(8.27825186329,-39.7742356128,2.67220081215));
#76740=CARTESIAN_POINT('Ctrl Pts',(8.05379939761,-39.7742356128,2.74035894609));
#76741=CARTESIAN_POINT('Ctrl Pts',(7.9779370982,-39.7742356128,2.74765496713));
#76742=CARTESIAN_POINT('Ctrl Pts',(7.82203636779,-39.7742356128,2.73225108729));
#76743=CARTESIAN_POINT('Ctrl Pts',(7.67278421879,-39.7742356128,2.66639360485));
#76744=CARTESIAN_POINT('Ctrl Pts',(7.59903734004,-39.7742356128,2.62164000818));
#76745=CARTESIAN_POINT('Ctrl Pts',(7.46503014366,-39.7742356128,2.52047218586));
#76746=CARTESIAN_POINT('Ctrl Pts',(7.35007323494,-39.7742356128,2.39634839519));
#76747=CARTESIAN_POINT('Ctrl Pts',(7.29780025627,-39.7742356128,2.32993852802));
#76748=CARTESIAN_POINT('Ctrl Pts',(7.25230657394,-39.7742356128,2.26107036804));
#76749=CARTESIAN_POINT('Ctrl Pts',(7.21384189758,-39.7742356128,2.18958432614));
#76750=CARTESIAN_POINT('',(9.23698117862,-39.7742356128,0.509886547137));
#76751=CARTESIAN_POINT('Ctrl Pts',(8.75956299023,-39.7742356128,2.0634404101));
#76752=CARTESIAN_POINT('Ctrl Pts',(8.92890465395,-39.7742356128,1.78598462948));
#76753=CARTESIAN_POINT('Ctrl Pts',(9.07290910839,-39.7742356128,1.49306491902));
#76754=CARTESIAN_POINT('Ctrl Pts',(9.12674985892,-39.7742356128,1.15064933619));
#76755=CARTESIAN_POINT('Ctrl Pts',(9.18664865847,-39.7742356128,0.831017278591));
#76756=CARTESIAN_POINT('Ctrl Pts',(9.23698117862,-39.7742356128,0.509886547137));
#76757=CARTESIAN_POINT('Origin',(8.43479356605655,-39.7742356128,0.840596259915162));
#76758=CARTESIAN_POINT('Origin',(-3.35265884719E-30,-39.7742356128,3.15283103411E-22));
#76759=CARTESIAN_POINT('Ctrl Pts',(4.25781969174464,-39.7742356128,-7.49892908854306));
#76760=CARTESIAN_POINT('Ctrl Pts',(4.65322788995043,-39.7742356128,-7.3163913616492));
#76761=CARTESIAN_POINT('Ctrl Pts',(5.03801677004475,-39.7742356128,-7.11164628336145));
#76762=CARTESIAN_POINT('Ctrl Pts',(5.41306173043686,-39.7742356128,-6.88530054623907));
#76763=CARTESIAN_POINT('Ctrl Pts',(6.471884508719,-39.7742356128,-6.17278862552067));
#76764=CARTESIAN_POINT('Ctrl Pts',(7.447100543,-39.7742356128,-5.31497212719));
#76765=CARTESIAN_POINT('Ctrl Pts',(8.1250786803,-39.7742356128,-4.64371494659));
#76766=CARTESIAN_POINT('Ctrl Pts',(8.99226462924,-39.7742356128,-3.46343233105));
#76767=CARTESIAN_POINT('Ctrl Pts',(9.35827765375,-39.7742356128,-2.07942227767));
#76768=CARTESIAN_POINT('Ctrl Pts',(9.40334820731,-39.7742356128,-1.48595469944));
#76769=CARTESIAN_POINT('Ctrl Pts',(9.38742862291538,-39.7742356128,-0.735709765136425));
#76770=CARTESIAN_POINT('Ctrl Pts',(9.30750311921127,-39.7742356128,0.00658879758684674));
#76771=CARTESIAN_POINT('Ctrl Pts',(9.28837293696608,-39.7742356128,0.161032819096423));
#76772=CARTESIAN_POINT('Ctrl Pts',(9.26699040489341,-39.7742356128,0.314888765115395));
#76773=CARTESIAN_POINT('Ctrl Pts',(9.24345636582343,-39.7742356128,0.468150490677146));
#76774=CARTESIAN_POINT('Origin',(-3.35265884719E-30,-39.7742356128,3.15283103411E-22));
#76775=CARTESIAN_POINT('',(1.87043161062015,-39.7742356128,-8.24476960831419));
#76776=CARTESIAN_POINT('Ctrl Pts',(1.87043161102975,-39.7742356128,-8.24476960823859));
#76777=CARTESIAN_POINT('Ctrl Pts',(2.37456097010993,-39.7742356128,-8.15400466703051));
#76778=CARTESIAN_POINT('Ctrl Pts',(2.86812085476427,-39.7742356128,-8.03407528099285));
#76779=CARTESIAN_POINT('Ctrl Pts',(3.34590835694244,-39.7742356128,-7.88493442690442));
#76780=CARTESIAN_POINT('Ctrl Pts',(3.80871374571701,-39.7742356128,-7.70625604558236));
#76781=CARTESIAN_POINT('Ctrl Pts',(4.25781969174463,-39.7742356128,-7.49892908854306));
#76782=CARTESIAN_POINT('',(1.51727342606,-39.7742356128,-7.9495168227));
#76783=CARTESIAN_POINT('Origin',(1.81727342606,-39.7742356128,-7.9495168227));
#76784=CARTESIAN_POINT('',(1.51727342606,-39.7742356128,-5.3088808072));
#76785=CARTESIAN_POINT('',(1.51727342606,-39.7742356128,-6.62919881495));
#76786=CARTESIAN_POINT('',(1.68475792039,-39.7742356128,-5.03973467448));
#76787=CARTESIAN_POINT('Origin',(1.81727342606,-39.7742356128,-5.3088808072));
#76788=CARTESIAN_POINT('Origin',(-4.74165425577699,-39.7742356127985,1.63373408714116));
#76789=CARTESIAN_POINT('Origin',(-3.35265884719E-30,-39.7742356128,3.15283103411E-22));
#76790=CARTESIAN_POINT('Ctrl Pts',(-4.25781969174463,-39.7742356128,-7.49892908854306));
#76791=CARTESIAN_POINT('Ctrl Pts',(-4.65322788995043,-39.7742356128,-7.3163913616492));
#76792=CARTESIAN_POINT('Ctrl Pts',(-5.03801677004475,-39.7742356128,-7.11164628336145));
#76793=CARTESIAN_POINT('Ctrl Pts',(-5.41306173043686,-39.7742356128,-6.88530054623907));
#76794=CARTESIAN_POINT('Ctrl Pts',(-6.471884508719,-39.7742356128,-6.17278862552066));
#76795=CARTESIAN_POINT('Ctrl Pts',(-7.447100543,-39.7742356128,-5.31497212719));
#76796=CARTESIAN_POINT('Ctrl Pts',(-8.1250786803,-39.7742356128,-4.64371494659));
#76797=CARTESIAN_POINT('Ctrl Pts',(-8.99226462924,-39.7742356128,-3.46343233105));
#76798=CARTESIAN_POINT('Ctrl Pts',(-9.35827765375,-39.7742356128,-2.07942227767));
#76799=CARTESIAN_POINT('Ctrl Pts',(-9.40334820731,-39.7742356128,-1.48595469944));
#76800=CARTESIAN_POINT('Ctrl Pts',(-9.38742862291538,-39.7742356128,-0.735709765136425));
#76801=CARTESIAN_POINT('Ctrl Pts',(-9.30750311921127,-39.7742356128,0.00658879758684674));
#76802=CARTESIAN_POINT('Ctrl Pts',(-9.28837293696608,-39.7742356128,0.161032819096423));
#76803=CARTESIAN_POINT('Ctrl Pts',(-9.26699040489341,-39.7742356128,0.314888765115395));
#76804=CARTESIAN_POINT('Ctrl Pts',(-9.24345636582343,-39.7742356128,0.468150490677146));
#76805=CARTESIAN_POINT('Origin',(-3.35265884719E-30,-39.7742356128,3.15283103411E-22));
#76806=CARTESIAN_POINT('',(-1.68475792039,-39.7742356128,-5.03973467448));
#76807=CARTESIAN_POINT('Origin',(4.74165425391462,-39.7742356127985,1.63373408533383));
#76808=CARTESIAN_POINT('',(-1.51727342606,-39.7742356128,-5.3088808072));
#76809=CARTESIAN_POINT('Origin',(-1.81727342606,-39.7742356128,-5.3088808072));
#76810=CARTESIAN_POINT('',(-1.51727342606,-39.7742356128,-7.9495168227));
#76811=CARTESIAN_POINT('',(-1.51727342606,-39.7742356128,-6.62919881495));
#76812=CARTESIAN_POINT('',(-1.87043161062015,-39.7742356128,-8.24476960831419));
#76813=CARTESIAN_POINT('Origin',(-1.81727342606,-39.7742356128,-7.9495168227));
#76814=CARTESIAN_POINT('Ctrl Pts',(-1.87043161102975,-39.7742356128,-8.24476960823859));
#76815=CARTESIAN_POINT('Ctrl Pts',(-2.37456097010993,-39.7742356128,-8.15400466703051));
#76816=CARTESIAN_POINT('Ctrl Pts',(-2.86812085476427,-39.7742356128,-8.03407528099285));
#76817=CARTESIAN_POINT('Ctrl Pts',(-3.34590835694244,-39.7742356128,-7.88493442690443));
#76818=CARTESIAN_POINT('Ctrl Pts',(-3.80871374571701,-39.7742356128,-7.70625604558236));
#76819=CARTESIAN_POINT('Ctrl Pts',(-4.25781969174463,-39.7742356128,-7.49892908854306));
#76820=CARTESIAN_POINT('Origin',(-3.35265884719E-30,-39.7742356128,3.15283103411E-22));
#76821=CARTESIAN_POINT('',(-3.67755401867,-39.7742356128,-3.05915055738));
#76822=CARTESIAN_POINT('Ctrl Pts',(-7.04639034878034,-39.7742356128,1.13407180047521));
#76823=CARTESIAN_POINT('Ctrl Pts',(-6.98577032985781,-39.7742356128,0.696425342316252));
#76824=CARTESIAN_POINT('Ctrl Pts',(-6.89012094467166,-39.7742356128,0.272653387012416));
#76825=CARTESIAN_POINT('Ctrl Pts',(-6.75651149488734,-39.7742356128,-0.133493132432014));
#76826=CARTESIAN_POINT('Ctrl Pts',(-6.39374256643522,-39.7742356128,-0.93640428199725));
#76827=CARTESIAN_POINT('Ctrl Pts',(-5.86106085412,-39.7742356128,-1.62790491519));
#76828=CARTESIAN_POINT('Ctrl Pts',(-5.53842443335,-39.7742356128,-1.95360958375));
#76829=CARTESIAN_POINT('Ctrl Pts',(-4.98933040959,-39.7742356128,-2.39194593497));
#76830=CARTESIAN_POINT('Ctrl Pts',(-4.36273333629,-39.7742356128,-2.74903878258));
#76831=CARTESIAN_POINT('Ctrl Pts',(-4.14078300625,-39.7742356128,-2.86156599489));
#76832=CARTESIAN_POINT('Ctrl Pts',(-3.91246466012,-39.7742356128,-2.96464616022));
#76833=CARTESIAN_POINT('Ctrl Pts',(-3.67755401867,-39.7742356128,-3.05915055738));
#76834=CARTESIAN_POINT('',(-3.51985615629,-39.7742356128,-3.20601908088));
#76835=CARTESIAN_POINT('Origin',(-3.78952269078,-39.7742356128,-3.33747234321));
#76836=CARTESIAN_POINT('Origin',(1143.38887689168,-39.774235612772,1093.0893729638));
#76837=CARTESIAN_POINT('',(-2.62096770799,-39.7742356128,-2.76784153979));
#76838=CARTESIAN_POINT('Ctrl Pts',(-2.62096770799,-39.7742356128,-2.76784153979));
#76839=CARTESIAN_POINT('Ctrl Pts',(-2.48674506753,-39.7742356128,-3.04318924635));
#76840=CARTESIAN_POINT('Ctrl Pts',(-2.32123277945,-39.7742356128,-3.28726285739));
#76841=CARTESIAN_POINT('Ctrl Pts',(-2.12330703536,-39.7742356128,-3.49933208248));
#76842=CARTESIAN_POINT('',(-3.30432511166,-39.7742356128,-2.13141127128));
#76843=CARTESIAN_POINT('Origin',(-3.57176864012569,-39.7742356128,-3.10366221508032));
#76844=CARTESIAN_POINT('Ctrl Pts',(-6.02437852526,-39.7742356128,1.07105719696));
#76845=CARTESIAN_POINT('Ctrl Pts',(-5.86422039559,-39.7742356128,0.163050845024));
#76846=CARTESIAN_POINT('Ctrl Pts',(-5.51798981241,-39.7742356128,-0.635658287301));
#76847=CARTESIAN_POINT('Ctrl Pts',(-4.97390737876,-39.7742356128,-1.26910580103));
#76848=CARTESIAN_POINT('Ctrl Pts',(-4.20012016579,-39.7742356128,-1.77103350786));
#76849=CARTESIAN_POINT('Ctrl Pts',(-3.30432511166,-39.7742356128,-2.13141127128));
#76850=CARTESIAN_POINT('Origin',(-3.35265884719E-30,-39.7742356128,3.15283103411E-22));
#76851=CARTESIAN_POINT('Origin',(-3.35265884719E-30,-39.7742356128,3.15283103411E-22));
#76852=CARTESIAN_POINT('',(-9.23698117862,-39.7742356128,0.509886547152));
#76853=CARTESIAN_POINT('Origin',(-8.43479129614805,-39.7742356128,0.840597206515149));
#76854=CARTESIAN_POINT('',(-8.75956299023,-39.7742356128,2.0634404101));
#76855=CARTESIAN_POINT('Ctrl Pts',(-8.75956299023,-39.7742356128,2.0634404101));
#76856=CARTESIAN_POINT('Ctrl Pts',(-8.92890465395,-39.7742356128,1.78598462948));
#76857=CARTESIAN_POINT('Ctrl Pts',(-9.07290910839,-39.7742356128,1.49306491902));
#76858=CARTESIAN_POINT('Ctrl Pts',(-9.12674985892,-39.7742356128,1.15064933619));
#76859=CARTESIAN_POINT('Ctrl Pts',(-9.18664865847,-39.7742356128,0.831017278591));
#76860=CARTESIAN_POINT('Ctrl Pts',(-9.23698117861771,-39.7742356128,0.509886547151641));
#76861=CARTESIAN_POINT('',(-7.21384189758,-39.7742356128,2.18958432614));
#76862=CARTESIAN_POINT('Ctrl Pts',(-8.75956299024,-39.7742356128,2.0634404101));
#76863=CARTESIAN_POINT('Ctrl Pts',(-8.67258032609,-39.7742356128,2.20595609378));
#76864=CARTESIAN_POINT('Ctrl Pts',(-8.57679326147,-39.7742356128,2.34786591099));
#76865=CARTESIAN_POINT('Ctrl Pts',(-8.46448329596,-39.7742356128,2.49604426586));
#76866=CARTESIAN_POINT('Ctrl Pts',(-8.27825186329,-39.7742356128,2.67220081215));
#76867=CARTESIAN_POINT('Ctrl Pts',(-8.05379939761,-39.7742356128,2.74035894609));
#76868=CARTESIAN_POINT('Ctrl Pts',(-7.9779370982,-39.7742356128,2.74765496713));
#76869=CARTESIAN_POINT('Ctrl Pts',(-7.82203636779,-39.7742356128,2.73225108729));
#76870=CARTESIAN_POINT('Ctrl Pts',(-7.67278421879,-39.7742356128,2.66639360485));
#76871=CARTESIAN_POINT('Ctrl Pts',(-7.59903734004,-39.7742356128,2.62164000818));
#76872=CARTESIAN_POINT('Ctrl Pts',(-7.46503014366,-39.7742356128,2.52047218586));
#76873=CARTESIAN_POINT('Ctrl Pts',(-7.35007323494,-39.7742356128,2.39634839519));
#76874=CARTESIAN_POINT('Ctrl Pts',(-7.29780025627,-39.7742356128,2.32993852802));
#76875=CARTESIAN_POINT('Ctrl Pts',(-7.25230657394,-39.7742356128,2.26107036804));
#76876=CARTESIAN_POINT('Ctrl Pts',(-7.21384189758,-39.7742356128,2.18958432614));
#76877=CARTESIAN_POINT('',(-7.07911993306,-39.7742356128,1.41233341424));
#76878=CARTESIAN_POINT('Ctrl Pts',(-7.21384189758,-39.7742356128,2.18958432614));
#76879=CARTESIAN_POINT('Ctrl Pts',(-7.13908599018,-39.7742356128,2.05065155888));
#76880=CARTESIAN_POINT('Ctrl Pts',(-7.08905059141,-39.7742356128,1.8984189694));
#76881=CARTESIAN_POINT('Ctrl Pts',(-7.1053290044,-39.7742356128,1.72681022597));
#76882=CARTESIAN_POINT('Ctrl Pts',(-7.09439724612,-39.7742356128,1.56936004643));
#76883=CARTESIAN_POINT('Ctrl Pts',(-7.07911993306,-39.7742356128,1.41233341424));
#76884=CARTESIAN_POINT('Ctrl Pts',(-7.07911993306,-39.7742356128,1.41233341424));
#76885=CARTESIAN_POINT('Ctrl Pts',(-7.07459783011678,-39.7742356128,1.36585334327954));
#76886=CARTESIAN_POINT('Ctrl Pts',(-7.06961906998814,-39.7742356128,1.31941671396497));
#76887=CARTESIAN_POINT('Ctrl Pts',(-7.05871909787096,-39.7742356128,1.22665564708761));
#76888=CARTESIAN_POINT('Ctrl Pts',(-7.05279772717288,-39.7742356128,1.18032989304729));
#76889=CARTESIAN_POINT('Ctrl Pts',(-7.04639034822408,-39.7742356128,1.1340717964593));
#76890=CARTESIAN_POINT('Origin',(-3.35265884719E-30,-38.2742356128,3.15283103411E-22));
#76891=CARTESIAN_POINT('',(9.47221976654,-38.2742356128,2.49225909299));
#76892=CARTESIAN_POINT('',(6.53914701908,-38.2742356128,2.5806950957));
#76893=CARTESIAN_POINT('Ctrl Pts',(9.47221976654,-38.2742356128,2.49225909299));
#76894=CARTESIAN_POINT('Ctrl Pts',(9.39947240551,-38.2742356128,2.61145111814));
#76895=CARTESIAN_POINT('Ctrl Pts',(9.32101749845,-38.2742356128,2.73104611971));
#76896=CARTESIAN_POINT('Ctrl Pts',(9.23447554945,-38.2742356128,2.85280836926));
#76897=CARTESIAN_POINT('Ctrl Pts',(9.02906684789,-38.2742356128,3.10681559939));
#76898=CARTESIAN_POINT('Ctrl Pts',(8.75253761634,-38.2742356128,3.33309151087));
#76899=CARTESIAN_POINT('Ctrl Pts',(8.5879953064,-38.2742356128,3.43383230551));
#76900=CARTESIAN_POINT('Ctrl Pts',(8.23034267354,-38.2742356128,3.56436456904));
#76901=CARTESIAN_POINT('Ctrl Pts',(7.84867458413,-38.2742356128,3.56156543232));
#76902=CARTESIAN_POINT('Ctrl Pts',(7.67119781066,-38.2742356128,3.52757441198));
#76903=CARTESIAN_POINT('Ctrl Pts',(7.27066371621,-38.2742356128,3.38466568023));
#76904=CARTESIAN_POINT('Ctrl Pts',(6.95203985001,-38.2742356128,3.13761299508));
#76905=CARTESIAN_POINT('Ctrl Pts',(6.78734156337,-38.2742356128,2.96846990237));
#76906=CARTESIAN_POINT('Ctrl Pts',(6.6484900876,-38.2742356128,2.78390759916));
#76907=CARTESIAN_POINT('Ctrl Pts',(6.53914701908,-38.2742356128,2.5806950957));
#76908=CARTESIAN_POINT('',(2.42434411094,-38.2742356128,-2.36824808793));
#76909=CARTESIAN_POINT('Ctrl Pts',(6.53914701908,-38.2742356128,2.5806950957));
#76910=CARTESIAN_POINT('Ctrl Pts',(5.92921620253,-38.2742356128,1.44714753899));
#76911=CARTESIAN_POINT('Ctrl Pts',(6.2734552887,-38.2742356128,-0.199812643821));
#76912=CARTESIAN_POINT('Ctrl Pts',(4.66846608736,-38.2742356128,-1.09094389297));
#76913=CARTESIAN_POINT('Ctrl Pts',(3.58890539941,-38.2742356128,-1.81984798791));
#76914=CARTESIAN_POINT('Ctrl Pts',(2.42434411094,-38.2742356128,-2.36824808793));
#76915=CARTESIAN_POINT('',(1.11895565834,-38.2742356128,-2.79941259037));
#76916=CARTESIAN_POINT('Origin',(5.88418203051333E-14,-38.2742356128,2.77999550540993));
#76917=CARTESIAN_POINT('',(0.717273426056,-38.2742356128,-3.28965091665));
#76918=CARTESIAN_POINT('Origin',(1.21727342606,-38.2742356128,-3.28965091665));
#76919=CARTESIAN_POINT('',(0.717273426056,-38.2742356128,-7.9495168227));
#76920=CARTESIAN_POINT('',(0.717273426056,-38.2742356128,0.717427860236));
#76921=CARTESIAN_POINT('',(2.02820898725,-38.2742356128,-9.02284995699));
#76922=CARTESIAN_POINT('Origin',(1.81725567298,-38.2742356128,-7.94326730652));
#76923=CARTESIAN_POINT('',(2.06575948168,-38.2742356128,-9.01576047707));
#76924=CARTESIAN_POINT('Origin',(2.60353656354866,-38.2742356128,-11.9671681877212));
#76925=CARTESIAN_POINT('',(10.0571285787,-38.2742356128,0.645805825719));
#76926=CARTESIAN_POINT('Ctrl Pts',(2.06575948168004,-38.2742356128,-9.0157604770702));
#76927=CARTESIAN_POINT('Ctrl Pts',(2.96721946584242,-38.2742356128,-8.8515051248253));
#76928=CARTESIAN_POINT('Ctrl Pts',(3.84599035268564,-38.2742356128,-8.59864711375854));
#76929=CARTESIAN_POINT('Ctrl Pts',(4.67357601907077,-38.2742356128,-8.25401330976187));
#76930=CARTESIAN_POINT('Ctrl Pts',(6.17345275440962,-38.2742356128,-7.42645694768941));
#76931=CARTESIAN_POINT('Ctrl Pts',(7.5161640814,-38.2742356128,-6.34532321195));
#76932=CARTESIAN_POINT('Ctrl Pts',(8.15806093588,-38.2742356128,-5.76170299258));
#76933=CARTESIAN_POINT('Ctrl Pts',(9.14108523272,-38.2742356128,-4.69984607968));
#76934=CARTESIAN_POINT('Ctrl Pts',(9.81302959348,-38.2742356128,-3.42961050122));
#76935=CARTESIAN_POINT('Ctrl Pts',(10.0098671635,-38.2742356128,-2.88411398337));
#76936=CARTESIAN_POINT('Ctrl Pts',(10.222733632,-38.2742356128,-1.82926592992));
#76937=CARTESIAN_POINT('Ctrl Pts',(10.2199521215,-38.2742356128,-0.771812654558));
#76938=CARTESIAN_POINT('Ctrl Pts',(10.184046519,-38.2742356128,-0.287190507733));
#76939=CARTESIAN_POINT('Ctrl Pts',(10.1298079404,-38.2742356128,0.182098137249));
#76940=CARTESIAN_POINT('Ctrl Pts',(10.0571285787022,-38.2742356128,0.645805825719337));
#76941=CARTESIAN_POINT('Ctrl Pts',(9.47221976654,-38.2742356128,2.49225909299));
#76942=CARTESIAN_POINT('Ctrl Pts',(9.54575444005,-38.2742356128,2.3717771053));
#76943=CARTESIAN_POINT('Ctrl Pts',(9.61961951766,-38.2742356128,2.24151541202));
#76944=CARTESIAN_POINT('Ctrl Pts',(9.68609489427,-38.2742356128,2.10542437124));
#76945=CARTESIAN_POINT('Ctrl Pts',(9.84457330898,-38.2742356128,1.72211870919));
#76946=CARTESIAN_POINT('Ctrl Pts',(9.94207621049,-38.2742356128,1.33157301839));
#76947=CARTESIAN_POINT('Ctrl Pts',(9.98299011243,-38.2742356128,1.0898271634));
#76948=CARTESIAN_POINT('Ctrl Pts',(10.0216701384,-38.2742356128,0.872037193625));
#76949=CARTESIAN_POINT('Ctrl Pts',(10.0571285787,-38.2742356128,0.645805825719));
#76950=CARTESIAN_POINT('',(-5.2400559546,-38.2742356128,5.59690998219));
#76951=CARTESIAN_POINT('',(-4.39152711004478,-38.2742356128,1.85538989759538));
#76952=CARTESIAN_POINT('Ctrl Pts',(-5.2400559546,-38.2742356128,5.59690998219));
#76953=CARTESIAN_POINT('Ctrl Pts',(-5.25990082634,-38.2742356128,5.0059883748));
#76954=CARTESIAN_POINT('Ctrl Pts',(-5.23061607717,-38.2742356128,4.36229648927));
#76955=CARTESIAN_POINT('Ctrl Pts',(-5.00490058958,-38.2742356128,3.77298874453));
#76956=CARTESIAN_POINT('Ctrl Pts',(-4.75506448705,-38.2742356128,3.08655684628));
#76957=CARTESIAN_POINT('Ctrl Pts',(-4.54755634075,-38.2742356128,2.39287258614));
#76958=CARTESIAN_POINT('Ctrl Pts',(-4.4987250478,-38.2742356128,2.21955031284));
#76959=CARTESIAN_POINT('Ctrl Pts',(-4.44893332626,-38.2742356128,2.04003858973));
#76960=CARTESIAN_POINT('Ctrl Pts',(-4.39152710765,-38.2742356128,1.85538989834));
#76961=CARTESIAN_POINT('',(-0.605290084208,-38.2742356128,-1.95105924441));
#76962=CARTESIAN_POINT('Ctrl Pts',(-0.605290084206,-38.2742356128,-1.95105924441));
#76963=CARTESIAN_POINT('Ctrl Pts',(-0.774096521679,-38.2742356128,-1.91628513625));
#76964=CARTESIAN_POINT('Ctrl Pts',(-0.942624183674,-38.2742356128,-1.87619510128));
#76965=CARTESIAN_POINT('Ctrl Pts',(-1.11061388614,-38.2742356128,-1.83037525603));
#76966=CARTESIAN_POINT('Ctrl Pts',(-1.74274860628,-38.2742356128,-1.63293852912));
#76967=CARTESIAN_POINT('Ctrl Pts',(-2.34679547467,-38.2742356128,-1.33257881069));
#76968=CARTESIAN_POINT('Ctrl Pts',(-2.73083933763,-38.2742356128,-1.04090474176));
#76969=CARTESIAN_POINT('Ctrl Pts',(-3.39638296129,-38.2742356128,-0.293897533174));
#76970=CARTESIAN_POINT('Ctrl Pts',(-3.86916001537,-38.2742356128,0.542814468562));
#76971=CARTESIAN_POINT('Ctrl Pts',(-4.06911877342,-38.2742356128,0.942104314053));
#76972=CARTESIAN_POINT('Ctrl Pts',(-4.24744781279,-38.2742356128,1.39201586348));
#76973=CARTESIAN_POINT('Ctrl Pts',(-4.39143626207,-38.2742356128,1.85509771049));
#76974=CARTESIAN_POINT('Ctrl Pts',(-4.39145443226365,-38.2742356128,1.85515614772492));
#76975=CARTESIAN_POINT('Ctrl Pts',(-4.3914726024573,-38.2742356128,1.85521458495984));
#76976=CARTESIAN_POINT('Ctrl Pts',(-4.39149077265095,-38.2742356128,1.85527302219476));
#76977=CARTESIAN_POINT('Ctrl Pts',(-4.3915089428446,-38.2742356128,1.85533145942968));
#76978=CARTESIAN_POINT('Ctrl Pts',(-4.39152711303826,-38.2742356128,1.8553898966646));
#76979=CARTESIAN_POINT('',(0.605290084208,-38.2742356128,-1.95105924441));
#76980=CARTESIAN_POINT('Origin',(1.39679934285653E-13,-38.2742356128,0.987243652491003));
#76981=CARTESIAN_POINT('',(4.39138551652333,-38.2742356128,1.85493449099992));
#76982=CARTESIAN_POINT('Ctrl Pts',(0.605290084206,-38.2742356128,-1.95105924441));
#76983=CARTESIAN_POINT('Ctrl Pts',(0.774096521679,-38.2742356128,-1.91628513625));
#76984=CARTESIAN_POINT('Ctrl Pts',(0.942624183674,-38.2742356128,-1.87619510128));
#76985=CARTESIAN_POINT('Ctrl Pts',(1.11061388614,-38.2742356128,-1.83037525603));
#76986=CARTESIAN_POINT('Ctrl Pts',(1.74274860628,-38.2742356128,-1.63293852912));
#76987=CARTESIAN_POINT('Ctrl Pts',(2.34679547467,-38.2742356128,-1.33257881069));
#76988=CARTESIAN_POINT('Ctrl Pts',(2.73083933763,-38.2742356128,-1.04090474176));
#76989=CARTESIAN_POINT('Ctrl Pts',(3.39635927668,-38.2742356128,-0.29392411682));
#76990=CARTESIAN_POINT('Ctrl Pts',(3.86912636582,-38.2742356128,0.542754916759));
#76991=CARTESIAN_POINT('Ctrl Pts',(4.06899942193,-38.2742356128,0.941795900815));
#76992=CARTESIAN_POINT('Ctrl Pts',(4.2473975181,-38.2742356128,1.39188897252));
#76993=CARTESIAN_POINT('Ctrl Pts',(4.39138551009,-38.2742356128,1.854934493));
#76994=CARTESIAN_POINT('',(5.2400559546,-38.2742356128,5.59690998219));
#76995=CARTESIAN_POINT('Ctrl Pts',(5.2400559546,-38.2742356128,5.59690998219));
#76996=CARTESIAN_POINT('Ctrl Pts',(5.25990082634,-38.2742356128,5.0059883748));
#76997=CARTESIAN_POINT('Ctrl Pts',(5.23061607717,-38.2742356128,4.36229648927));
#76998=CARTESIAN_POINT('Ctrl Pts',(5.00490058958,-38.2742356128,3.77298874453));
#76999=CARTESIAN_POINT('Ctrl Pts',(4.75506448705,-38.2742356128,3.08655684628));
#77000=CARTESIAN_POINT('Ctrl Pts',(4.54755634075,-38.2742356128,2.39287258614));
#77001=CARTESIAN_POINT('Ctrl Pts',(4.4987250478,-38.2742356128,2.21955031284));
#77002=CARTESIAN_POINT('Ctrl Pts',(4.44893332626,-38.2742356128,2.04003858973));
#77003=CARTESIAN_POINT('Ctrl Pts',(4.39152710765,-38.2742356128,1.85538989834));
#77004=CARTESIAN_POINT('Ctrl Pts',(4.3914987908103,-38.2742356128,1.8552988164412));
#77005=CARTESIAN_POINT('Ctrl Pts',(4.39147047397061,-38.2742356128001,1.85520773454239));
#77006=CARTESIAN_POINT('Ctrl Pts',(4.39144215713091,-38.2742356128001,1.85511665264359));
#77007=CARTESIAN_POINT('Ctrl Pts',(4.39141384029122,-38.2742356128001,1.85502557074478));
#77008=CARTESIAN_POINT('Ctrl Pts',(4.39138552345152,-38.2742356128001,1.85493448884598));
#77009=CARTESIAN_POINT('',(-7.34769233304E-15,-38.2742356128,10.664345987));
#77010=CARTESIAN_POINT('Origin',(-0.000416107150120478,-38.2742356128,5.42091963994));
#77011=CARTESIAN_POINT('Origin',(0.00041610715012382,-38.2742356128,5.42091963994));
#77012=CARTESIAN_POINT('',(-2.06575948168,-38.2742356128,-9.01576047707));
#77013=CARTESIAN_POINT('',(-2.02820898725,-38.2742356128,-9.02284995699));
#77014=CARTESIAN_POINT('Origin',(-2.60353654477611,-38.2742356128,-11.967168053913));
#77015=CARTESIAN_POINT('',(-0.717273426055,-38.2742356128,-7.9495168227));
#77016=CARTESIAN_POINT('Origin',(-1.81725567298,-38.2742356128,-7.94326730652));
#77017=CARTESIAN_POINT('',(-0.717273426056,-38.2742356128,-3.28965091665));
#77018=CARTESIAN_POINT('',(-0.717273426056,-38.2742356128,0.717427860236));
#77019=CARTESIAN_POINT('',(-1.11895565834,-38.2742356128,-2.79941259037));
#77020=CARTESIAN_POINT('Origin',(-1.21727342606,-38.2742356128,-3.28965091665));
#77021=CARTESIAN_POINT('',(-2.42434411094,-38.2742356128,-2.36824808793));
#77022=CARTESIAN_POINT('Origin',(-5.88418203051333E-14,-38.2742356128,2.77999550540993));
#77023=CARTESIAN_POINT('',(-6.53914701908,-38.2742356128,2.5806950957));
#77024=CARTESIAN_POINT('Ctrl Pts',(-6.53914701908,-38.2742356128,2.5806950957));
#77025=CARTESIAN_POINT('Ctrl Pts',(-5.92921620253,-38.2742356128,1.44714753899));
#77026=CARTESIAN_POINT('Ctrl Pts',(-6.2734552887,-38.2742356128,-0.199812643821));
#77027=CARTESIAN_POINT('Ctrl Pts',(-4.66846608736,-38.2742356128,-1.09094389297));
#77028=CARTESIAN_POINT('Ctrl Pts',(-3.58890539941,-38.2742356128,-1.81984798791));
#77029=CARTESIAN_POINT('Ctrl Pts',(-2.42434411094,-38.2742356128,-2.36824808793));
#77030=CARTESIAN_POINT('',(-9.47221976654,-38.2742356128,2.49225909299));
#77031=CARTESIAN_POINT('Ctrl Pts',(-9.47221976654,-38.2742356128,2.49225909299));
#77032=CARTESIAN_POINT('Ctrl Pts',(-9.39947240551,-38.2742356128,2.61145111814));
#77033=CARTESIAN_POINT('Ctrl Pts',(-9.32101749845,-38.2742356128,2.73104611971));
#77034=CARTESIAN_POINT('Ctrl Pts',(-9.23447554945,-38.2742356128,2.85280836926));
#77035=CARTESIAN_POINT('Ctrl Pts',(-9.02906684789,-38.2742356128,3.10681559939));
#77036=CARTESIAN_POINT('Ctrl Pts',(-8.75253761634,-38.2742356128,3.33309151087));
#77037=CARTESIAN_POINT('Ctrl Pts',(-8.5879953064,-38.2742356128,3.43383230551));
#77038=CARTESIAN_POINT('Ctrl Pts',(-8.23034267354,-38.2742356128,3.56436456904));
#77039=CARTESIAN_POINT('Ctrl Pts',(-7.84867458413,-38.2742356128,3.56156543232));
#77040=CARTESIAN_POINT('Ctrl Pts',(-7.67119781066,-38.2742356128,3.52757441198));
#77041=CARTESIAN_POINT('Ctrl Pts',(-7.27066371621,-38.2742356128,3.38466568023));
#77042=CARTESIAN_POINT('Ctrl Pts',(-6.95203985001,-38.2742356128,3.13761299508));
#77043=CARTESIAN_POINT('Ctrl Pts',(-6.78734156337,-38.2742356128,2.96846990237));
#77044=CARTESIAN_POINT('Ctrl Pts',(-6.6484900876,-38.2742356128,2.78390759916));
#77045=CARTESIAN_POINT('Ctrl Pts',(-6.53914701908,-38.2742356128,2.5806950957));
#77046=CARTESIAN_POINT('',(-10.0571285787,-38.2742356128,0.645805825719));
#77047=CARTESIAN_POINT('Ctrl Pts',(-9.47221976654,-38.2742356128,2.49225909299));
#77048=CARTESIAN_POINT('Ctrl Pts',(-9.54575444005,-38.2742356128,2.3717771053));
#77049=CARTESIAN_POINT('Ctrl Pts',(-9.61961951766,-38.2742356128,2.24151541202));
#77050=CARTESIAN_POINT('Ctrl Pts',(-9.68609489427,-38.2742356128,2.10542437124));
#77051=CARTESIAN_POINT('Ctrl Pts',(-9.84457330898,-38.2742356128,1.72211870919));
#77052=CARTESIAN_POINT('Ctrl Pts',(-9.94207621049,-38.2742356128,1.33157301839));
#77053=CARTESIAN_POINT('Ctrl Pts',(-9.98299011243,-38.2742356128,1.0898271634));
#77054=CARTESIAN_POINT('Ctrl Pts',(-10.0216701384,-38.2742356128,0.872037193625));
#77055=CARTESIAN_POINT('Ctrl Pts',(-10.0571285787,-38.2742356128,0.645805825719));
#77056=CARTESIAN_POINT('Ctrl Pts',(-2.06575948168004,-38.2742356128,-9.0157604770702));
#77057=CARTESIAN_POINT('Ctrl Pts',(-2.96721946584242,-38.2742356128,-8.8515051248253));
#77058=CARTESIAN_POINT('Ctrl Pts',(-3.84599035268564,-38.2742356128,-8.59864711375854));
#77059=CARTESIAN_POINT('Ctrl Pts',(-4.67357601907077,-38.2742356128,-8.25401330976187));
#77060=CARTESIAN_POINT('Ctrl Pts',(-6.17345275440962,-38.2742356128,-7.42645694768941));
#77061=CARTESIAN_POINT('Ctrl Pts',(-7.5161640814,-38.2742356128,-6.34532321195));
#77062=CARTESIAN_POINT('Ctrl Pts',(-8.15806093588,-38.2742356128,-5.76170299258));
#77063=CARTESIAN_POINT('Ctrl Pts',(-9.14108523272,-38.2742356128,-4.69984607968));
#77064=CARTESIAN_POINT('Ctrl Pts',(-9.81302959348,-38.2742356128,-3.42961050122));
#77065=CARTESIAN_POINT('Ctrl Pts',(-10.0098671635,-38.2742356128,-2.88411398337));
#77066=CARTESIAN_POINT('Ctrl Pts',(-10.222733632,-38.2742356128,-1.82926592992));
#77067=CARTESIAN_POINT('Ctrl Pts',(-10.2199521215,-38.2742356128,-0.771812654558));
#77068=CARTESIAN_POINT('Ctrl Pts',(-10.184046519,-38.2742356128,-0.287190507733));
#77069=CARTESIAN_POINT('Ctrl Pts',(-10.1298079404,-38.2742356128,0.182098137249));
#77070=CARTESIAN_POINT('Ctrl Pts',(-10.0571285787022,-38.2742356128,0.645805825719337));
#77071=CARTESIAN_POINT('Origin',(-0.000416107150126,-37.6642356128,5.42091963994));
#77072=CARTESIAN_POINT('',(3.98812927127E-15,-37.2742356128,9.86434598407));
#77073=CARTESIAN_POINT('Origin',(-0.000416107150126,-37.2742356128,5.42091963994));
#77074=CARTESIAN_POINT('',(-1.02820313028E-15,-39.6642356128,9.86434598407));
#77075=CARTESIAN_POINT('Origin',(0.000416107150126,-37.6642356128,5.42091963994));
#77076=CARTESIAN_POINT('Origin',(0.000416107150126,-37.2742356128,5.42091963994));
#77077=CARTESIAN_POINT('Ctrl Pts',(0.772076508424,-39.7742356128,-1.09035382089));
#77078=CARTESIAN_POINT('Ctrl Pts',(0.772076508424,-36.7742356128,-1.09035382089));
#77079=CARTESIAN_POINT('Ctrl Pts',(0.886178610516,-39.7742356128,-1.05996501737));
#77080=CARTESIAN_POINT('Ctrl Pts',(0.886178610516,-36.7742356128,-1.05996501737));
#77081=CARTESIAN_POINT('Ctrl Pts',(0.999471783383,-39.7742356128,-1.02648938573));
#77082=CARTESIAN_POINT('Ctrl Pts',(0.999471783383,-36.7742356128,-1.02648938573));
#77083=CARTESIAN_POINT('Ctrl Pts',(1.11165616418,-39.7742356128,-0.989701314619));
#77084=CARTESIAN_POINT('Ctrl Pts',(1.11165616418,-36.7742356128,-0.989701314619));
#77085=CARTESIAN_POINT('Ctrl Pts',(1.3921632233,-39.7742356128,-0.887346335547));
#77086=CARTESIAN_POINT('Ctrl Pts',(1.3921632233,-36.7742356128,-0.887346335547));
#77087=CARTESIAN_POINT('Ctrl Pts',(1.65990259641,-39.7742356128,-0.759470300753));
#77088=CARTESIAN_POINT('Ctrl Pts',(1.65990259641,-36.7742356128,-0.759470300753));
#77089=CARTESIAN_POINT('Ctrl Pts',(1.81552533939,-39.7742356128,-0.67135889116));
#77090=CARTESIAN_POINT('Ctrl Pts',(1.81552533939,-36.7742356128,-0.67135889116));
#77091=CARTESIAN_POINT('Ctrl Pts',(2.13001246648,-39.7742356128,-0.455784308931));
#77092=CARTESIAN_POINT('Ctrl Pts',(2.13001246648,-36.7742356128,-0.455784308931));
#77093=CARTESIAN_POINT('Ctrl Pts',(2.40225756964,-39.7742356128,-0.187376365848));
#77094=CARTESIAN_POINT('Ctrl Pts',(2.40225756964,-36.7742356128,-0.187376365848));
#77095=CARTESIAN_POINT('Ctrl Pts',(2.53491876149,-39.7742356128,-0.0306790811922));
#77096=CARTESIAN_POINT('Ctrl Pts',(2.53491876149,-36.7742356128,-0.0306790811922));
#77097=CARTESIAN_POINT('Ctrl Pts',(2.74588721076,-39.7742356128,0.250416153254));
#77098=CARTESIAN_POINT('Ctrl Pts',(2.74588721076,-36.7742356128,0.250416153254));
#77099=CARTESIAN_POINT('Ctrl Pts',(2.93290680803,-39.7742356128,0.545770364295));
#77100=CARTESIAN_POINT('Ctrl Pts',(2.93290680803,-36.7742356128,0.545770364295));
#77101=CARTESIAN_POINT('Ctrl Pts',(3.00715366555,-39.7742356128,0.670355528577));
#77102=CARTESIAN_POINT('Ctrl Pts',(3.00715366555,-36.7742356128,0.670355528577));
#77103=CARTESIAN_POINT('Ctrl Pts',(3.20108514097,-39.7742356128,1.0165930916));
#77104=CARTESIAN_POINT('Ctrl Pts',(3.20108514097,-36.7742356128,1.0165930916));
#77105=CARTESIAN_POINT('Ctrl Pts',(3.36887363395,-39.7742356128,1.37561285195));
#77106=CARTESIAN_POINT('Ctrl Pts',(3.36887363395,-36.7742356128,1.37561285195));
#77107=CARTESIAN_POINT('Ctrl Pts',(3.46527948246,-39.7742356128,1.60915269898));
#77108=CARTESIAN_POINT('Ctrl Pts',(3.46527948246,-36.7742356128,1.60915269898));
#77109=CARTESIAN_POINT('Ctrl Pts',(3.55147728822,-39.7742356128,1.84810892036));
#77110=CARTESIAN_POINT('Ctrl Pts',(3.55147728822,-36.7742356128,1.84810892036));
#77111=CARTESIAN_POINT('Ctrl Pts',(3.62746705121,-39.7742356128,2.09248151608));
#77112=CARTESIAN_POINT('Ctrl Pts',(3.62746705121,-36.7742356128,2.09248151608));
#77113=CARTESIAN_POINT('',(0.772076508359764,-37.2742356128,-1.09035382049956));
#77114=CARTESIAN_POINT('Ctrl Pts',(0.772076508424,-37.2742356128,-1.09035382089));
#77115=CARTESIAN_POINT('Ctrl Pts',(0.886178610516,-37.2742356128,-1.05996501737));
#77116=CARTESIAN_POINT('Ctrl Pts',(0.999471783383,-37.2742356128,-1.02648938573));
#77117=CARTESIAN_POINT('Ctrl Pts',(1.11165616418,-37.2742356128,-0.989701314619));
#77118=CARTESIAN_POINT('Ctrl Pts',(1.3921632233,-37.2742356128,-0.887346335547));
#77119=CARTESIAN_POINT('Ctrl Pts',(1.65990259641,-37.2742356128,-0.759470300753));
#77120=CARTESIAN_POINT('Ctrl Pts',(1.81552533939,-37.2742356128,-0.67135889116));
#77121=CARTESIAN_POINT('Ctrl Pts',(2.13001246648,-37.2742356128,-0.455784308931));
#77122=CARTESIAN_POINT('Ctrl Pts',(2.40225756964,-37.2742356128,-0.187376365848));
#77123=CARTESIAN_POINT('Ctrl Pts',(2.53491876149,-37.2742356128,-0.0306790811922));
#77124=CARTESIAN_POINT('Ctrl Pts',(2.74588721076,-37.2742356128,0.250416153254));
#77125=CARTESIAN_POINT('Ctrl Pts',(2.93290680803,-37.2742356128,0.545770364295));
#77126=CARTESIAN_POINT('Ctrl Pts',(3.00715366555,-37.2742356128,0.670355528577));
#77127=CARTESIAN_POINT('Ctrl Pts',(3.20108514097,-37.2742356128,1.0165930916));
#77128=CARTESIAN_POINT('Ctrl Pts',(3.36887363395,-37.2742356128,1.37561285195));
#77129=CARTESIAN_POINT('Ctrl Pts',(3.46527948246,-37.2742356128,1.60915269898));
#77130=CARTESIAN_POINT('Ctrl Pts',(3.55147728822,-37.2742356128,1.84810892036));
#77131=CARTESIAN_POINT('Ctrl Pts',(3.62746705121,-37.2742356128,2.09248151608));
#77132=CARTESIAN_POINT('',(0.772076508426,-39.6642356128,-1.09035382089));
#77133=CARTESIAN_POINT('Origin',(-3.35265884719E-30,-37.2742356128,3.15283103411E-22));
#77134=CARTESIAN_POINT('',(-0.605290084059043,-37.2742356128,-1.95105924377086));
#77135=CARTESIAN_POINT('',(-4.39152711004478,-37.2742356128,1.85538989759537));
#77136=CARTESIAN_POINT('Ctrl Pts',(-0.605290084206,-37.2742356128,-1.95105924441));
#77137=CARTESIAN_POINT('Ctrl Pts',(-0.774096521679,-37.2742356128,-1.91628513625));
#77138=CARTESIAN_POINT('Ctrl Pts',(-0.942624183674,-37.2742356128,-1.87619510128));
#77139=CARTESIAN_POINT('Ctrl Pts',(-1.11061388614,-37.2742356128,-1.83037525603));
#77140=CARTESIAN_POINT('Ctrl Pts',(-1.74274860628,-37.2742356128,-1.63293852912));
#77141=CARTESIAN_POINT('Ctrl Pts',(-2.34679547467,-37.2742356128,-1.33257881069));
#77142=CARTESIAN_POINT('Ctrl Pts',(-2.73083933763,-37.2742356128,-1.04090474176));
#77143=CARTESIAN_POINT('Ctrl Pts',(-3.39638296129,-37.2742356128,-0.293897533174));
#77144=CARTESIAN_POINT('Ctrl Pts',(-3.86916001537,-37.2742356128,0.542814468562));
#77145=CARTESIAN_POINT('Ctrl Pts',(-4.06911877342,-37.2742356128,0.942104314053));
#77146=CARTESIAN_POINT('Ctrl Pts',(-4.24744781279,-37.2742356128,1.39201586348));
#77147=CARTESIAN_POINT('Ctrl Pts',(-4.39143626207,-37.2742356128,1.85509771049));
#77148=CARTESIAN_POINT('Ctrl Pts',(-4.39145443226365,-37.2742356128,1.85515614772492));
#77149=CARTESIAN_POINT('Ctrl Pts',(-4.3914726024573,-37.2742356128,1.85521458495984));
#77150=CARTESIAN_POINT('Ctrl Pts',(-4.39149077265095,-37.2742356128,1.85527302219476));
#77151=CARTESIAN_POINT('Ctrl Pts',(-4.3915089428446,-37.2742356128,1.85533145942968));
#77152=CARTESIAN_POINT('Ctrl Pts',(-4.39152711303826,-37.2742356128,1.8553898966646));
#77153=CARTESIAN_POINT('',(-5.2400559546,-37.2742356128,5.59690998219));
#77154=CARTESIAN_POINT('Ctrl Pts',(-5.2400559546,-37.2742356128,5.59690998219));
#77155=CARTESIAN_POINT('Ctrl Pts',(-5.25990082634,-37.2742356128,5.0059883748));
#77156=CARTESIAN_POINT('Ctrl Pts',(-5.23061607717,-37.2742356128,4.36229648927));
#77157=CARTESIAN_POINT('Ctrl Pts',(-5.00490058958,-37.2742356128,3.77298874453));
#77158=CARTESIAN_POINT('Ctrl Pts',(-4.75506448705,-37.2742356128,3.08655684628));
#77159=CARTESIAN_POINT('Ctrl Pts',(-4.54755634075,-37.2742356128,2.39287258614));
#77160=CARTESIAN_POINT('Ctrl Pts',(-4.4987250478,-37.2742356128,2.21955031284));
#77161=CARTESIAN_POINT('Ctrl Pts',(-4.44893332626,-37.2742356128,2.04003858973));
#77162=CARTESIAN_POINT('Ctrl Pts',(-4.39152710765,-37.2742356128,1.85538989834));
#77163=CARTESIAN_POINT('',(4.37703259054E-15,-37.2742356128,10.664345987));
#77164=CARTESIAN_POINT('Origin',(0.000416107150126,-37.2742356128,5.42091963994));
#77165=CARTESIAN_POINT('',(5.2400559546,-37.2742356128,5.59690998219));
#77166=CARTESIAN_POINT('Origin',(-0.000416107150126,-37.2742356128,5.42091963994));
#77167=CARTESIAN_POINT('',(4.39138551612134,-37.2742356128,1.85493449668939));
#77168=CARTESIAN_POINT('Ctrl Pts',(5.2400559546,-37.2742356128,5.59690998219));
#77169=CARTESIAN_POINT('Ctrl Pts',(5.25990082634,-37.2742356128,5.0059883748));
#77170=CARTESIAN_POINT('Ctrl Pts',(5.23061607717,-37.2742356128,4.36229648927));
#77171=CARTESIAN_POINT('Ctrl Pts',(5.00490058958,-37.2742356128,3.77298874453));
#77172=CARTESIAN_POINT('Ctrl Pts',(4.75506448705,-37.2742356128,3.08655684628));
#77173=CARTESIAN_POINT('Ctrl Pts',(4.54755634075,-37.2742356128,2.39287258614));
#77174=CARTESIAN_POINT('Ctrl Pts',(4.4987250478,-37.2742356128,2.21955031284));
#77175=CARTESIAN_POINT('Ctrl Pts',(4.44893332626,-37.2742356128,2.04003858973));
#77176=CARTESIAN_POINT('Ctrl Pts',(4.39152710765,-37.2742356128,1.85538989834));
#77177=CARTESIAN_POINT('Ctrl Pts',(4.39149879112577,-37.2742356128,1.8552988174559));
#77178=CARTESIAN_POINT('Ctrl Pts',(4.39147047460154,-37.2742356128,1.85520773657181));
#77179=CARTESIAN_POINT('Ctrl Pts',(4.39144215807731,-37.2742356128,1.85511665568771));
#77180=CARTESIAN_POINT('Ctrl Pts',(4.39141384155308,-37.2742356128,1.85502557480361));
#77181=CARTESIAN_POINT('Ctrl Pts',(4.39138552502885,-37.2742356128,1.85493449391952));
#77182=CARTESIAN_POINT('',(0.605290084059048,-37.2742356128,-1.95105924377088));
#77183=CARTESIAN_POINT('Ctrl Pts',(0.605290084206,-37.2742356128,-1.95105924441));
#77184=CARTESIAN_POINT('Ctrl Pts',(0.774096521679,-37.2742356128,-1.91628513625));
#77185=CARTESIAN_POINT('Ctrl Pts',(0.942624183674,-37.2742356128,-1.87619510128));
#77186=CARTESIAN_POINT('Ctrl Pts',(1.11061388614,-37.2742356128,-1.83037525603));
#77187=CARTESIAN_POINT('Ctrl Pts',(1.74274860628,-37.2742356128,-1.63293852912));
#77188=CARTESIAN_POINT('Ctrl Pts',(2.34679547467,-37.2742356128,-1.33257881069));
#77189=CARTESIAN_POINT('Ctrl Pts',(2.73083933763,-37.2742356128,-1.04090474176));
#77190=CARTESIAN_POINT('Ctrl Pts',(3.39635927668,-37.2742356128,-0.29392411682));
#77191=CARTESIAN_POINT('Ctrl Pts',(3.86912636582,-37.2742356128,0.542754916759));
#77192=CARTESIAN_POINT('Ctrl Pts',(4.06899942193,-37.2742356128,0.941795900815));
#77193=CARTESIAN_POINT('Ctrl Pts',(4.2473975181,-37.2742356128,1.39188897252));
#77194=CARTESIAN_POINT('Ctrl Pts',(4.39138551009,-37.2742356128,1.854934493));
#77195=CARTESIAN_POINT('Origin',(1.44440015504E-13,-37.2742356128,0.987243652491));
#77196=CARTESIAN_POINT('',(-0.772076508359766,-37.2742356128,-1.09035382049957));
#77197=CARTESIAN_POINT('Origin',(-3.57491813929E-14,-37.2742356128,1.80859389597));
#77198=CARTESIAN_POINT('Ctrl Pts',(-0.772076508424,-37.2742356128,-1.09035382089));
#77199=CARTESIAN_POINT('Ctrl Pts',(-0.886178610516,-37.2742356128,-1.05996501737));
#77200=CARTESIAN_POINT('Ctrl Pts',(-0.999471783383,-37.2742356128,-1.02648938573));
#77201=CARTESIAN_POINT('Ctrl Pts',(-1.11165616418,-37.2742356128,-0.989701314619));
#77202=CARTESIAN_POINT('Ctrl Pts',(-1.3921632233,-37.2742356128,-0.887346335547));
#77203=CARTESIAN_POINT('Ctrl Pts',(-1.65990259641,-37.2742356128,-0.759470300753));
#77204=CARTESIAN_POINT('Ctrl Pts',(-1.81552533939,-37.2742356128,-0.67135889116));
#77205=CARTESIAN_POINT('Ctrl Pts',(-2.13001246648,-37.2742356128,-0.455784308931));
#77206=CARTESIAN_POINT('Ctrl Pts',(-2.40225756964,-37.2742356128,-0.187376365848));
#77207=CARTESIAN_POINT('Ctrl Pts',(-2.53491876149,-37.2742356128,-0.0306790811922));
#77208=CARTESIAN_POINT('Ctrl Pts',(-2.74588721076,-37.2742356128,0.250416153254));
#77209=CARTESIAN_POINT('Ctrl Pts',(-2.93290680803,-37.2742356128,0.545770364295));
#77210=CARTESIAN_POINT('Ctrl Pts',(-3.00715366555,-37.2742356128,0.670355528577));
#77211=CARTESIAN_POINT('Ctrl Pts',(-3.20108514097,-37.2742356128,1.0165930916));
#77212=CARTESIAN_POINT('Ctrl Pts',(-3.36887363395,-37.2742356128,1.37561285195));
#77213=CARTESIAN_POINT('Ctrl Pts',(-3.46527948246,-37.2742356128,1.60915269898));
#77214=CARTESIAN_POINT('Ctrl Pts',(-3.55147728822,-37.2742356128,1.84810892036));
#77215=CARTESIAN_POINT('Ctrl Pts',(-3.62746705121,-37.2742356128,2.09248151608));
#77216=CARTESIAN_POINT('Origin',(-3.57491813929E-14,-38.2742356128,1.80859389597));
#77217=CARTESIAN_POINT('',(-0.772076508426,-38.2742356128,-1.09035382089));
#77218=CARTESIAN_POINT('Ctrl Pts',(-0.772076508424,-39.7742356128,-1.09035382089));
#77219=CARTESIAN_POINT('Ctrl Pts',(-0.772076508424,-36.7742356128,-1.09035382089));
#77220=CARTESIAN_POINT('Ctrl Pts',(-0.886178610516,-39.7742356128,-1.05996501737));
#77221=CARTESIAN_POINT('Ctrl Pts',(-0.886178610516,-36.7742356128,-1.05996501737));
#77222=CARTESIAN_POINT('Ctrl Pts',(-0.999471783383,-39.7742356128,-1.02648938573));
#77223=CARTESIAN_POINT('Ctrl Pts',(-0.999471783383,-36.7742356128,-1.02648938573));
#77224=CARTESIAN_POINT('Ctrl Pts',(-1.11165616418,-39.7742356128,-0.989701314619));
#77225=CARTESIAN_POINT('Ctrl Pts',(-1.11165616418,-36.7742356128,-0.989701314619));
#77226=CARTESIAN_POINT('Ctrl Pts',(-1.3921632233,-39.7742356128,-0.887346335547));
#77227=CARTESIAN_POINT('Ctrl Pts',(-1.3921632233,-36.7742356128,-0.887346335547));
#77228=CARTESIAN_POINT('Ctrl Pts',(-1.65990259641,-39.7742356128,-0.759470300753));
#77229=CARTESIAN_POINT('Ctrl Pts',(-1.65990259641,-36.7742356128,-0.759470300753));
#77230=CARTESIAN_POINT('Ctrl Pts',(-1.81552533939,-39.7742356128,-0.67135889116));
#77231=CARTESIAN_POINT('Ctrl Pts',(-1.81552533939,-36.7742356128,-0.67135889116));
#77232=CARTESIAN_POINT('Ctrl Pts',(-2.13001246648,-39.7742356128,-0.455784308931));
#77233=CARTESIAN_POINT('Ctrl Pts',(-2.13001246648,-36.7742356128,-0.455784308931));
#77234=CARTESIAN_POINT('Ctrl Pts',(-2.40225756964,-39.7742356128,-0.187376365848));
#77235=CARTESIAN_POINT('Ctrl Pts',(-2.40225756964,-36.7742356128,-0.187376365848));
#77236=CARTESIAN_POINT('Ctrl Pts',(-2.53491876149,-39.7742356128,-0.0306790811922));
#77237=CARTESIAN_POINT('Ctrl Pts',(-2.53491876149,-36.7742356128,-0.0306790811922));
#77238=CARTESIAN_POINT('Ctrl Pts',(-2.74588721076,-39.7742356128,0.250416153254));
#77239=CARTESIAN_POINT('Ctrl Pts',(-2.74588721076,-36.7742356128,0.250416153254));
#77240=CARTESIAN_POINT('Ctrl Pts',(-2.93290680803,-39.7742356128,0.545770364295));
#77241=CARTESIAN_POINT('Ctrl Pts',(-2.93290680803,-36.7742356128,0.545770364295));
#77242=CARTESIAN_POINT('Ctrl Pts',(-3.00715366555,-39.7742356128,0.670355528577));
#77243=CARTESIAN_POINT('Ctrl Pts',(-3.00715366555,-36.7742356128,0.670355528577));
#77244=CARTESIAN_POINT('Ctrl Pts',(-3.20108514097,-39.7742356128,1.0165930916));
#77245=CARTESIAN_POINT('Ctrl Pts',(-3.20108514097,-36.7742356128,1.0165930916));
#77246=CARTESIAN_POINT('Ctrl Pts',(-3.36887363395,-39.7742356128,1.37561285195));
#77247=CARTESIAN_POINT('Ctrl Pts',(-3.36887363395,-36.7742356128,1.37561285195));
#77248=CARTESIAN_POINT('Ctrl Pts',(-3.46527948246,-39.7742356128,1.60915269898));
#77249=CARTESIAN_POINT('Ctrl Pts',(-3.46527948246,-36.7742356128,1.60915269898));
#77250=CARTESIAN_POINT('Ctrl Pts',(-3.55147728822,-39.7742356128,1.84810892036));
#77251=CARTESIAN_POINT('Ctrl Pts',(-3.55147728822,-36.7742356128,1.84810892036));
#77252=CARTESIAN_POINT('Ctrl Pts',(-3.62746705121,-39.7742356128,2.09248151608));
#77253=CARTESIAN_POINT('Ctrl Pts',(-3.62746705121,-36.7742356128,2.09248151608));
#77254=CARTESIAN_POINT('Ctrl Pts',(7.07911993306,-39.7742356128,1.41233341424));
#77255=CARTESIAN_POINT('Ctrl Pts',(7.07911993306,-36.7742356128,1.41233341424));
#77256=CARTESIAN_POINT('Ctrl Pts',(7.03043912742,-39.7742356128,0.911971673481));
#77257=CARTESIAN_POINT('Ctrl Pts',(7.03043912742,-36.7742356128,0.911971673481));
#77258=CARTESIAN_POINT('Ctrl Pts',(6.93879090488,-39.7742356128,0.427451671407));
#77259=CARTESIAN_POINT('Ctrl Pts',(6.93879090488,-36.7742356128,0.427451671407));
#77260=CARTESIAN_POINT('Ctrl Pts',(6.79968866463,-39.7742356128,-0.0361534703089));
#77261=CARTESIAN_POINT('Ctrl Pts',(6.79968866463,-36.7742356128,-0.0361534703089));
#77262=CARTESIAN_POINT('Ctrl Pts',(6.4258973146,-39.7742356128,-0.894662603614));
#77263=CARTESIAN_POINT('Ctrl Pts',(6.4258973146,-36.7742356128,-0.894662603614));
#77264=CARTESIAN_POINT('Ctrl Pts',(5.86106085412,-39.7742356128,-1.62790491519));
#77265=CARTESIAN_POINT('Ctrl Pts',(5.86106085412,-36.7742356128,-1.62790491519));
#77266=CARTESIAN_POINT('Ctrl Pts',(5.53842443335,-39.7742356128,-1.95360958375));
#77267=CARTESIAN_POINT('Ctrl Pts',(5.53842443335,-36.7742356128,-1.95360958375));
#77268=CARTESIAN_POINT('Ctrl Pts',(4.98933040959,-39.7742356128,-2.39194593497));
#77269=CARTESIAN_POINT('Ctrl Pts',(4.98933040959,-36.7742356128,-2.39194593497));
#77270=CARTESIAN_POINT('Ctrl Pts',(4.36273333629,-39.7742356128,-2.74903878258));
#77271=CARTESIAN_POINT('Ctrl Pts',(4.36273333629,-36.7742356128,-2.74903878258));
#77272=CARTESIAN_POINT('Ctrl Pts',(4.14078300625,-39.7742356128,-2.86156599489));
#77273=CARTESIAN_POINT('Ctrl Pts',(4.14078300625,-36.7742356128,-2.86156599489));
#77274=CARTESIAN_POINT('Ctrl Pts',(3.91246466012,-39.7742356128,-2.96464616022));
#77275=CARTESIAN_POINT('Ctrl Pts',(3.91246466012,-36.7742356128,-2.96464616022));
#77276=CARTESIAN_POINT('Ctrl Pts',(3.67755401867,-39.7742356128,-3.05915055738));
#77277=CARTESIAN_POINT('Ctrl Pts',(3.67755401867,-36.7742356128,-3.05915055738));
#77278=CARTESIAN_POINT('',(3.67755401867,-37.2742356128,-3.05915055738));
#77279=CARTESIAN_POINT('',(3.67755401867,-39.6642356128,-3.05915055738));
#77280=CARTESIAN_POINT('',(7.07911993306,-37.2742356128,1.41233341424));
#77281=CARTESIAN_POINT('Ctrl Pts',(7.07911993306,-37.2742356128,1.41233341424));
#77282=CARTESIAN_POINT('Ctrl Pts',(7.03043912742,-37.2742356128,0.911971673481));
#77283=CARTESIAN_POINT('Ctrl Pts',(6.93879090488,-37.2742356128,0.427451671407));
#77284=CARTESIAN_POINT('Ctrl Pts',(6.79968866463,-37.2742356128,-0.0361534703089));
#77285=CARTESIAN_POINT('Ctrl Pts',(6.4258973146,-37.2742356128,-0.894662603614));
#77286=CARTESIAN_POINT('Ctrl Pts',(5.86106085412,-37.2742356128,-1.62790491519));
#77287=CARTESIAN_POINT('Ctrl Pts',(5.53842443335,-37.2742356128,-1.95360958375));
#77288=CARTESIAN_POINT('Ctrl Pts',(4.98933040959,-37.2742356128,-2.39194593497));
#77289=CARTESIAN_POINT('Ctrl Pts',(4.36273333629,-37.2742356128,-2.74903878258));
#77290=CARTESIAN_POINT('Ctrl Pts',(4.14078300625,-37.2742356128,-2.86156599489));
#77291=CARTESIAN_POINT('Ctrl Pts',(3.91246466012,-37.2742356128,-2.96464616022));
#77292=CARTESIAN_POINT('Ctrl Pts',(3.67755401867,-37.2742356128,-3.05915055738));
#77293=CARTESIAN_POINT('',(7.07911993306,-39.6642356128,1.41233341424));
#77294=CARTESIAN_POINT('Origin',(3.78952269078,-37.6642356128,-3.33747234321));
#77295=CARTESIAN_POINT('',(3.51985615629,-37.2742356128,-3.20601908088));
#77296=CARTESIAN_POINT('Origin',(3.78952269078,-37.2742356128,-3.33747234321));
#77297=CARTESIAN_POINT('',(3.51985615629,-39.6642356128,-3.20601908088));
#77298=CARTESIAN_POINT('Ctrl Pts',(3.51985615629,-39.7742356128,-3.20601908088));
#77299=CARTESIAN_POINT('Ctrl Pts',(3.51985615629,-36.7742356128,-3.20601908088));
#77300=CARTESIAN_POINT('Ctrl Pts',(3.35540949155,-39.7742356128,-3.54336911238));
#77301=CARTESIAN_POINT('Ctrl Pts',(3.35540949155,-36.7742356128,-3.54336911238));
#77302=CARTESIAN_POINT('Ctrl Pts',(3.15758359021,-39.7742356128,-3.85751660428));
#77303=CARTESIAN_POINT('Ctrl Pts',(3.15758359021,-36.7742356128,-3.85751660428));
#77304=CARTESIAN_POINT('Ctrl Pts',(2.92553217282,-39.7742356128,-4.14369667075));
#77305=CARTESIAN_POINT('Ctrl Pts',(2.92553217282,-36.7742356128,-4.14369667075));
#77306=CARTESIAN_POINT('Ctrl Pts',(2.54664760633,-39.7742356128,-4.50813716291));
#77307=CARTESIAN_POINT('Ctrl Pts',(2.54664760633,-36.7742356128,-4.50813716291));
#77308=CARTESIAN_POINT('Ctrl Pts',(2.10878664609,-39.7742356128,-4.80650592873));
#77309=CARTESIAN_POINT('Ctrl Pts',(2.10878664609,-36.7742356128,-4.80650592873));
#77310=CARTESIAN_POINT('Ctrl Pts',(1.97163547839,-39.7742356128,-4.89045414442));
#77311=CARTESIAN_POINT('Ctrl Pts',(1.97163547839,-36.7742356128,-4.89045414442));
#77312=CARTESIAN_POINT('Ctrl Pts',(1.8303523356,-39.7742356128,-4.96805050291));
#77313=CARTESIAN_POINT('Ctrl Pts',(1.8303523356,-36.7742356128,-4.96805050291));
#77314=CARTESIAN_POINT('Ctrl Pts',(1.68475792039,-39.7742356128,-5.03973467448));
#77315=CARTESIAN_POINT('Ctrl Pts',(1.68475792039,-36.7742356128,-5.03973467448));
#77316=CARTESIAN_POINT('',(1.68475792039,-37.2742356128,-5.03973467448));
#77317=CARTESIAN_POINT('',(1.68475792039,-39.6642356128,-5.03973467448));
#77318=CARTESIAN_POINT('Ctrl Pts',(3.51985615629,-37.2742356128,-3.20601908088));
#77319=CARTESIAN_POINT('Ctrl Pts',(3.35540949155,-37.2742356128,-3.54336911238));
#77320=CARTESIAN_POINT('Ctrl Pts',(3.15758359021,-37.2742356128,-3.85751660428));
#77321=CARTESIAN_POINT('Ctrl Pts',(2.92553217282,-37.2742356128,-4.14369667075));
#77322=CARTESIAN_POINT('Ctrl Pts',(2.54664760633,-37.2742356128,-4.50813716291));
#77323=CARTESIAN_POINT('Ctrl Pts',(2.10878664609,-37.2742356128,-4.80650592873));
#77324=CARTESIAN_POINT('Ctrl Pts',(1.97163547839,-37.2742356128,-4.89045414442));
#77325=CARTESIAN_POINT('Ctrl Pts',(1.8303523356,-37.2742356128,-4.96805050291));
#77326=CARTESIAN_POINT('Ctrl Pts',(1.68475792039,-37.2742356128,-5.03973467448));
#77327=CARTESIAN_POINT('Ctrl Pts',(7.21384189758,-39.7742356128,2.18958432614));
#77328=CARTESIAN_POINT('Ctrl Pts',(7.21384189758,-36.7742356128,2.18958432614));
#77329=CARTESIAN_POINT('Ctrl Pts',(7.13908599018,-39.7742356128,2.05065155888));
#77330=CARTESIAN_POINT('Ctrl Pts',(7.13908599018,-36.7742356128,2.05065155888));
#77331=CARTESIAN_POINT('Ctrl Pts',(7.08905059141,-39.7742356128,1.8984189694));
#77332=CARTESIAN_POINT('Ctrl Pts',(7.08905059141,-36.7742356128,1.8984189694));
#77333=CARTESIAN_POINT('Ctrl Pts',(7.1053290044,-39.7742356128,1.72681022597));
#77334=CARTESIAN_POINT('Ctrl Pts',(7.1053290044,-36.7742356128,1.72681022597));
#77335=CARTESIAN_POINT('Ctrl Pts',(7.09439724612,-39.7742356128,1.56936004643));
#77336=CARTESIAN_POINT('Ctrl Pts',(7.09439724612,-36.7742356128,1.56936004643));
#77337=CARTESIAN_POINT('Ctrl Pts',(7.07911993306,-39.7742356128,1.41233341424));
#77338=CARTESIAN_POINT('Ctrl Pts',(7.07911993306,-36.7742356128,1.41233341424));
#77339=CARTESIAN_POINT('',(7.21384189758,-37.2742356128,2.18958432614));
#77340=CARTESIAN_POINT('',(7.21384189758,-39.6642356128,2.18958432614));
#77341=CARTESIAN_POINT('Ctrl Pts',(7.21384189758,-37.2742356128,2.18958432614));
#77342=CARTESIAN_POINT('Ctrl Pts',(7.13908599018,-37.2742356128,2.05065155888));
#77343=CARTESIAN_POINT('Ctrl Pts',(7.08905059141,-37.2742356128,1.8984189694));
#77344=CARTESIAN_POINT('Ctrl Pts',(7.1053290044,-37.2742356128,1.72681022597));
#77345=CARTESIAN_POINT('Ctrl Pts',(7.09439724612,-37.2742356128,1.56936004643));
#77346=CARTESIAN_POINT('Ctrl Pts',(7.07911993306,-37.2742356128,1.41233341424));
#77347=CARTESIAN_POINT('Ctrl Pts',(8.75956299024,-39.7742356128,2.0634404101));
#77348=CARTESIAN_POINT('Ctrl Pts',(8.75956299024,-36.7742356128,2.0634404101));
#77349=CARTESIAN_POINT('Ctrl Pts',(8.67258032609,-39.7742356128,2.20595609378));
#77350=CARTESIAN_POINT('Ctrl Pts',(8.67258032609,-36.7742356128,2.20595609378));
#77351=CARTESIAN_POINT('Ctrl Pts',(8.57679326147,-39.7742356128,2.34786591099));
#77352=CARTESIAN_POINT('Ctrl Pts',(8.57679326147,-36.7742356128,2.34786591099));
#77353=CARTESIAN_POINT('Ctrl Pts',(8.46448329596,-39.7742356128,2.49604426586));
#77354=CARTESIAN_POINT('Ctrl Pts',(8.46448329596,-36.7742356128,2.49604426586));
#77355=CARTESIAN_POINT('Ctrl Pts',(8.27825186329,-39.7742356128,2.67220081215));
#77356=CARTESIAN_POINT('Ctrl Pts',(8.27825186329,-36.7742356128,2.67220081215));
#77357=CARTESIAN_POINT('Ctrl Pts',(8.05379939761,-39.7742356128,2.74035894609));
#77358=CARTESIAN_POINT('Ctrl Pts',(8.05379939761,-36.7742356128,2.74035894609));
#77359=CARTESIAN_POINT('Ctrl Pts',(7.9779370982,-39.7742356128,2.74765496713));
#77360=CARTESIAN_POINT('Ctrl Pts',(7.9779370982,-36.7742356128,2.74765496713));
#77361=CARTESIAN_POINT('Ctrl Pts',(7.82203636779,-39.7742356128,2.73225108729));
#77362=CARTESIAN_POINT('Ctrl Pts',(7.82203636779,-36.7742356128,2.73225108729));
#77363=CARTESIAN_POINT('Ctrl Pts',(7.67278421879,-39.7742356128,2.66639360485));
#77364=CARTESIAN_POINT('Ctrl Pts',(7.67278421879,-36.7742356128,2.66639360485));
#77365=CARTESIAN_POINT('Ctrl Pts',(7.59903734004,-39.7742356128,2.62164000818));
#77366=CARTESIAN_POINT('Ctrl Pts',(7.59903734004,-36.7742356128,2.62164000818));
#77367=CARTESIAN_POINT('Ctrl Pts',(7.46503014366,-39.7742356128,2.52047218586));
#77368=CARTESIAN_POINT('Ctrl Pts',(7.46503014366,-36.7742356128,2.52047218586));
#77369=CARTESIAN_POINT('Ctrl Pts',(7.35007323494,-39.7742356128,2.39634839519));
#77370=CARTESIAN_POINT('Ctrl Pts',(7.35007323494,-36.7742356128,2.39634839519));
#77371=CARTESIAN_POINT('Ctrl Pts',(7.29780025627,-39.7742356128,2.32993852802));
#77372=CARTESIAN_POINT('Ctrl Pts',(7.29780025627,-36.7742356128,2.32993852802));
#77373=CARTESIAN_POINT('Ctrl Pts',(7.25230657394,-39.7742356128,2.26107036804));
#77374=CARTESIAN_POINT('Ctrl Pts',(7.25230657394,-36.7742356128,2.26107036804));
#77375=CARTESIAN_POINT('Ctrl Pts',(7.21384189758,-39.7742356128,2.18958432614));
#77376=CARTESIAN_POINT('Ctrl Pts',(7.21384189758,-36.7742356128,2.18958432614));
#77377=CARTESIAN_POINT('',(8.75956299023,-37.2742356128,2.0634404101));
#77378=CARTESIAN_POINT('',(8.75956299024,-39.6642356128,2.0634404101));
#77379=CARTESIAN_POINT('Ctrl Pts',(8.75956299024,-37.2742356128,2.0634404101));
#77380=CARTESIAN_POINT('Ctrl Pts',(8.67258032609,-37.2742356128,2.20595609378));
#77381=CARTESIAN_POINT('Ctrl Pts',(8.57679326147,-37.2742356128,2.34786591099));
#77382=CARTESIAN_POINT('Ctrl Pts',(8.46448329596,-37.2742356128,2.49604426586));
#77383=CARTESIAN_POINT('Ctrl Pts',(8.27825186329,-37.2742356128,2.67220081215));
#77384=CARTESIAN_POINT('Ctrl Pts',(8.05379939761,-37.2742356128,2.74035894609));
#77385=CARTESIAN_POINT('Ctrl Pts',(7.9779370982,-37.2742356128,2.74765496713));
#77386=CARTESIAN_POINT('Ctrl Pts',(7.82203636779,-37.2742356128,2.73225108729));
#77387=CARTESIAN_POINT('Ctrl Pts',(7.67278421879,-37.2742356128,2.66639360485));
#77388=CARTESIAN_POINT('Ctrl Pts',(7.59903734004,-37.2742356128,2.62164000818));
#77389=CARTESIAN_POINT('Ctrl Pts',(7.46503014366,-37.2742356128,2.52047218586));
#77390=CARTESIAN_POINT('Ctrl Pts',(7.35007323494,-37.2742356128,2.39634839519));
#77391=CARTESIAN_POINT('Ctrl Pts',(7.29780025627,-37.2742356128,2.32993852802));
#77392=CARTESIAN_POINT('Ctrl Pts',(7.25230657394,-37.2742356128,2.26107036804));
#77393=CARTESIAN_POINT('Ctrl Pts',(7.21384189758,-37.2742356128,2.18958432614));
#77394=CARTESIAN_POINT('Ctrl Pts',(8.75956299023,-39.7742356128,2.0634404101));
#77395=CARTESIAN_POINT('Ctrl Pts',(8.75956299023,-36.7742356128,2.0634404101));
#77396=CARTESIAN_POINT('Ctrl Pts',(8.92890465395,-39.7742356128,1.78598462948));
#77397=CARTESIAN_POINT('Ctrl Pts',(8.92890465395,-36.7742356128,1.78598462948));
#77398=CARTESIAN_POINT('Ctrl Pts',(9.07290910839,-39.7742356128,1.49306491902));
#77399=CARTESIAN_POINT('Ctrl Pts',(9.07290910839,-36.7742356128,1.49306491902));
#77400=CARTESIAN_POINT('Ctrl Pts',(9.12674985892,-39.7742356128,1.15064933619));
#77401=CARTESIAN_POINT('Ctrl Pts',(9.12674985892,-36.7742356128,1.15064933619));
#77402=CARTESIAN_POINT('Ctrl Pts',(9.18664865847,-39.7742356128,0.831017278591));
#77403=CARTESIAN_POINT('Ctrl Pts',(9.18664865847,-36.7742356128,0.831017278591));
#77404=CARTESIAN_POINT('Ctrl Pts',(9.23698117862,-39.7742356128,0.509886547137));
#77405=CARTESIAN_POINT('Ctrl Pts',(9.23698117862,-36.7742356128,0.509886547137));
#77406=CARTESIAN_POINT('',(9.23698117862,-37.2742356128,0.509886547137));
#77407=CARTESIAN_POINT('Ctrl Pts',(8.75956299023,-37.2742356128,2.0634404101));
#77408=CARTESIAN_POINT('Ctrl Pts',(8.92890465395,-37.2742356128,1.78598462948));
#77409=CARTESIAN_POINT('Ctrl Pts',(9.07290910839,-37.2742356128,1.49306491902));
#77410=CARTESIAN_POINT('Ctrl Pts',(9.12674985892,-37.2742356128,1.15064933619));
#77411=CARTESIAN_POINT('Ctrl Pts',(9.18664865847,-37.2742356128,0.831017278591));
#77412=CARTESIAN_POINT('Ctrl Pts',(9.23698117862,-37.2742356128,0.509886547137));
#77413=CARTESIAN_POINT('',(9.23698117862,-39.6642356128,0.509886547137));
#77414=CARTESIAN_POINT('Ctrl Pts',(1.8704316098,-39.7742356128,-8.24476960846));
#77415=CARTESIAN_POINT('Ctrl Pts',(1.8704316098,-36.7742356128,-8.24476960846));
#77416=CARTESIAN_POINT('Ctrl Pts',(2.8184136576,-39.7742356128,-8.07409211621));
#77417=CARTESIAN_POINT('Ctrl Pts',(2.8184136576,-36.7742356128,-8.07409211621));
#77418=CARTESIAN_POINT('Ctrl Pts',(3.72902170056,-39.7742356128,-7.80028819978));
#77419=CARTESIAN_POINT('Ctrl Pts',(3.72902170056,-36.7742356128,-7.80028819978));
#77420=CARTESIAN_POINT('Ctrl Pts',(4.56766016636,-39.7742356128,-7.42304518879));
#77421=CARTESIAN_POINT('Ctrl Pts',(4.56766016636,-36.7742356128,-7.42304518879));
#77422=CARTESIAN_POINT('Ctrl Pts',(6.0885112091,-39.7742356128,-6.51001025629));
#77423=CARTESIAN_POINT('Ctrl Pts',(6.0885112091,-36.7742356128,-6.51001025629));
#77424=CARTESIAN_POINT('Ctrl Pts',(7.447100543,-39.7742356128,-5.31497212719));
#77425=CARTESIAN_POINT('Ctrl Pts',(7.447100543,-36.7742356128,-5.31497212719));
#77426=CARTESIAN_POINT('Ctrl Pts',(8.1250786803,-39.7742356128,-4.64371494659));
#77427=CARTESIAN_POINT('Ctrl Pts',(8.1250786803,-36.7742356128,-4.64371494659));
#77428=CARTESIAN_POINT('Ctrl Pts',(8.99226462924,-39.7742356128,-3.46343233105));
#77429=CARTESIAN_POINT('Ctrl Pts',(8.99226462924,-36.7742356128,-3.46343233105));
#77430=CARTESIAN_POINT('Ctrl Pts',(9.35827765375,-39.7742356128,-2.07942227767));
#77431=CARTESIAN_POINT('Ctrl Pts',(9.35827765375,-36.7742356128,-2.07942227767));
#77432=CARTESIAN_POINT('Ctrl Pts',(9.40334820731,-39.7742356128,-1.48595469944));
#77433=CARTESIAN_POINT('Ctrl Pts',(9.40334820731,-36.7742356128,-1.48595469944));
#77434=CARTESIAN_POINT('Ctrl Pts',(9.38724768323,-39.7742356128,-0.727182590117));
#77435=CARTESIAN_POINT('Ctrl Pts',(9.38724768323,-36.7742356128,-0.727182590117));
#77436=CARTESIAN_POINT('Ctrl Pts',(9.30567800741,-39.7742356128,0.0234614864805));
#77437=CARTESIAN_POINT('Ctrl Pts',(9.30567800741,-36.7742356128,0.0234614864805));
#77438=CARTESIAN_POINT('Ctrl Pts',(9.28522407236,-39.7742356128,0.186274742007));
#77439=CARTESIAN_POINT('Ctrl Pts',(9.28522407236,-36.7742356128,0.186274742007));
#77440=CARTESIAN_POINT('Ctrl Pts',(9.26229015361,-39.7742356128,0.348410633982));
#77441=CARTESIAN_POINT('Ctrl Pts',(9.26229015361,-36.7742356128,0.348410633982));
#77442=CARTESIAN_POINT('Ctrl Pts',(9.23698117862,-39.7742356128,0.509886547152));
#77443=CARTESIAN_POINT('Ctrl Pts',(9.23698117862,-36.7742356128,0.509886547152));
#77444=CARTESIAN_POINT('',(1.87043161062015,-37.2742356128,-8.24476960831419));
#77445=CARTESIAN_POINT('Ctrl Pts',(1.87043161102975,-37.2742356128,-8.24476960823859));
#77446=CARTESIAN_POINT('Ctrl Pts',(2.81841365854501,-37.2742356128,-8.07409211592585));
#77447=CARTESIAN_POINT('Ctrl Pts',(3.72902170121274,-37.2742356128,-7.80028819948638));
#77448=CARTESIAN_POINT('Ctrl Pts',(4.56766016677875,-37.2742356128,-7.42304518853861));
#77449=CARTESIAN_POINT('Ctrl Pts',(6.08851120928704,-37.2742356128,-6.51001025612548));
#77450=CARTESIAN_POINT('Ctrl Pts',(7.447100543,-37.2742356128,-5.31497212719));
#77451=CARTESIAN_POINT('Ctrl Pts',(8.1250786803,-37.2742356128,-4.64371494659));
#77452=CARTESIAN_POINT('Ctrl Pts',(8.99226462924,-37.2742356128,-3.46343233105));
#77453=CARTESIAN_POINT('Ctrl Pts',(9.35827765375,-37.2742356128,-2.07942227767));
#77454=CARTESIAN_POINT('Ctrl Pts',(9.40334820731,-37.2742356128,-1.48595469944));
#77455=CARTESIAN_POINT('Ctrl Pts',(9.38724768323,-37.2742356128,-0.727182590117));
#77456=CARTESIAN_POINT('Ctrl Pts',(9.30567800741,-37.2742356128,0.0234614864805));
#77457=CARTESIAN_POINT('Ctrl Pts',(9.28522407236,-37.2742356128,0.186274742007));
#77458=CARTESIAN_POINT('Ctrl Pts',(9.26229015361,-37.2742356128,0.348410633982));
#77459=CARTESIAN_POINT('Ctrl Pts',(9.23698117862229,-37.2742356128,0.509886547137359));
#77460=CARTESIAN_POINT('',(1.8704316098,-39.6642356128,-8.24476960846));
#77461=CARTESIAN_POINT('Origin',(1.81727342606,-37.6642356128,-7.9495168227));
#77462=CARTESIAN_POINT('',(1.51727342606,-37.2742356128,-7.9495168227));
#77463=CARTESIAN_POINT('Origin',(1.81727342606,-37.2742356128,-7.9495168227));
#77464=CARTESIAN_POINT('',(1.51727342606,-39.6642356128,-7.9495168227));
#77465=CARTESIAN_POINT('Origin',(1.51727342606,-39.2742356128,-5.3088808072));
#77466=CARTESIAN_POINT('',(1.51727342606,-37.2742356128,-5.3088808072));
#77467=CARTESIAN_POINT('',(1.51727342606,-37.2742356128,-6.62919881495));
#77468=CARTESIAN_POINT('',(1.51727342606,-38.5242356128,-5.3088808072));
#77469=CARTESIAN_POINT('Origin',(1.81727342606,-37.6642356128,-5.3088808072));
#77470=CARTESIAN_POINT('Origin',(1.81727342606,-37.2742356128,-5.3088808072));
#77471=CARTESIAN_POINT('Ctrl Pts',(-1.8704316098,-39.7742356128,-8.24476960846));
#77472=CARTESIAN_POINT('Ctrl Pts',(-1.8704316098,-36.7742356128,-8.24476960846));
#77473=CARTESIAN_POINT('Ctrl Pts',(-2.8184136576,-39.7742356128,-8.07409211621));
#77474=CARTESIAN_POINT('Ctrl Pts',(-2.8184136576,-36.7742356128,-8.07409211621));
#77475=CARTESIAN_POINT('Ctrl Pts',(-3.72902170056,-39.7742356128,-7.80028819978));
#77476=CARTESIAN_POINT('Ctrl Pts',(-3.72902170056,-36.7742356128,-7.80028819978));
#77477=CARTESIAN_POINT('Ctrl Pts',(-4.56766016636,-39.7742356128,-7.42304518879));
#77478=CARTESIAN_POINT('Ctrl Pts',(-4.56766016636,-36.7742356128,-7.42304518879));
#77479=CARTESIAN_POINT('Ctrl Pts',(-6.0885112091,-39.7742356128,-6.51001025629));
#77480=CARTESIAN_POINT('Ctrl Pts',(-6.0885112091,-36.7742356128,-6.51001025629));
#77481=CARTESIAN_POINT('Ctrl Pts',(-7.447100543,-39.7742356128,-5.31497212719));
#77482=CARTESIAN_POINT('Ctrl Pts',(-7.447100543,-36.7742356128,-5.31497212719));
#77483=CARTESIAN_POINT('Ctrl Pts',(-8.1250786803,-39.7742356128,-4.64371494659));
#77484=CARTESIAN_POINT('Ctrl Pts',(-8.1250786803,-36.7742356128,-4.64371494659));
#77485=CARTESIAN_POINT('Ctrl Pts',(-8.99226462924,-39.7742356128,-3.46343233105));
#77486=CARTESIAN_POINT('Ctrl Pts',(-8.99226462924,-36.7742356128,-3.46343233105));
#77487=CARTESIAN_POINT('Ctrl Pts',(-9.35827765375,-39.7742356128,-2.07942227767));
#77488=CARTESIAN_POINT('Ctrl Pts',(-9.35827765375,-36.7742356128,-2.07942227767));
#77489=CARTESIAN_POINT('Ctrl Pts',(-9.40334820731,-39.7742356128,-1.48595469944));
#77490=CARTESIAN_POINT('Ctrl Pts',(-9.40334820731,-36.7742356128,-1.48595469944));
#77491=CARTESIAN_POINT('Ctrl Pts',(-9.38724768323,-39.7742356128,-0.727182590117));
#77492=CARTESIAN_POINT('Ctrl Pts',(-9.38724768323,-36.7742356128,-0.727182590117));
#77493=CARTESIAN_POINT('Ctrl Pts',(-9.30567800741,-39.7742356128,0.0234614864805));
#77494=CARTESIAN_POINT('Ctrl Pts',(-9.30567800741,-36.7742356128,0.0234614864805));
#77495=CARTESIAN_POINT('Ctrl Pts',(-9.28522407236,-39.7742356128,0.186274742007));
#77496=CARTESIAN_POINT('Ctrl Pts',(-9.28522407236,-36.7742356128,0.186274742007));
#77497=CARTESIAN_POINT('Ctrl Pts',(-9.26229015361,-39.7742356128,0.348410633982));
#77498=CARTESIAN_POINT('Ctrl Pts',(-9.26229015361,-36.7742356128,0.348410633982));
#77499=CARTESIAN_POINT('Ctrl Pts',(-9.23698117862,-39.7742356128,0.509886547152));
#77500=CARTESIAN_POINT('Ctrl Pts',(-9.23698117862,-36.7742356128,0.509886547152));
#77501=CARTESIAN_POINT('',(-1.87043161062015,-37.2742356128,-8.24476960831419));
#77502=CARTESIAN_POINT('',(-9.23698117862,-37.2742356128,0.509886547152));
#77503=CARTESIAN_POINT('Ctrl Pts',(-1.87043161102975,-37.2742356128,-8.24476960823859));
#77504=CARTESIAN_POINT('Ctrl Pts',(-2.81841365854501,-37.2742356128,-8.07409211592585));
#77505=CARTESIAN_POINT('Ctrl Pts',(-3.72902170121274,-37.2742356128,-7.80028819948638));
#77506=CARTESIAN_POINT('Ctrl Pts',(-4.56766016677875,-37.2742356128,-7.42304518853861));
#77507=CARTESIAN_POINT('Ctrl Pts',(-6.08851120928704,-37.2742356128,-6.51001025612548));
#77508=CARTESIAN_POINT('Ctrl Pts',(-7.447100543,-37.2742356128,-5.31497212719));
#77509=CARTESIAN_POINT('Ctrl Pts',(-8.1250786803,-37.2742356128,-4.64371494659));
#77510=CARTESIAN_POINT('Ctrl Pts',(-8.99226462924,-37.2742356128,-3.46343233105));
#77511=CARTESIAN_POINT('Ctrl Pts',(-9.35827765375,-37.2742356128,-2.07942227767));
#77512=CARTESIAN_POINT('Ctrl Pts',(-9.40334820731,-37.2742356128,-1.48595469944));
#77513=CARTESIAN_POINT('Ctrl Pts',(-9.38724768323,-37.2742356128,-0.727182590117));
#77514=CARTESIAN_POINT('Ctrl Pts',(-9.30567800741,-37.2742356128,0.0234614864805));
#77515=CARTESIAN_POINT('Ctrl Pts',(-9.28522407236,-37.2742356128,0.186274742007));
#77516=CARTESIAN_POINT('Ctrl Pts',(-9.26229015361,-37.2742356128,0.348410633982));
#77517=CARTESIAN_POINT('Ctrl Pts',(-9.23698117862,-37.2742356128,0.509886547152));
#77518=CARTESIAN_POINT('',(-9.23698117862,-39.6642356128,0.509886547152));
#77519=CARTESIAN_POINT('',(-1.8704316098,-39.6642356128,-8.24476960846));
#77520=CARTESIAN_POINT('Ctrl Pts',(-3.51985615629,-39.7742356128,-3.20601908088));
#77521=CARTESIAN_POINT('Ctrl Pts',(-3.51985615629,-36.7742356128,-3.20601908088));
#77522=CARTESIAN_POINT('Ctrl Pts',(-3.35540949155,-39.7742356128,-3.54336911238));
#77523=CARTESIAN_POINT('Ctrl Pts',(-3.35540949155,-36.7742356128,-3.54336911238));
#77524=CARTESIAN_POINT('Ctrl Pts',(-3.15758359021,-39.7742356128,-3.85751660428));
#77525=CARTESIAN_POINT('Ctrl Pts',(-3.15758359021,-36.7742356128,-3.85751660428));
#77526=CARTESIAN_POINT('Ctrl Pts',(-2.92553217282,-39.7742356128,-4.14369667075));
#77527=CARTESIAN_POINT('Ctrl Pts',(-2.92553217282,-36.7742356128,-4.14369667075));
#77528=CARTESIAN_POINT('Ctrl Pts',(-2.54664760633,-39.7742356128,-4.50813716291));
#77529=CARTESIAN_POINT('Ctrl Pts',(-2.54664760633,-36.7742356128,-4.50813716291));
#77530=CARTESIAN_POINT('Ctrl Pts',(-2.10878664609,-39.7742356128,-4.80650592873));
#77531=CARTESIAN_POINT('Ctrl Pts',(-2.10878664609,-36.7742356128,-4.80650592873));
#77532=CARTESIAN_POINT('Ctrl Pts',(-1.97163547839,-39.7742356128,-4.89045414442));
#77533=CARTESIAN_POINT('Ctrl Pts',(-1.97163547839,-36.7742356128,-4.89045414442));
#77534=CARTESIAN_POINT('Ctrl Pts',(-1.8303523356,-39.7742356128,-4.96805050291));
#77535=CARTESIAN_POINT('Ctrl Pts',(-1.8303523356,-36.7742356128,-4.96805050291));
#77536=CARTESIAN_POINT('Ctrl Pts',(-1.68475792039,-39.7742356128,-5.03973467448));
#77537=CARTESIAN_POINT('Ctrl Pts',(-1.68475792039,-36.7742356128,-5.03973467448));
#77538=CARTESIAN_POINT('',(-3.51985615629,-37.2742356128,-3.20601908088));
#77539=CARTESIAN_POINT('',(-1.68475792039,-37.2742356128,-5.03973467448));
#77540=CARTESIAN_POINT('Ctrl Pts',(-3.51985615629,-37.2742356128,-3.20601908088));
#77541=CARTESIAN_POINT('Ctrl Pts',(-3.35540949155,-37.2742356128,-3.54336911238));
#77542=CARTESIAN_POINT('Ctrl Pts',(-3.15758359021,-37.2742356128,-3.85751660428));
#77543=CARTESIAN_POINT('Ctrl Pts',(-2.92553217282,-37.2742356128,-4.14369667075));
#77544=CARTESIAN_POINT('Ctrl Pts',(-2.54664760633,-37.2742356128,-4.50813716291));
#77545=CARTESIAN_POINT('Ctrl Pts',(-2.10878664609,-37.2742356128,-4.80650592873));
#77546=CARTESIAN_POINT('Ctrl Pts',(-1.97163547839,-37.2742356128,-4.89045414442));
#77547=CARTESIAN_POINT('Ctrl Pts',(-1.8303523356,-37.2742356128,-4.96805050291));
#77548=CARTESIAN_POINT('Ctrl Pts',(-1.68475792039,-37.2742356128,-5.03973467448));
#77549=CARTESIAN_POINT('',(-1.68475792039,-39.6642356128,-5.03973467448));
#77550=CARTESIAN_POINT('',(-3.51985615629,-39.6642356128,-3.20601908088));
#77551=CARTESIAN_POINT('Origin',(-1.81727342606,-37.6642356128,-5.3088808072));
#77552=CARTESIAN_POINT('',(-1.51727342606,-37.2742356128,-5.3088808072));
#77553=CARTESIAN_POINT('Origin',(-1.81727342606,-37.2742356128,-5.3088808072));
#77554=CARTESIAN_POINT('',(-1.51727342606,-39.6642356128,-5.3088808072));
#77555=CARTESIAN_POINT('Origin',(-1.51727342606,-39.2742356128,-5.3088808072));
#77556=CARTESIAN_POINT('',(-1.51727342606,-37.2742356128,-7.9495168227));
#77557=CARTESIAN_POINT('',(-1.51727342606,-37.2742356128,-6.62919881495));
#77558=CARTESIAN_POINT('',(-1.51727342606,-38.5242356128,-7.9495168227));
#77559=CARTESIAN_POINT('Origin',(-1.81727342606,-37.6642356128,-7.9495168227));
#77560=CARTESIAN_POINT('Origin',(-1.81727342606,-37.2742356128,-7.9495168227));
#77561=CARTESIAN_POINT('Origin',(-3.78952269078,-37.6642356128,-3.33747234321));
#77562=CARTESIAN_POINT('',(-3.67755401867,-37.2742356128,-3.05915055738));
#77563=CARTESIAN_POINT('Origin',(-3.78952269078,-37.2742356128,-3.33747234321));
#77564=CARTESIAN_POINT('',(-3.67755401867,-39.6642356128,-3.05915055738));
#77565=CARTESIAN_POINT('Ctrl Pts',(-7.07911993306,-39.7742356128,1.41233341424));
#77566=CARTESIAN_POINT('Ctrl Pts',(-7.07911993306,-36.7742356128,1.41233341424));
#77567=CARTESIAN_POINT('Ctrl Pts',(-7.03043912742,-39.7742356128,0.911971673481));
#77568=CARTESIAN_POINT('Ctrl Pts',(-7.03043912742,-36.7742356128,0.911971673481));
#77569=CARTESIAN_POINT('Ctrl Pts',(-6.93879090488,-39.7742356128,0.427451671407));
#77570=CARTESIAN_POINT('Ctrl Pts',(-6.93879090488,-36.7742356128,0.427451671407));
#77571=CARTESIAN_POINT('Ctrl Pts',(-6.79968866463,-39.7742356128,-0.0361534703089));
#77572=CARTESIAN_POINT('Ctrl Pts',(-6.79968866463,-36.7742356128,-0.0361534703089));
#77573=CARTESIAN_POINT('Ctrl Pts',(-6.4258973146,-39.7742356128,-0.894662603614));
#77574=CARTESIAN_POINT('Ctrl Pts',(-6.4258973146,-36.7742356128,-0.894662603614));
#77575=CARTESIAN_POINT('Ctrl Pts',(-5.86106085412,-39.7742356128,-1.62790491519));
#77576=CARTESIAN_POINT('Ctrl Pts',(-5.86106085412,-36.7742356128,-1.62790491519));
#77577=CARTESIAN_POINT('Ctrl Pts',(-5.53842443335,-39.7742356128,-1.95360958375));
#77578=CARTESIAN_POINT('Ctrl Pts',(-5.53842443335,-36.7742356128,-1.95360958375));
#77579=CARTESIAN_POINT('Ctrl Pts',(-4.98933040959,-39.7742356128,-2.39194593497));
#77580=CARTESIAN_POINT('Ctrl Pts',(-4.98933040959,-36.7742356128,-2.39194593497));
#77581=CARTESIAN_POINT('Ctrl Pts',(-4.36273333629,-39.7742356128,-2.74903878258));
#77582=CARTESIAN_POINT('Ctrl Pts',(-4.36273333629,-36.7742356128,-2.74903878258));
#77583=CARTESIAN_POINT('Ctrl Pts',(-4.14078300625,-39.7742356128,-2.86156599489));
#77584=CARTESIAN_POINT('Ctrl Pts',(-4.14078300625,-36.7742356128,-2.86156599489));
#77585=CARTESIAN_POINT('Ctrl Pts',(-3.91246466012,-39.7742356128,-2.96464616022));
#77586=CARTESIAN_POINT('Ctrl Pts',(-3.91246466012,-36.7742356128,-2.96464616022));
#77587=CARTESIAN_POINT('Ctrl Pts',(-3.67755401867,-39.7742356128,-3.05915055738));
#77588=CARTESIAN_POINT('Ctrl Pts',(-3.67755401867,-36.7742356128,-3.05915055738));
#77589=CARTESIAN_POINT('',(-7.07911993306,-37.2742356128,1.41233341424));
#77590=CARTESIAN_POINT('Ctrl Pts',(-7.07911993306,-37.2742356128,1.41233341424));
#77591=CARTESIAN_POINT('Ctrl Pts',(-7.03043912742,-37.2742356128,0.911971673481));
#77592=CARTESIAN_POINT('Ctrl Pts',(-6.93879090488,-37.2742356128,0.427451671407));
#77593=CARTESIAN_POINT('Ctrl Pts',(-6.79968866463,-37.2742356128,-0.0361534703089));
#77594=CARTESIAN_POINT('Ctrl Pts',(-6.4258973146,-37.2742356128,-0.894662603614));
#77595=CARTESIAN_POINT('Ctrl Pts',(-5.86106085412,-37.2742356128,-1.62790491519));
#77596=CARTESIAN_POINT('Ctrl Pts',(-5.53842443335,-37.2742356128,-1.95360958375));
#77597=CARTESIAN_POINT('Ctrl Pts',(-4.98933040959,-37.2742356128,-2.39194593497));
#77598=CARTESIAN_POINT('Ctrl Pts',(-4.36273333629,-37.2742356128,-2.74903878258));
#77599=CARTESIAN_POINT('Ctrl Pts',(-4.14078300625,-37.2742356128,-2.86156599489));
#77600=CARTESIAN_POINT('Ctrl Pts',(-3.91246466012,-37.2742356128,-2.96464616022));
#77601=CARTESIAN_POINT('Ctrl Pts',(-3.67755401867,-37.2742356128,-3.05915055738));
#77602=CARTESIAN_POINT('',(-7.07911993306,-39.6642356128,1.41233341424));
#77603=CARTESIAN_POINT('Ctrl Pts',(-8.75956299023,-39.7742356128,2.0634404101));
#77604=CARTESIAN_POINT('Ctrl Pts',(-8.75956299023,-36.7742356128,2.0634404101));
#77605=CARTESIAN_POINT('Ctrl Pts',(-8.92890465395,-39.7742356128,1.78598462948));
#77606=CARTESIAN_POINT('Ctrl Pts',(-8.92890465395,-36.7742356128,1.78598462948));
#77607=CARTESIAN_POINT('Ctrl Pts',(-9.07290910839,-39.7742356128,1.49306491902));
#77608=CARTESIAN_POINT('Ctrl Pts',(-9.07290910839,-36.7742356128,1.49306491902));
#77609=CARTESIAN_POINT('Ctrl Pts',(-9.12674985892,-39.7742356128,1.15064933619));
#77610=CARTESIAN_POINT('Ctrl Pts',(-9.12674985892,-36.7742356128,1.15064933619));
#77611=CARTESIAN_POINT('Ctrl Pts',(-9.18664865847,-39.7742356128,0.831017278591));
#77612=CARTESIAN_POINT('Ctrl Pts',(-9.18664865847,-36.7742356128,0.831017278591));
#77613=CARTESIAN_POINT('Ctrl Pts',(-9.23698117862,-39.7742356128,0.509886547137));
#77614=CARTESIAN_POINT('Ctrl Pts',(-9.23698117862,-36.7742356128,0.509886547137));
#77615=CARTESIAN_POINT('',(-8.75956299023,-37.2742356128,2.0634404101));
#77616=CARTESIAN_POINT('Ctrl Pts',(-8.75956299023,-37.2742356128,2.0634404101));
#77617=CARTESIAN_POINT('Ctrl Pts',(-8.92890465395,-37.2742356128,1.78598462948));
#77618=CARTESIAN_POINT('Ctrl Pts',(-9.07290910839,-37.2742356128,1.49306491902));
#77619=CARTESIAN_POINT('Ctrl Pts',(-9.12674985892,-37.2742356128,1.15064933619));
#77620=CARTESIAN_POINT('Ctrl Pts',(-9.18664865847,-37.2742356128,0.831017278591));
#77621=CARTESIAN_POINT('Ctrl Pts',(-9.23698117861771,-37.2742356128,0.509886547151641));
#77622=CARTESIAN_POINT('',(-8.75956299023,-39.6642356128,2.0634404101));
#77623=CARTESIAN_POINT('Ctrl Pts',(-8.75956299024,-39.7742356128,2.0634404101));
#77624=CARTESIAN_POINT('Ctrl Pts',(-8.75956299024,-36.7742356128,2.0634404101));
#77625=CARTESIAN_POINT('Ctrl Pts',(-8.67258032609,-39.7742356128,2.20595609378));
#77626=CARTESIAN_POINT('Ctrl Pts',(-8.67258032609,-36.7742356128,2.20595609378));
#77627=CARTESIAN_POINT('Ctrl Pts',(-8.57679326147,-39.7742356128,2.34786591099));
#77628=CARTESIAN_POINT('Ctrl Pts',(-8.57679326147,-36.7742356128,2.34786591099));
#77629=CARTESIAN_POINT('Ctrl Pts',(-8.46448329596,-39.7742356128,2.49604426586));
#77630=CARTESIAN_POINT('Ctrl Pts',(-8.46448329596,-36.7742356128,2.49604426586));
#77631=CARTESIAN_POINT('Ctrl Pts',(-8.27825186329,-39.7742356128,2.67220081215));
#77632=CARTESIAN_POINT('Ctrl Pts',(-8.27825186329,-36.7742356128,2.67220081215));
#77633=CARTESIAN_POINT('Ctrl Pts',(-8.05379939761,-39.7742356128,2.74035894609));
#77634=CARTESIAN_POINT('Ctrl Pts',(-8.05379939761,-36.7742356128,2.74035894609));
#77635=CARTESIAN_POINT('Ctrl Pts',(-7.9779370982,-39.7742356128,2.74765496713));
#77636=CARTESIAN_POINT('Ctrl Pts',(-7.9779370982,-36.7742356128,2.74765496713));
#77637=CARTESIAN_POINT('Ctrl Pts',(-7.82203636779,-39.7742356128,2.73225108729));
#77638=CARTESIAN_POINT('Ctrl Pts',(-7.82203636779,-36.7742356128,2.73225108729));
#77639=CARTESIAN_POINT('Ctrl Pts',(-7.67278421879,-39.7742356128,2.66639360485));
#77640=CARTESIAN_POINT('Ctrl Pts',(-7.67278421879,-36.7742356128,2.66639360485));
#77641=CARTESIAN_POINT('Ctrl Pts',(-7.59903734004,-39.7742356128,2.62164000818));
#77642=CARTESIAN_POINT('Ctrl Pts',(-7.59903734004,-36.7742356128,2.62164000818));
#77643=CARTESIAN_POINT('Ctrl Pts',(-7.46503014366,-39.7742356128,2.52047218586));
#77644=CARTESIAN_POINT('Ctrl Pts',(-7.46503014366,-36.7742356128,2.52047218586));
#77645=CARTESIAN_POINT('Ctrl Pts',(-7.35007323494,-39.7742356128,2.39634839519));
#77646=CARTESIAN_POINT('Ctrl Pts',(-7.35007323494,-36.7742356128,2.39634839519));
#77647=CARTESIAN_POINT('Ctrl Pts',(-7.29780025627,-39.7742356128,2.32993852802));
#77648=CARTESIAN_POINT('Ctrl Pts',(-7.29780025627,-36.7742356128,2.32993852802));
#77649=CARTESIAN_POINT('Ctrl Pts',(-7.25230657394,-39.7742356128,2.26107036804));
#77650=CARTESIAN_POINT('Ctrl Pts',(-7.25230657394,-36.7742356128,2.26107036804));
#77651=CARTESIAN_POINT('Ctrl Pts',(-7.21384189758,-39.7742356128,2.18958432614));
#77652=CARTESIAN_POINT('Ctrl Pts',(-7.21384189758,-36.7742356128,2.18958432614));
#77653=CARTESIAN_POINT('',(-7.21384189758,-37.2742356128,2.18958432614));
#77654=CARTESIAN_POINT('Ctrl Pts',(-8.75956299023,-37.2742356128,2.0634404101));
#77655=CARTESIAN_POINT('Ctrl Pts',(-8.67258032609,-37.2742356128,2.20595609378));
#77656=CARTESIAN_POINT('Ctrl Pts',(-8.57679326147,-37.2742356128,2.34786591099));
#77657=CARTESIAN_POINT('Ctrl Pts',(-8.46448329596,-37.2742356128,2.49604426586));
#77658=CARTESIAN_POINT('Ctrl Pts',(-8.27825186329,-37.2742356128,2.67220081215));
#77659=CARTESIAN_POINT('Ctrl Pts',(-8.05379939761,-37.2742356128,2.74035894609));
#77660=CARTESIAN_POINT('Ctrl Pts',(-7.9779370982,-37.2742356128,2.74765496713));
#77661=CARTESIAN_POINT('Ctrl Pts',(-7.82203636779,-37.2742356128,2.73225108729));
#77662=CARTESIAN_POINT('Ctrl Pts',(-7.67278421879,-37.2742356128,2.66639360485));
#77663=CARTESIAN_POINT('Ctrl Pts',(-7.59903734004,-37.2742356128,2.62164000818));
#77664=CARTESIAN_POINT('Ctrl Pts',(-7.46503014366,-37.2742356128,2.52047218586));
#77665=CARTESIAN_POINT('Ctrl Pts',(-7.35007323494,-37.2742356128,2.39634839519));
#77666=CARTESIAN_POINT('Ctrl Pts',(-7.29780025627,-37.2742356128,2.32993852802));
#77667=CARTESIAN_POINT('Ctrl Pts',(-7.25230657394,-37.2742356128,2.26107036804));
#77668=CARTESIAN_POINT('Ctrl Pts',(-7.21384189758,-37.2742356128,2.18958432614));
#77669=CARTESIAN_POINT('',(-7.21384189758,-39.6642356128,2.18958432614));
#77670=CARTESIAN_POINT('Ctrl Pts',(-7.21384189758,-39.7742356128,2.18958432614));
#77671=CARTESIAN_POINT('Ctrl Pts',(-7.21384189758,-36.7742356128,2.18958432614));
#77672=CARTESIAN_POINT('Ctrl Pts',(-7.13908599018,-39.7742356128,2.05065155888));
#77673=CARTESIAN_POINT('Ctrl Pts',(-7.13908599018,-36.7742356128,2.05065155888));
#77674=CARTESIAN_POINT('Ctrl Pts',(-7.08905059141,-39.7742356128,1.8984189694));
#77675=CARTESIAN_POINT('Ctrl Pts',(-7.08905059141,-36.7742356128,1.8984189694));
#77676=CARTESIAN_POINT('Ctrl Pts',(-7.1053290044,-39.7742356128,1.72681022597));
#77677=CARTESIAN_POINT('Ctrl Pts',(-7.1053290044,-36.7742356128,1.72681022597));
#77678=CARTESIAN_POINT('Ctrl Pts',(-7.09439724612,-39.7742356128,1.56936004643));
#77679=CARTESIAN_POINT('Ctrl Pts',(-7.09439724612,-36.7742356128,1.56936004643));
#77680=CARTESIAN_POINT('Ctrl Pts',(-7.07911993306,-39.7742356128,1.41233341424));
#77681=CARTESIAN_POINT('Ctrl Pts',(-7.07911993306,-36.7742356128,1.41233341424));
#77682=CARTESIAN_POINT('Ctrl Pts',(-7.21384189758,-37.2742356128,2.18958432614));
#77683=CARTESIAN_POINT('Ctrl Pts',(-7.13908599018,-37.2742356128,2.05065155888));
#77684=CARTESIAN_POINT('Ctrl Pts',(-7.08905059141,-37.2742356128,1.8984189694));
#77685=CARTESIAN_POINT('Ctrl Pts',(-7.1053290044,-37.2742356128,1.72681022597));
#77686=CARTESIAN_POINT('Ctrl Pts',(-7.09439724612,-37.2742356128,1.56936004643));
#77687=CARTESIAN_POINT('Ctrl Pts',(-7.07911993306,-37.2742356128,1.41233341424));
#77688=CARTESIAN_POINT('Ctrl Pts',(9.47221976654,-38.2742356128,2.49225909299));
#77689=CARTESIAN_POINT('Ctrl Pts',(9.47221976654,-37.0742356128,2.49225909299));
#77690=CARTESIAN_POINT('Ctrl Pts',(9.39947240551,-38.2742356128,2.61145111814));
#77691=CARTESIAN_POINT('Ctrl Pts',(9.39947240551,-37.0742356128,2.61145111814));
#77692=CARTESIAN_POINT('Ctrl Pts',(9.32101749845,-38.2742356128,2.73104611971));
#77693=CARTESIAN_POINT('Ctrl Pts',(9.32101749845,-37.0742356128,2.73104611971));
#77694=CARTESIAN_POINT('Ctrl Pts',(9.23447554945,-38.2742356128,2.85280836926));
#77695=CARTESIAN_POINT('Ctrl Pts',(9.23447554945,-37.0742356128,2.85280836926));
#77696=CARTESIAN_POINT('Ctrl Pts',(9.02906684789,-38.2742356128,3.10681559939));
#77697=CARTESIAN_POINT('Ctrl Pts',(9.02906684789,-37.0742356128,3.10681559939));
#77698=CARTESIAN_POINT('Ctrl Pts',(8.75253761634,-38.2742356128,3.33309151087));
#77699=CARTESIAN_POINT('Ctrl Pts',(8.75253761634,-37.0742356128,3.33309151087));
#77700=CARTESIAN_POINT('Ctrl Pts',(8.5879953064,-38.2742356128,3.43383230551));
#77701=CARTESIAN_POINT('Ctrl Pts',(8.5879953064,-37.0742356128,3.43383230551));
#77702=CARTESIAN_POINT('Ctrl Pts',(8.23034267354,-38.2742356128,3.56436456904));
#77703=CARTESIAN_POINT('Ctrl Pts',(8.23034267354,-37.0742356128,3.56436456904));
#77704=CARTESIAN_POINT('Ctrl Pts',(7.84867458413,-38.2742356128,3.56156543232));
#77705=CARTESIAN_POINT('Ctrl Pts',(7.84867458413,-37.0742356128,3.56156543232));
#77706=CARTESIAN_POINT('Ctrl Pts',(7.67119781066,-38.2742356128,3.52757441198));
#77707=CARTESIAN_POINT('Ctrl Pts',(7.67119781066,-37.0742356128,3.52757441198));
#77708=CARTESIAN_POINT('Ctrl Pts',(7.27066371621,-38.2742356128,3.38466568023));
#77709=CARTESIAN_POINT('Ctrl Pts',(7.27066371621,-37.0742356128,3.38466568023));
#77710=CARTESIAN_POINT('Ctrl Pts',(6.95203985001,-38.2742356128,3.13761299508));
#77711=CARTESIAN_POINT('Ctrl Pts',(6.95203985001,-37.0742356128,3.13761299508));
#77712=CARTESIAN_POINT('Ctrl Pts',(6.78734156337,-38.2742356128,2.96846990237));
#77713=CARTESIAN_POINT('Ctrl Pts',(6.78734156337,-37.0742356128,2.96846990237));
#77714=CARTESIAN_POINT('Ctrl Pts',(6.6484900876,-38.2742356128,2.78390759916));
#77715=CARTESIAN_POINT('Ctrl Pts',(6.6484900876,-37.0742356128,2.78390759916));
#77716=CARTESIAN_POINT('Ctrl Pts',(6.53914701908,-38.2742356128,2.5806950957));
#77717=CARTESIAN_POINT('Ctrl Pts',(6.53914701908,-37.0742356128,2.5806950957));
#77718=CARTESIAN_POINT('',(9.47221976654,-37.2742356128,2.49225909299));
#77719=CARTESIAN_POINT('',(9.47221976654,-37.6642356128,2.49225909299));
#77720=CARTESIAN_POINT('',(6.53914701908,-37.2742356128,2.5806950957));
#77721=CARTESIAN_POINT('Ctrl Pts',(9.47221976654,-37.2742356128,2.49225909299));
#77722=CARTESIAN_POINT('Ctrl Pts',(9.39947240551,-37.2742356128,2.61145111814));
#77723=CARTESIAN_POINT('Ctrl Pts',(9.32101749845,-37.2742356128,2.73104611971));
#77724=CARTESIAN_POINT('Ctrl Pts',(9.23447554945,-37.2742356128,2.85280836926));
#77725=CARTESIAN_POINT('Ctrl Pts',(9.02906684789,-37.2742356128,3.10681559939));
#77726=CARTESIAN_POINT('Ctrl Pts',(8.75253761634,-37.2742356128,3.33309151087));
#77727=CARTESIAN_POINT('Ctrl Pts',(8.5879953064,-37.2742356128,3.43383230551));
#77728=CARTESIAN_POINT('Ctrl Pts',(8.23034267354,-37.2742356128,3.56436456904));
#77729=CARTESIAN_POINT('Ctrl Pts',(7.84867458413,-37.2742356128,3.56156543232));
#77730=CARTESIAN_POINT('Ctrl Pts',(7.67119781066,-37.2742356128,3.52757441198));
#77731=CARTESIAN_POINT('Ctrl Pts',(7.27066371621,-37.2742356128,3.38466568023));
#77732=CARTESIAN_POINT('Ctrl Pts',(6.95203985001,-37.2742356128,3.13761299508));
#77733=CARTESIAN_POINT('Ctrl Pts',(6.78734156337,-37.2742356128,2.96846990237));
#77734=CARTESIAN_POINT('Ctrl Pts',(6.6484900876,-37.2742356128,2.78390759916));
#77735=CARTESIAN_POINT('Ctrl Pts',(6.53914701908,-37.2742356128,2.5806950957));
#77736=CARTESIAN_POINT('',(6.53914701908,-37.6642356128,2.5806950957));
#77737=CARTESIAN_POINT('Ctrl Pts',(6.53914701908,-38.2742356128,2.5806950957));
#77738=CARTESIAN_POINT('Ctrl Pts',(6.53914701908,-37.0742356128,2.5806950957));
#77739=CARTESIAN_POINT('Ctrl Pts',(5.92921620253,-38.2742356128,1.44714753899));
#77740=CARTESIAN_POINT('Ctrl Pts',(5.92921620253,-37.0742356128,1.44714753899));
#77741=CARTESIAN_POINT('Ctrl Pts',(6.2734552887,-38.2742356128,-0.199812643821));
#77742=CARTESIAN_POINT('Ctrl Pts',(6.2734552887,-37.0742356128,-0.199812643821));
#77743=CARTESIAN_POINT('Ctrl Pts',(4.66846608736,-38.2742356128,-1.09094389297));
#77744=CARTESIAN_POINT('Ctrl Pts',(4.66846608736,-37.0742356128,-1.09094389297));
#77745=CARTESIAN_POINT('Ctrl Pts',(3.58890539941,-38.2742356128,-1.81984798791));
#77746=CARTESIAN_POINT('Ctrl Pts',(3.58890539941,-37.0742356128,-1.81984798791));
#77747=CARTESIAN_POINT('Ctrl Pts',(2.42434411094,-38.2742356128,-2.36824808793));
#77748=CARTESIAN_POINT('Ctrl Pts',(2.42434411094,-37.0742356128,-2.36824808793));
#77749=CARTESIAN_POINT('',(2.42434411094,-37.2742356128,-2.36824808793));
#77750=CARTESIAN_POINT('Ctrl Pts',(6.53914701908,-37.2742356128,2.5806950957));
#77751=CARTESIAN_POINT('Ctrl Pts',(5.92921620253,-37.2742356128,1.44714753899));
#77752=CARTESIAN_POINT('Ctrl Pts',(6.2734552887,-37.2742356128,-0.199812643821));
#77753=CARTESIAN_POINT('Ctrl Pts',(4.66846608736,-37.2742356128,-1.09094389297));
#77754=CARTESIAN_POINT('Ctrl Pts',(3.58890539941,-37.2742356128,-1.81984798791));
#77755=CARTESIAN_POINT('Ctrl Pts',(2.42434411094,-37.2742356128,-2.36824808793));
#77756=CARTESIAN_POINT('',(2.42434411094,-37.6642356128,-2.36824808793));
#77757=CARTESIAN_POINT('Origin',(6.28286804938E-15,-37.6642356128,2.77999550541));
#77758=CARTESIAN_POINT('',(1.11895565834,-37.2742356128,-2.79941259037));
#77759=CARTESIAN_POINT('Origin',(6.28286804938E-15,-37.2742356128,2.77999550541));
#77760=CARTESIAN_POINT('',(1.11895565834,-37.6642356128,-2.79941259037));
#77761=CARTESIAN_POINT('Origin',(1.21727342606,-38.2742356128,-3.28965091665));
#77762=CARTESIAN_POINT('',(0.717273426056,-37.2742356128,-3.28965091665));
#77763=CARTESIAN_POINT('',(0.717273426056,-38.2742356128,-3.28965091665));
#77764=CARTESIAN_POINT('Origin',(1.21727342606,-37.2742356128,-3.28965091665));
#77765=CARTESIAN_POINT('Origin',(0.717273426056,-39.2742356128,-2.86512409447));
#77766=CARTESIAN_POINT('',(0.717273426055,-37.2742356128,-7.9495168227));
#77767=CARTESIAN_POINT('',(0.717273426056,-37.2742356128,-5.61958386968));
#77768=CARTESIAN_POINT('',(0.717273426056,-37.7742356128,-7.9495168227));
#77769=CARTESIAN_POINT('Origin',(1.81725567298,-37.6642356128,-7.94326730652));
#77770=CARTESIAN_POINT('',(2.02820898725,-37.2742356128,-9.02284995699));
#77771=CARTESIAN_POINT('',(2.02820898725,-37.6642356128,-9.02284995699));
#77772=CARTESIAN_POINT('Origin',(1.81725567298,-37.2742356128,-7.94326730652));
#77773=CARTESIAN_POINT('Origin',(2.60353620801,-38.2742356128,-11.9671662765));
#77774=CARTESIAN_POINT('',(2.06575948168,-37.2742356128,-9.01576047707));
#77775=CARTESIAN_POINT('Origin',(2.60353620801,-37.2742356128,-11.9671662765));
#77776=CARTESIAN_POINT('',(2.06575948168,-38.2742356128,-9.01576047707));
#77777=CARTESIAN_POINT('Ctrl Pts',(2.06575946829,-38.2742356128,-9.01576047951));
#77778=CARTESIAN_POINT('Ctrl Pts',(2.06575946829,-37.0742356128,-9.01576047951));
#77779=CARTESIAN_POINT('Ctrl Pts',(2.9672194554,-38.2742356128,-8.85150512783));
#77780=CARTESIAN_POINT('Ctrl Pts',(2.9672194554,-37.0742356128,-8.85150512783));
#77781=CARTESIAN_POINT('Ctrl Pts',(3.84599034531,-38.2742356128,-8.59864711683));
#77782=CARTESIAN_POINT('Ctrl Pts',(3.84599034531,-37.0742356128,-8.59864711683));
#77783=CARTESIAN_POINT('Ctrl Pts',(4.67357601438,-38.2742356128,-8.25401331235));
#77784=CARTESIAN_POINT('Ctrl Pts',(4.67357601438,-37.0742356128,-8.25401331235));
#77785=CARTESIAN_POINT('Ctrl Pts',(6.17345275231,-38.2742356128,-7.42645694938));
#77786=CARTESIAN_POINT('Ctrl Pts',(6.17345275231,-37.0742356128,-7.42645694938));
#77787=CARTESIAN_POINT('Ctrl Pts',(7.5161640814,-38.2742356128,-6.34532321195));
#77788=CARTESIAN_POINT('Ctrl Pts',(7.5161640814,-37.0742356128,-6.34532321195));
#77789=CARTESIAN_POINT('Ctrl Pts',(8.15806093588,-38.2742356128,-5.76170299258));
#77790=CARTESIAN_POINT('Ctrl Pts',(8.15806093588,-37.0742356128,-5.76170299258));
#77791=CARTESIAN_POINT('Ctrl Pts',(9.14108523272,-38.2742356128,-4.69984607968));
#77792=CARTESIAN_POINT('Ctrl Pts',(9.14108523272,-37.0742356128,-4.69984607968));
#77793=CARTESIAN_POINT('Ctrl Pts',(9.81302959348,-38.2742356128,-3.42961050122));
#77794=CARTESIAN_POINT('Ctrl Pts',(9.81302959348,-37.0742356128,-3.42961050122));
#77795=CARTESIAN_POINT('Ctrl Pts',(10.0098671635,-38.2742356128,-2.88411398337));
#77796=CARTESIAN_POINT('Ctrl Pts',(10.0098671635,-37.0742356128,-2.88411398337));
#77797=CARTESIAN_POINT('Ctrl Pts',(10.222733632,-38.2742356128,-1.82926592992));
#77798=CARTESIAN_POINT('Ctrl Pts',(10.222733632,-37.0742356128,-1.82926592992));
#77799=CARTESIAN_POINT('Ctrl Pts',(10.2199521215,-38.2742356128,-0.771812654558));
#77800=CARTESIAN_POINT('Ctrl Pts',(10.2199521215,-37.0742356128,-0.771812654558));
#77801=CARTESIAN_POINT('Ctrl Pts',(10.184046519,-38.2742356128,-0.287190507733));
#77802=CARTESIAN_POINT('Ctrl Pts',(10.184046519,-37.0742356128,-0.287190507733));
#77803=CARTESIAN_POINT('Ctrl Pts',(10.1298079404,-38.2742356128,0.182098137249));
#77804=CARTESIAN_POINT('Ctrl Pts',(10.1298079404,-37.0742356128,0.182098137249));
#77805=CARTESIAN_POINT('Ctrl Pts',(10.0571285787,-38.2742356128,0.645805825733));
#77806=CARTESIAN_POINT('Ctrl Pts',(10.0571285787,-37.0742356128,0.645805825733));
#77807=CARTESIAN_POINT('',(10.0571285787,-37.2742356128,0.645805825719));
#77808=CARTESIAN_POINT('Ctrl Pts',(2.06575948168004,-37.2742356128,-9.0157604770702));
#77809=CARTESIAN_POINT('Ctrl Pts',(2.96721946584242,-37.2742356128,-8.8515051248253));
#77810=CARTESIAN_POINT('Ctrl Pts',(3.84599035268564,-37.2742356128,-8.59864711375854));
#77811=CARTESIAN_POINT('Ctrl Pts',(4.67357601907077,-37.2742356128,-8.25401330976187));
#77812=CARTESIAN_POINT('Ctrl Pts',(6.17345275440962,-37.2742356128,-7.42645694768941));
#77813=CARTESIAN_POINT('Ctrl Pts',(7.5161640814,-37.2742356128,-6.34532321195));
#77814=CARTESIAN_POINT('Ctrl Pts',(8.15806093588,-37.2742356128,-5.76170299258));
#77815=CARTESIAN_POINT('Ctrl Pts',(9.14108523272,-37.2742356128,-4.69984607968));
#77816=CARTESIAN_POINT('Ctrl Pts',(9.81302959348,-37.2742356128,-3.42961050122));
#77817=CARTESIAN_POINT('Ctrl Pts',(10.0098671635,-37.2742356128,-2.88411398337));
#77818=CARTESIAN_POINT('Ctrl Pts',(10.222733632,-37.2742356128,-1.82926592992));
#77819=CARTESIAN_POINT('Ctrl Pts',(10.2199521215,-37.2742356128,-0.771812654558));
#77820=CARTESIAN_POINT('Ctrl Pts',(10.184046519,-37.2742356128,-0.287190507733));
#77821=CARTESIAN_POINT('Ctrl Pts',(10.1298079404,-37.2742356128,0.182098137249));
#77822=CARTESIAN_POINT('Ctrl Pts',(10.0571285787022,-37.2742356128,0.645805825719337));
#77823=CARTESIAN_POINT('',(10.0571285787,-37.6642356128,0.645805825719));
#77824=CARTESIAN_POINT('Ctrl Pts',(9.47221976654,-38.2742356128,2.49225909299));
#77825=CARTESIAN_POINT('Ctrl Pts',(9.47221976654,-37.0742356128,2.49225909299));
#77826=CARTESIAN_POINT('Ctrl Pts',(9.54575444005,-38.2742356128,2.3717771053));
#77827=CARTESIAN_POINT('Ctrl Pts',(9.54575444005,-37.0742356128,2.3717771053));
#77828=CARTESIAN_POINT('Ctrl Pts',(9.61961951766,-38.2742356128,2.24151541202));
#77829=CARTESIAN_POINT('Ctrl Pts',(9.61961951766,-37.0742356128,2.24151541202));
#77830=CARTESIAN_POINT('Ctrl Pts',(9.68609489427,-38.2742356128,2.10542437124));
#77831=CARTESIAN_POINT('Ctrl Pts',(9.68609489427,-37.0742356128,2.10542437124));
#77832=CARTESIAN_POINT('Ctrl Pts',(9.84457330898,-38.2742356128,1.72211870919));
#77833=CARTESIAN_POINT('Ctrl Pts',(9.84457330898,-37.0742356128,1.72211870919));
#77834=CARTESIAN_POINT('Ctrl Pts',(9.94207621049,-38.2742356128,1.33157301839));
#77835=CARTESIAN_POINT('Ctrl Pts',(9.94207621049,-37.0742356128,1.33157301839));
#77836=CARTESIAN_POINT('Ctrl Pts',(9.98299011243,-38.2742356128,1.0898271634));
#77837=CARTESIAN_POINT('Ctrl Pts',(9.98299011243,-37.0742356128,1.0898271634));
#77838=CARTESIAN_POINT('Ctrl Pts',(10.0216701384,-38.2742356128,0.872037193625));
#77839=CARTESIAN_POINT('Ctrl Pts',(10.0216701384,-37.0742356128,0.872037193625));
#77840=CARTESIAN_POINT('Ctrl Pts',(10.0571285787,-38.2742356128,0.645805825719));
#77841=CARTESIAN_POINT('Ctrl Pts',(10.0571285787,-37.0742356128,0.645805825719));
#77842=CARTESIAN_POINT('Ctrl Pts',(9.47221976654,-37.2742356128,2.49225909299));
#77843=CARTESIAN_POINT('Ctrl Pts',(9.54575444005,-37.2742356128,2.3717771053));
#77844=CARTESIAN_POINT('Ctrl Pts',(9.61961951766,-37.2742356128,2.24151541202));
#77845=CARTESIAN_POINT('Ctrl Pts',(9.68609489427,-37.2742356128,2.10542437124));
#77846=CARTESIAN_POINT('Ctrl Pts',(9.84457330898,-37.2742356128,1.72211870919));
#77847=CARTESIAN_POINT('Ctrl Pts',(9.94207621049,-37.2742356128,1.33157301839));
#77848=CARTESIAN_POINT('Ctrl Pts',(9.98299011243,-37.2742356128,1.0898271634));
#77849=CARTESIAN_POINT('Ctrl Pts',(10.0216701384,-37.2742356128,0.872037193625));
#77850=CARTESIAN_POINT('Ctrl Pts',(10.0571285787,-37.2742356128,0.645805825719));
#77851=CARTESIAN_POINT('Ctrl Pts',(-5.2400559546,-38.2742356128,5.59690998219));
#77852=CARTESIAN_POINT('Ctrl Pts',(-5.2400559546,-37.0742356128,5.59690998219));
#77853=CARTESIAN_POINT('Ctrl Pts',(-5.25990082634,-38.2742356128,5.0059883748));
#77854=CARTESIAN_POINT('Ctrl Pts',(-5.25990082634,-37.0742356128,5.0059883748));
#77855=CARTESIAN_POINT('Ctrl Pts',(-5.23061607717,-38.2742356128,4.36229648927));
#77856=CARTESIAN_POINT('Ctrl Pts',(-5.23061607717,-37.0742356128,4.36229648927));
#77857=CARTESIAN_POINT('Ctrl Pts',(-5.00490058958,-38.2742356128,3.77298874453));
#77858=CARTESIAN_POINT('Ctrl Pts',(-5.00490058958,-37.0742356128,3.77298874453));
#77859=CARTESIAN_POINT('Ctrl Pts',(-4.75506448705,-38.2742356128,3.08655684628));
#77860=CARTESIAN_POINT('Ctrl Pts',(-4.75506448705,-37.0742356128,3.08655684628));
#77861=CARTESIAN_POINT('Ctrl Pts',(-4.54755634075,-38.2742356128,2.39287258614));
#77862=CARTESIAN_POINT('Ctrl Pts',(-4.54755634075,-37.0742356128,2.39287258614));
#77863=CARTESIAN_POINT('Ctrl Pts',(-4.4987250478,-38.2742356128,2.21955031284));
#77864=CARTESIAN_POINT('Ctrl Pts',(-4.4987250478,-37.0742356128,2.21955031284));
#77865=CARTESIAN_POINT('Ctrl Pts',(-4.44893332626,-38.2742356128,2.04003858973));
#77866=CARTESIAN_POINT('Ctrl Pts',(-4.44893332626,-37.0742356128,2.04003858973));
#77867=CARTESIAN_POINT('Ctrl Pts',(-4.39152710765,-38.2742356128,1.85538989834));
#77868=CARTESIAN_POINT('Ctrl Pts',(-4.39152710765,-37.0742356128,1.85538989834));
#77869=CARTESIAN_POINT('',(-4.39152710765,-37.6642356128,1.85538989834));
#77870=CARTESIAN_POINT('',(-5.2400559546,-37.6642356128,5.59690998219));
#77871=CARTESIAN_POINT('Ctrl Pts',(-0.605290084206,-38.2742356128,-1.95105924441));
#77872=CARTESIAN_POINT('Ctrl Pts',(-0.605290084206,-37.0742356128,-1.95105924441));
#77873=CARTESIAN_POINT('Ctrl Pts',(-0.774096521679,-38.2742356128,-1.91628513625));
#77874=CARTESIAN_POINT('Ctrl Pts',(-0.774096521679,-37.0742356128,-1.91628513625));
#77875=CARTESIAN_POINT('Ctrl Pts',(-0.942624183674,-38.2742356128,-1.87619510128));
#77876=CARTESIAN_POINT('Ctrl Pts',(-0.942624183674,-37.0742356128,-1.87619510128));
#77877=CARTESIAN_POINT('Ctrl Pts',(-1.11061388614,-38.2742356128,-1.83037525603));
#77878=CARTESIAN_POINT('Ctrl Pts',(-1.11061388614,-37.0742356128,-1.83037525603));
#77879=CARTESIAN_POINT('Ctrl Pts',(-1.74274860628,-38.2742356128,-1.63293852912));
#77880=CARTESIAN_POINT('Ctrl Pts',(-1.74274860628,-37.0742356128,-1.63293852912));
#77881=CARTESIAN_POINT('Ctrl Pts',(-2.34679547467,-38.2742356128,-1.33257881069));
#77882=CARTESIAN_POINT('Ctrl Pts',(-2.34679547467,-37.0742356128,-1.33257881069));
#77883=CARTESIAN_POINT('Ctrl Pts',(-2.73083933763,-38.2742356128,-1.04090474176));
#77884=CARTESIAN_POINT('Ctrl Pts',(-2.73083933763,-37.0742356128,-1.04090474176));
#77885=CARTESIAN_POINT('Ctrl Pts',(-3.39638296129,-38.2742356128,-0.293897533174));
#77886=CARTESIAN_POINT('Ctrl Pts',(-3.39638296129,-37.0742356128,-0.293897533174));
#77887=CARTESIAN_POINT('Ctrl Pts',(-3.86916001537,-38.2742356128,0.542814468562));
#77888=CARTESIAN_POINT('Ctrl Pts',(-3.86916001537,-37.0742356128,0.542814468562));
#77889=CARTESIAN_POINT('Ctrl Pts',(-4.06911877342,-38.2742356128,0.942104314053));
#77890=CARTESIAN_POINT('Ctrl Pts',(-4.06911877342,-37.0742356128,0.942104314053));
#77891=CARTESIAN_POINT('Ctrl Pts',(-4.24744781279,-38.2742356128,1.39201586348));
#77892=CARTESIAN_POINT('Ctrl Pts',(-4.24744781279,-37.0742356128,1.39201586348));
#77893=CARTESIAN_POINT('Ctrl Pts',(-4.39143626207,-38.2742356128,1.85509771049));
#77894=CARTESIAN_POINT('Ctrl Pts',(-4.39143626207,-37.0742356128,1.85509771049));
#77895=CARTESIAN_POINT('Ctrl Pts',(-4.39145443226365,-38.2742356128,1.85515614772492));
#77896=CARTESIAN_POINT('Ctrl Pts',(-4.39145443226365,-37.0742356128,1.85515614772492));
#77897=CARTESIAN_POINT('Ctrl Pts',(-4.3914726024573,-38.2742356128,1.85521458495984));
#77898=CARTESIAN_POINT('Ctrl Pts',(-4.3914726024573,-37.0742356128,1.85521458495984));
#77899=CARTESIAN_POINT('Ctrl Pts',(-4.39149077265095,-38.2742356128,1.85527302219476));
#77900=CARTESIAN_POINT('Ctrl Pts',(-4.39149077265095,-37.0742356128,1.85527302219476));
#77901=CARTESIAN_POINT('Ctrl Pts',(-4.3915089428446,-38.2742356128,1.85533145942968));
#77902=CARTESIAN_POINT('Ctrl Pts',(-4.3915089428446,-37.0742356128,1.85533145942968));
#77903=CARTESIAN_POINT('Ctrl Pts',(-4.39152711303826,-38.2742356128,1.8553898966646));
#77904=CARTESIAN_POINT('Ctrl Pts',(-4.39152711303826,-37.0742356128,1.8553898966646));
#77905=CARTESIAN_POINT('',(-0.605290084208,-37.6642356128,-1.95105924441));
#77906=CARTESIAN_POINT('Origin',(1.44440015504E-13,-38.2742356128,0.987243652491));
#77907=CARTESIAN_POINT('',(0.605290084208,-38.2742356128,-1.95105924441));
#77908=CARTESIAN_POINT('Ctrl Pts',(0.605290084206,-38.2742356128,-1.95105924441));
#77909=CARTESIAN_POINT('Ctrl Pts',(0.605290084206,-37.0742356128,-1.95105924441));
#77910=CARTESIAN_POINT('Ctrl Pts',(0.774096521679,-38.2742356128,-1.91628513625));
#77911=CARTESIAN_POINT('Ctrl Pts',(0.774096521679,-37.0742356128,-1.91628513625));
#77912=CARTESIAN_POINT('Ctrl Pts',(0.942624183674,-38.2742356128,-1.87619510128));
#77913=CARTESIAN_POINT('Ctrl Pts',(0.942624183674,-37.0742356128,-1.87619510128));
#77914=CARTESIAN_POINT('Ctrl Pts',(1.11061388614,-38.2742356128,-1.83037525603));
#77915=CARTESIAN_POINT('Ctrl Pts',(1.11061388614,-37.0742356128,-1.83037525603));
#77916=CARTESIAN_POINT('Ctrl Pts',(1.74274860628,-38.2742356128,-1.63293852912));
#77917=CARTESIAN_POINT('Ctrl Pts',(1.74274860628,-37.0742356128,-1.63293852912));
#77918=CARTESIAN_POINT('Ctrl Pts',(2.34679547467,-38.2742356128,-1.33257881069));
#77919=CARTESIAN_POINT('Ctrl Pts',(2.34679547467,-37.0742356128,-1.33257881069));
#77920=CARTESIAN_POINT('Ctrl Pts',(2.73083933763,-38.2742356128,-1.04090474176));
#77921=CARTESIAN_POINT('Ctrl Pts',(2.73083933763,-37.0742356128,-1.04090474176));
#77922=CARTESIAN_POINT('Ctrl Pts',(3.39635927668,-38.2742356128,-0.29392411682));
#77923=CARTESIAN_POINT('Ctrl Pts',(3.39635927668,-37.0742356128,-0.29392411682));
#77924=CARTESIAN_POINT('Ctrl Pts',(3.86912636582,-38.2742356128,0.542754916759));
#77925=CARTESIAN_POINT('Ctrl Pts',(3.86912636582,-37.0742356128,0.542754916759));
#77926=CARTESIAN_POINT('Ctrl Pts',(4.06899942193,-38.2742356128,0.941795900815));
#77927=CARTESIAN_POINT('Ctrl Pts',(4.06899942193,-37.0742356128,0.941795900815));
#77928=CARTESIAN_POINT('Ctrl Pts',(4.2473975181,-38.2742356128,1.39188897252));
#77929=CARTESIAN_POINT('Ctrl Pts',(4.2473975181,-37.0742356128,1.39188897252));
#77930=CARTESIAN_POINT('Ctrl Pts',(4.39138551009,-38.2742356128,1.854934493));
#77931=CARTESIAN_POINT('Ctrl Pts',(4.39138551009,-37.0742356128,1.854934493));
#77932=CARTESIAN_POINT('',(4.39138551009,-37.6642356128,1.854934493));
#77933=CARTESIAN_POINT('Ctrl Pts',(5.2400559546,-38.2742356128,5.59690998219));
#77934=CARTESIAN_POINT('Ctrl Pts',(5.2400559546,-37.0742356128,5.59690998219));
#77935=CARTESIAN_POINT('Ctrl Pts',(5.25990082634,-38.2742356128,5.0059883748));
#77936=CARTESIAN_POINT('Ctrl Pts',(5.25990082634,-37.0742356128,5.0059883748));
#77937=CARTESIAN_POINT('Ctrl Pts',(5.23061607717,-38.2742356128,4.36229648927));
#77938=CARTESIAN_POINT('Ctrl Pts',(5.23061607717,-37.0742356128,4.36229648927));
#77939=CARTESIAN_POINT('Ctrl Pts',(5.00490058958,-38.2742356128,3.77298874453));
#77940=CARTESIAN_POINT('Ctrl Pts',(5.00490058958,-37.0742356128,3.77298874453));
#77941=CARTESIAN_POINT('Ctrl Pts',(4.75506448705,-38.2742356128,3.08655684628));
#77942=CARTESIAN_POINT('Ctrl Pts',(4.75506448705,-37.0742356128,3.08655684628));
#77943=CARTESIAN_POINT('Ctrl Pts',(4.54755634075,-38.2742356128,2.39287258614));
#77944=CARTESIAN_POINT('Ctrl Pts',(4.54755634075,-37.0742356128,2.39287258614));
#77945=CARTESIAN_POINT('Ctrl Pts',(4.4987250478,-38.2742356128,2.21955031284));
#77946=CARTESIAN_POINT('Ctrl Pts',(4.4987250478,-37.0742356128,2.21955031284));
#77947=CARTESIAN_POINT('Ctrl Pts',(4.44893332626,-38.2742356128,2.04003858973));
#77948=CARTESIAN_POINT('Ctrl Pts',(4.44893332626,-37.0742356128,2.04003858973));
#77949=CARTESIAN_POINT('Ctrl Pts',(4.39152710765,-38.2742356128,1.85538989834));
#77950=CARTESIAN_POINT('Ctrl Pts',(4.39152710765,-37.0742356128,1.85538989834));
#77951=CARTESIAN_POINT('Ctrl Pts',(4.3914987908103,-38.2742356128,1.8552988164412));
#77952=CARTESIAN_POINT('Ctrl Pts',(4.3914987908103,-37.0742356128,1.8552988164412));
#77953=CARTESIAN_POINT('Ctrl Pts',(4.39147047397061,-38.2742356128001,1.85520773454239));
#77954=CARTESIAN_POINT('Ctrl Pts',(4.39147047397061,-37.0742356128,1.85520773454239));
#77955=CARTESIAN_POINT('Ctrl Pts',(4.39144215713091,-38.2742356128001,1.85511665264359));
#77956=CARTESIAN_POINT('Ctrl Pts',(4.39144215713091,-37.0742356128,1.85511665264359));
#77957=CARTESIAN_POINT('Ctrl Pts',(4.39141384029122,-38.2742356128001,1.85502557074478));
#77958=CARTESIAN_POINT('Ctrl Pts',(4.39141384029122,-37.0742356128,1.85502557074478));
#77959=CARTESIAN_POINT('Ctrl Pts',(4.39138552345152,-38.2742356128001,1.85493448884598));
#77960=CARTESIAN_POINT('Ctrl Pts',(4.39138552345152,-37.0742356128,1.85493448884598));
#77961=CARTESIAN_POINT('',(5.2400559546,-37.6642356128,5.59690998219));
#77962=CARTESIAN_POINT('Origin',(-0.000416107150126,-37.6642356128,5.42091963994));
#77963=CARTESIAN_POINT('',(-7.34769233304E-15,-37.6642356128,10.664345987));
#77964=CARTESIAN_POINT('Origin',(0.000416107150126,-37.6642356128,5.42091963994));
#77965=CARTESIAN_POINT('Origin',(-2.60353620801,-38.2742356128,-11.9671662765));
#77966=CARTESIAN_POINT('',(-2.02820898725,-37.2742356128,-9.02284995699));
#77967=CARTESIAN_POINT('',(-2.06575948168,-37.2742356128,-9.01576047707));
#77968=CARTESIAN_POINT('Origin',(-2.60353620801,-37.2742356128,-11.9671662765));
#77969=CARTESIAN_POINT('',(-2.02820898726,-38.2742356128,-9.02284995699));
#77970=CARTESIAN_POINT('',(-2.06575948168,-38.2742356128,-9.01576047707));
#77971=CARTESIAN_POINT('Origin',(-1.81725567298,-37.6642356128,-7.94326730652));
#77972=CARTESIAN_POINT('',(-0.717273426055,-37.2742356128,-7.9495168227));
#77973=CARTESIAN_POINT('Origin',(-1.81725567298,-37.2742356128,-7.94326730652));
#77974=CARTESIAN_POINT('',(-0.717273426055,-37.6642356128,-7.9495168227));
#77975=CARTESIAN_POINT('Origin',(-0.717273426056,-39.2742356128,-2.86512409447));
#77976=CARTESIAN_POINT('',(-0.717273426056,-37.2742356128,-3.28965091665));
#77977=CARTESIAN_POINT('',(-0.717273426056,-37.2742356128,-5.61958386968));
#77978=CARTESIAN_POINT('',(-0.717273426056,-37.7742356128,-3.28965091665));
#77979=CARTESIAN_POINT('Origin',(-1.21727342606,-38.2742356128,-3.28965091665));
#77980=CARTESIAN_POINT('',(-1.11895565834,-37.2742356128,-2.79941259037));
#77981=CARTESIAN_POINT('Origin',(-1.21727342606,-37.2742356128,-3.28965091665));
#77982=CARTESIAN_POINT('',(-1.11895565834,-38.2742356128,-2.79941259037));
#77983=CARTESIAN_POINT('Origin',(-6.28286804938E-15,-37.6642356128,2.77999550541));
#77984=CARTESIAN_POINT('',(-2.42434411094,-37.2742356128,-2.36824808793));
#77985=CARTESIAN_POINT('Origin',(-6.28286804938E-15,-37.2742356128,2.77999550541));
#77986=CARTESIAN_POINT('',(-2.42434411094,-37.6642356128,-2.36824808793));
#77987=CARTESIAN_POINT('Ctrl Pts',(-6.53914701908,-38.2742356128,2.5806950957));
#77988=CARTESIAN_POINT('Ctrl Pts',(-6.53914701908,-37.0742356128,2.5806950957));
#77989=CARTESIAN_POINT('Ctrl Pts',(-5.92921620253,-38.2742356128,1.44714753899));
#77990=CARTESIAN_POINT('Ctrl Pts',(-5.92921620253,-37.0742356128,1.44714753899));
#77991=CARTESIAN_POINT('Ctrl Pts',(-6.2734552887,-38.2742356128,-0.199812643821));
#77992=CARTESIAN_POINT('Ctrl Pts',(-6.2734552887,-37.0742356128,-0.199812643821));
#77993=CARTESIAN_POINT('Ctrl Pts',(-4.66846608736,-38.2742356128,-1.09094389297));
#77994=CARTESIAN_POINT('Ctrl Pts',(-4.66846608736,-37.0742356128,-1.09094389297));
#77995=CARTESIAN_POINT('Ctrl Pts',(-3.58890539941,-38.2742356128,-1.81984798791));
#77996=CARTESIAN_POINT('Ctrl Pts',(-3.58890539941,-37.0742356128,-1.81984798791));
#77997=CARTESIAN_POINT('Ctrl Pts',(-2.42434411094,-38.2742356128,-2.36824808793));
#77998=CARTESIAN_POINT('Ctrl Pts',(-2.42434411094,-37.0742356128,-2.36824808793));
#77999=CARTESIAN_POINT('',(-6.53914701908,-37.2742356128,2.5806950957));
#78000=CARTESIAN_POINT('Ctrl Pts',(-6.53914701908,-37.2742356128,2.5806950957));
#78001=CARTESIAN_POINT('Ctrl Pts',(-5.92921620253,-37.2742356128,1.44714753899));
#78002=CARTESIAN_POINT('Ctrl Pts',(-6.2734552887,-37.2742356128,-0.199812643821));
#78003=CARTESIAN_POINT('Ctrl Pts',(-4.66846608736,-37.2742356128,-1.09094389297));
#78004=CARTESIAN_POINT('Ctrl Pts',(-3.58890539941,-37.2742356128,-1.81984798791));
#78005=CARTESIAN_POINT('Ctrl Pts',(-2.42434411094,-37.2742356128,-2.36824808793));
#78006=CARTESIAN_POINT('',(-6.53914701908,-37.6642356128,2.5806950957));
#78007=CARTESIAN_POINT('Ctrl Pts',(-9.47221976654,-38.2742356128,2.49225909299));
#78008=CARTESIAN_POINT('Ctrl Pts',(-9.47221976654,-37.0742356128,2.49225909299));
#78009=CARTESIAN_POINT('Ctrl Pts',(-9.39947240551,-38.2742356128,2.61145111814));
#78010=CARTESIAN_POINT('Ctrl Pts',(-9.39947240551,-37.0742356128,2.61145111814));
#78011=CARTESIAN_POINT('Ctrl Pts',(-9.32101749845,-38.2742356128,2.73104611971));
#78012=CARTESIAN_POINT('Ctrl Pts',(-9.32101749845,-37.0742356128,2.73104611971));
#78013=CARTESIAN_POINT('Ctrl Pts',(-9.23447554945,-38.2742356128,2.85280836926));
#78014=CARTESIAN_POINT('Ctrl Pts',(-9.23447554945,-37.0742356128,2.85280836926));
#78015=CARTESIAN_POINT('Ctrl Pts',(-9.02906684789,-38.2742356128,3.10681559939));
#78016=CARTESIAN_POINT('Ctrl Pts',(-9.02906684789,-37.0742356128,3.10681559939));
#78017=CARTESIAN_POINT('Ctrl Pts',(-8.75253761634,-38.2742356128,3.33309151087));
#78018=CARTESIAN_POINT('Ctrl Pts',(-8.75253761634,-37.0742356128,3.33309151087));
#78019=CARTESIAN_POINT('Ctrl Pts',(-8.5879953064,-38.2742356128,3.43383230551));
#78020=CARTESIAN_POINT('Ctrl Pts',(-8.5879953064,-37.0742356128,3.43383230551));
#78021=CARTESIAN_POINT('Ctrl Pts',(-8.23034267354,-38.2742356128,3.56436456904));
#78022=CARTESIAN_POINT('Ctrl Pts',(-8.23034267354,-37.0742356128,3.56436456904));
#78023=CARTESIAN_POINT('Ctrl Pts',(-7.84867458413,-38.2742356128,3.56156543232));
#78024=CARTESIAN_POINT('Ctrl Pts',(-7.84867458413,-37.0742356128,3.56156543232));
#78025=CARTESIAN_POINT('Ctrl Pts',(-7.67119781066,-38.2742356128,3.52757441198));
#78026=CARTESIAN_POINT('Ctrl Pts',(-7.67119781066,-37.0742356128,3.52757441198));
#78027=CARTESIAN_POINT('Ctrl Pts',(-7.27066371621,-38.2742356128,3.38466568023));
#78028=CARTESIAN_POINT('Ctrl Pts',(-7.27066371621,-37.0742356128,3.38466568023));
#78029=CARTESIAN_POINT('Ctrl Pts',(-6.95203985001,-38.2742356128,3.13761299508));
#78030=CARTESIAN_POINT('Ctrl Pts',(-6.95203985001,-37.0742356128,3.13761299508));
#78031=CARTESIAN_POINT('Ctrl Pts',(-6.78734156337,-38.2742356128,2.96846990237));
#78032=CARTESIAN_POINT('Ctrl Pts',(-6.78734156337,-37.0742356128,2.96846990237));
#78033=CARTESIAN_POINT('Ctrl Pts',(-6.6484900876,-38.2742356128,2.78390759916));
#78034=CARTESIAN_POINT('Ctrl Pts',(-6.6484900876,-37.0742356128,2.78390759916));
#78035=CARTESIAN_POINT('Ctrl Pts',(-6.53914701908,-38.2742356128,2.5806950957));
#78036=CARTESIAN_POINT('Ctrl Pts',(-6.53914701908,-37.0742356128,2.5806950957));
#78037=CARTESIAN_POINT('',(-9.47221976654,-37.2742356128,2.49225909299));
#78038=CARTESIAN_POINT('Ctrl Pts',(-9.47221976654,-37.2742356128,2.49225909299));
#78039=CARTESIAN_POINT('Ctrl Pts',(-9.39947240551,-37.2742356128,2.61145111814));
#78040=CARTESIAN_POINT('Ctrl Pts',(-9.32101749845,-37.2742356128,2.73104611971));
#78041=CARTESIAN_POINT('Ctrl Pts',(-9.23447554945,-37.2742356128,2.85280836926));
#78042=CARTESIAN_POINT('Ctrl Pts',(-9.02906684789,-37.2742356128,3.10681559939));
#78043=CARTESIAN_POINT('Ctrl Pts',(-8.75253761634,-37.2742356128,3.33309151087));
#78044=CARTESIAN_POINT('Ctrl Pts',(-8.5879953064,-37.2742356128,3.43383230551));
#78045=CARTESIAN_POINT('Ctrl Pts',(-8.23034267354,-37.2742356128,3.56436456904));
#78046=CARTESIAN_POINT('Ctrl Pts',(-7.84867458413,-37.2742356128,3.56156543232));
#78047=CARTESIAN_POINT('Ctrl Pts',(-7.67119781066,-37.2742356128,3.52757441198));
#78048=CARTESIAN_POINT('Ctrl Pts',(-7.27066371621,-37.2742356128,3.38466568023));
#78049=CARTESIAN_POINT('Ctrl Pts',(-6.95203985001,-37.2742356128,3.13761299508));
#78050=CARTESIAN_POINT('Ctrl Pts',(-6.78734156337,-37.2742356128,2.96846990237));
#78051=CARTESIAN_POINT('Ctrl Pts',(-6.6484900876,-37.2742356128,2.78390759916));
#78052=CARTESIAN_POINT('Ctrl Pts',(-6.53914701908,-37.2742356128,2.5806950957));
#78053=CARTESIAN_POINT('',(-9.47221976654,-37.6642356128,2.49225909299));
#78054=CARTESIAN_POINT('Ctrl Pts',(-9.47221976654,-38.2742356128,2.49225909299));
#78055=CARTESIAN_POINT('Ctrl Pts',(-9.47221976654,-37.0742356128,2.49225909299));
#78056=CARTESIAN_POINT('Ctrl Pts',(-9.54575444005,-38.2742356128,2.3717771053));
#78057=CARTESIAN_POINT('Ctrl Pts',(-9.54575444005,-37.0742356128,2.3717771053));
#78058=CARTESIAN_POINT('Ctrl Pts',(-9.61961951766,-38.2742356128,2.24151541202));
#78059=CARTESIAN_POINT('Ctrl Pts',(-9.61961951766,-37.0742356128,2.24151541202));
#78060=CARTESIAN_POINT('Ctrl Pts',(-9.68609489427,-38.2742356128,2.10542437124));
#78061=CARTESIAN_POINT('Ctrl Pts',(-9.68609489427,-37.0742356128,2.10542437124));
#78062=CARTESIAN_POINT('Ctrl Pts',(-9.84457330898,-38.2742356128,1.72211870919));
#78063=CARTESIAN_POINT('Ctrl Pts',(-9.84457330898,-37.0742356128,1.72211870919));
#78064=CARTESIAN_POINT('Ctrl Pts',(-9.94207621049,-38.2742356128,1.33157301839));
#78065=CARTESIAN_POINT('Ctrl Pts',(-9.94207621049,-37.0742356128,1.33157301839));
#78066=CARTESIAN_POINT('Ctrl Pts',(-9.98299011243,-38.2742356128,1.0898271634));
#78067=CARTESIAN_POINT('Ctrl Pts',(-9.98299011243,-37.0742356128,1.0898271634));
#78068=CARTESIAN_POINT('Ctrl Pts',(-10.0216701384,-38.2742356128,0.872037193625));
#78069=CARTESIAN_POINT('Ctrl Pts',(-10.0216701384,-37.0742356128,0.872037193625));
#78070=CARTESIAN_POINT('Ctrl Pts',(-10.0571285787,-38.2742356128,0.645805825719));
#78071=CARTESIAN_POINT('Ctrl Pts',(-10.0571285787,-37.0742356128,0.645805825719));
#78072=CARTESIAN_POINT('',(-10.0571285787,-37.2742356128,0.645805825719));
#78073=CARTESIAN_POINT('Ctrl Pts',(-9.47221976654,-37.2742356128,2.49225909299));
#78074=CARTESIAN_POINT('Ctrl Pts',(-9.54575444005,-37.2742356128,2.3717771053));
#78075=CARTESIAN_POINT('Ctrl Pts',(-9.61961951766,-37.2742356128,2.24151541202));
#78076=CARTESIAN_POINT('Ctrl Pts',(-9.68609489427,-37.2742356128,2.10542437124));
#78077=CARTESIAN_POINT('Ctrl Pts',(-9.84457330898,-37.2742356128,1.72211870919));
#78078=CARTESIAN_POINT('Ctrl Pts',(-9.94207621049,-37.2742356128,1.33157301839));
#78079=CARTESIAN_POINT('Ctrl Pts',(-9.98299011243,-37.2742356128,1.0898271634));
#78080=CARTESIAN_POINT('Ctrl Pts',(-10.0216701384,-37.2742356128,0.872037193625));
#78081=CARTESIAN_POINT('Ctrl Pts',(-10.0571285787,-37.2742356128,0.645805825719));
#78082=CARTESIAN_POINT('',(-10.0571285787,-37.6642356128,0.645805825719));
#78083=CARTESIAN_POINT('Ctrl Pts',(-2.06575946829,-38.2742356128,-9.01576047951));
#78084=CARTESIAN_POINT('Ctrl Pts',(-2.06575946829,-37.0742356128,-9.01576047951));
#78085=CARTESIAN_POINT('Ctrl Pts',(-2.9672194554,-38.2742356128,-8.85150512783));
#78086=CARTESIAN_POINT('Ctrl Pts',(-2.9672194554,-37.0742356128,-8.85150512783));
#78087=CARTESIAN_POINT('Ctrl Pts',(-3.84599034531,-38.2742356128,-8.59864711683));
#78088=CARTESIAN_POINT('Ctrl Pts',(-3.84599034531,-37.0742356128,-8.59864711683));
#78089=CARTESIAN_POINT('Ctrl Pts',(-4.67357601438,-38.2742356128,-8.25401331235));
#78090=CARTESIAN_POINT('Ctrl Pts',(-4.67357601438,-37.0742356128,-8.25401331235));
#78091=CARTESIAN_POINT('Ctrl Pts',(-6.17345275231,-38.2742356128,-7.42645694938));
#78092=CARTESIAN_POINT('Ctrl Pts',(-6.17345275231,-37.0742356128,-7.42645694938));
#78093=CARTESIAN_POINT('Ctrl Pts',(-7.5161640814,-38.2742356128,-6.34532321195));
#78094=CARTESIAN_POINT('Ctrl Pts',(-7.5161640814,-37.0742356128,-6.34532321195));
#78095=CARTESIAN_POINT('Ctrl Pts',(-8.15806093588,-38.2742356128,-5.76170299258));
#78096=CARTESIAN_POINT('Ctrl Pts',(-8.15806093588,-37.0742356128,-5.76170299258));
#78097=CARTESIAN_POINT('Ctrl Pts',(-9.14108523272,-38.2742356128,-4.69984607968));
#78098=CARTESIAN_POINT('Ctrl Pts',(-9.14108523272,-37.0742356128,-4.69984607968));
#78099=CARTESIAN_POINT('Ctrl Pts',(-9.81302959348,-38.2742356128,-3.42961050122));
#78100=CARTESIAN_POINT('Ctrl Pts',(-9.81302959348,-37.0742356128,-3.42961050122));
#78101=CARTESIAN_POINT('Ctrl Pts',(-10.0098671635,-38.2742356128,-2.88411398337));
#78102=CARTESIAN_POINT('Ctrl Pts',(-10.0098671635,-37.0742356128,-2.88411398337));
#78103=CARTESIAN_POINT('Ctrl Pts',(-10.222733632,-38.2742356128,-1.82926592992));
#78104=CARTESIAN_POINT('Ctrl Pts',(-10.222733632,-37.0742356128,-1.82926592992));
#78105=CARTESIAN_POINT('Ctrl Pts',(-10.2199521215,-38.2742356128,-0.771812654558));
#78106=CARTESIAN_POINT('Ctrl Pts',(-10.2199521215,-37.0742356128,-0.771812654558));
#78107=CARTESIAN_POINT('Ctrl Pts',(-10.184046519,-38.2742356128,-0.287190507733));
#78108=CARTESIAN_POINT('Ctrl Pts',(-10.184046519,-37.0742356128,-0.287190507733));
#78109=CARTESIAN_POINT('Ctrl Pts',(-10.1298079404,-38.2742356128,0.182098137249));
#78110=CARTESIAN_POINT('Ctrl Pts',(-10.1298079404,-37.0742356128,0.182098137249));
#78111=CARTESIAN_POINT('Ctrl Pts',(-10.0571285787,-38.2742356128,0.645805825733));
#78112=CARTESIAN_POINT('Ctrl Pts',(-10.0571285787,-37.0742356128,0.645805825733));
#78113=CARTESIAN_POINT('Ctrl Pts',(-2.06575948168004,-37.2742356128,-9.0157604770702));
#78114=CARTESIAN_POINT('Ctrl Pts',(-2.96721946584242,-37.2742356128,-8.8515051248253));
#78115=CARTESIAN_POINT('Ctrl Pts',(-3.84599035268564,-37.2742356128,-8.59864711375854));
#78116=CARTESIAN_POINT('Ctrl Pts',(-4.67357601907077,-37.2742356128,-8.25401330976187));
#78117=CARTESIAN_POINT('Ctrl Pts',(-6.17345275440962,-37.2742356128,-7.42645694768941));
#78118=CARTESIAN_POINT('Ctrl Pts',(-7.5161640814,-37.2742356128,-6.34532321195));
#78119=CARTESIAN_POINT('Ctrl Pts',(-8.15806093588,-37.2742356128,-5.76170299258));
#78120=CARTESIAN_POINT('Ctrl Pts',(-9.14108523272,-37.2742356128,-4.69984607968));
#78121=CARTESIAN_POINT('Ctrl Pts',(-9.81302959348,-37.2742356128,-3.42961050122));
#78122=CARTESIAN_POINT('Ctrl Pts',(-10.0098671635,-37.2742356128,-2.88411398337));
#78123=CARTESIAN_POINT('Ctrl Pts',(-10.222733632,-37.2742356128,-1.82926592992));
#78124=CARTESIAN_POINT('Ctrl Pts',(-10.2199521215,-37.2742356128,-0.771812654558));
#78125=CARTESIAN_POINT('Ctrl Pts',(-10.184046519,-37.2742356128,-0.287190507733));
#78126=CARTESIAN_POINT('Ctrl Pts',(-10.1298079404,-37.2742356128,0.182098137249));
#78127=CARTESIAN_POINT('Ctrl Pts',(-10.0571285787022,-37.2742356128,0.645805825719337));
#78128=CARTESIAN_POINT('Origin',(-3.35265884719E-30,-37.2742356128,3.15283103411E-22));
#78129=CARTESIAN_POINT('Origin',(-3.35265884719E-30,-37.2742356128,3.15283103411E-22));
#78130=CARTESIAN_POINT('Origin',(0.5,-41.6742356128,13.1643460036));
#78131=CARTESIAN_POINT('',(0.5,-37.2742356128,13.9192139476));
#78132=CARTESIAN_POINT('Origin',(-0.5,-41.6742356128,13.1643460036));
#78133=CARTESIAN_POINT('',(-0.5,-37.2742356128,13.9192139476));
#78134=CARTESIAN_POINT('Origin',(0.5,-41.6742356128,13.1643460036));
#78135=CARTESIAN_POINT('',(0.5,-37.2742356128,-13.2046742098));
#78136=CARTESIAN_POINT('Origin',(-0.5,-41.6742356128,13.1643460036));
#78137=CARTESIAN_POINT('',(-0.5,-37.2742356128,-13.2046742098));
#78138=CARTESIAN_POINT('Origin',(-10.9208700025,-38.7742356128,-8.61474463077));
#78139=CARTESIAN_POINT('',(-11.7961681305,-33.7742356128,-9.46800252678));
#78140=CARTESIAN_POINT('',(-11.7961681305,-36.2742356128,-9.46800252678));
#78141=CARTESIAN_POINT('',(-10.9208700025,-33.7742356128,-8.61474463077));
#78142=CARTESIAN_POINT('',(-11.3585190665,-33.7742356128,-9.04137357878));
#78143=CARTESIAN_POINT('',(-10.9208700025,-37.2742356128,-8.61474463077));
#78144=CARTESIAN_POINT('',(-10.9208700025,-35.5242356128,-8.61474463077));
#78145=CARTESIAN_POINT('',(-10.1269675574,-37.2742356128,-7.84083285349));
#78146=CARTESIAN_POINT('Origin',(-11.6189039641,-38.7742356128,-7.89867997696));
#78147=CARTESIAN_POINT('',(-11.6189039641,-37.2742356128,-7.89867997696));
#78148=CARTESIAN_POINT('',(-10.8175627992,-37.2742356128,-7.11751678877));
#78149=CARTESIAN_POINT('',(-11.6189039641,-33.7742356128,-7.89867997696));
#78150=CARTESIAN_POINT('',(-11.6189039641,-35.5242356128,-7.89867997696));
#78151=CARTESIAN_POINT('',(-13.1382272111,-33.7742356128,-9.37974627375));
#78152=CARTESIAN_POINT('',(-12.3785655876,-33.7742356128,-8.63921312536));
#78153=CARTESIAN_POINT('',(-13.1382272111,-37.2742356128,-9.37974627375));
#78154=CARTESIAN_POINT('',(-13.1382272111,-35.5242356128,-9.37974627375));
#78155=CARTESIAN_POINT('',(-12.8689688238,-37.2742356128,-9.11726788193));
#78156=CARTESIAN_POINT('Origin',(-8.33174409695,-38.7742356128,-11.2707494202));
#78157=CARTESIAN_POINT('',(-9.86946476635,-37.2742356128,-12.7697498875));
#78158=CARTESIAN_POINT('',(-9.60206866896,-37.2742356128,-12.5090868927));
#78159=CARTESIAN_POINT('',(-9.86946476635,-33.7742356128,-12.7697498875));
#78160=CARTESIAN_POINT('',(-9.86946476635,-35.5242356128,-12.7697498875));
#78161=CARTESIAN_POINT('',(-8.33174409695,-33.7742356128,-11.2707494202));
#78162=CARTESIAN_POINT('',(-9.10060443165,-33.7742356128,-12.0202496539));
#78163=CARTESIAN_POINT('',(-8.33174409695,-37.2742356128,-11.2707494202));
#78164=CARTESIAN_POINT('',(-8.33174409695,-35.5242356128,-11.2707494202));
#78165=CARTESIAN_POINT('',(-7.34305038686,-37.2742356128,-10.3069512721));
#78166=CARTESIAN_POINT('Origin',(-9.02977805856,-38.7742356128,-10.5546847664));
#78167=CARTESIAN_POINT('',(-9.02977805856,-37.2742356128,-10.5546847664));
#78168=CARTESIAN_POINT('',(-8.12836745794,-37.2742356128,-9.6759719166));
#78169=CARTESIAN_POINT('',(-9.02977805856,-33.7742356128,-10.5546847664));
#78170=CARTESIAN_POINT('',(-9.02977805856,-35.5242356128,-10.5546847664));
#78171=CARTESIAN_POINT('',(-9.91508679725,-33.7742356128,-11.4177012033));
#78172=CARTESIAN_POINT('',(-9.47243242791,-33.7742356128,-10.9861929848));
#78173=CARTESIAN_POINT('',(-9.91508679725,-36.2742356128,-11.4177012033));
#78174=CARTESIAN_POINT('Origin',(9.02977805856,-38.7742356128,-10.5546847664));
#78175=CARTESIAN_POINT('',(9.91508679725,-33.7742356128,-11.4177012033));
#78176=CARTESIAN_POINT('',(9.91508679725,-36.2742356128,-11.4177012033));
#78177=CARTESIAN_POINT('',(9.02977805856,-33.7742356128,-10.5546847664));
#78178=CARTESIAN_POINT('',(9.47243242791,-33.7742356128,-10.9861929848));
#78179=CARTESIAN_POINT('',(9.02977805856,-37.2742356128,-10.5546847664));
#78180=CARTESIAN_POINT('',(9.02977805856,-35.5242356128,-10.5546847664));
#78181=CARTESIAN_POINT('',(8.12836745794,-37.2742356128,-9.6759719166));
#78182=CARTESIAN_POINT('Origin',(8.33174409695,-38.7742356128,-11.2707494202));
#78183=CARTESIAN_POINT('',(8.33174409695,-37.2742356128,-11.2707494202));
#78184=CARTESIAN_POINT('',(7.34305038686,-37.2742356128,-10.3069512721));
#78185=CARTESIAN_POINT('',(8.33174409695,-33.7742356128,-11.2707494202));
#78186=CARTESIAN_POINT('',(8.33174409695,-35.5242356128,-11.2707494202));
#78187=CARTESIAN_POINT('',(9.86946476635,-33.7742356128,-12.7697498875));
#78188=CARTESIAN_POINT('',(9.10060443165,-33.7742356128,-12.0202496539));
#78189=CARTESIAN_POINT('',(9.86946476635,-37.2742356128,-12.7697498875));
#78190=CARTESIAN_POINT('',(9.86946476635,-35.5242356128,-12.7697498875));
#78191=CARTESIAN_POINT('',(9.60206866896,-37.2742356128,-12.5090868927));
#78192=CARTESIAN_POINT('Origin',(11.6189039641,-38.7742356128,-7.89867997696));
#78193=CARTESIAN_POINT('',(13.1382272111,-37.2742356128,-9.37974627375));
#78194=CARTESIAN_POINT('',(12.8689688238,-37.2742356128,-9.11726788193));
#78195=CARTESIAN_POINT('',(13.1382272111,-33.7742356128,-9.37974627375));
#78196=CARTESIAN_POINT('',(13.1382272111,-35.5242356128,-9.37974627375));
#78197=CARTESIAN_POINT('',(11.6189039641,-33.7742356128,-7.89867997696));
#78198=CARTESIAN_POINT('',(12.3785655876,-33.7742356128,-8.63921312536));
#78199=CARTESIAN_POINT('',(11.6189039641,-37.2742356128,-7.89867997696));
#78200=CARTESIAN_POINT('',(11.6189039641,-35.5242356128,-7.89867997696));
#78201=CARTESIAN_POINT('',(10.8175627992,-37.2742356128,-7.11751678877));
#78202=CARTESIAN_POINT('Origin',(10.9208700025,-38.7742356128,-8.61474463077));
#78203=CARTESIAN_POINT('',(10.9208700025,-37.2742356128,-8.61474463077));
#78204=CARTESIAN_POINT('',(10.1269675574,-37.2742356128,-7.84083285349));
#78205=CARTESIAN_POINT('',(10.9208700025,-33.7742356128,-8.61474463077));
#78206=CARTESIAN_POINT('',(10.9208700025,-35.5242356128,-8.61474463077));
#78207=CARTESIAN_POINT('',(11.7961681305,-33.7742356128,-9.46800252678));
#78208=CARTESIAN_POINT('',(11.3585190665,-33.7742356128,-9.04137357878));
#78209=CARTESIAN_POINT('',(11.7961681305,-36.2742356128,-9.46800252678));
#78210=CARTESIAN_POINT('Origin',(-3.35265884719E-30,-37.2742356128,3.15283103411E-22));
#78211=CARTESIAN_POINT('Origin',(12.9288170226,-37.2742356128,-9.5945656699));
#78212=CARTESIAN_POINT('Origin',(-3.35265884719E-30,-37.2742356128,3.15283103411E-22));
#78213=CARTESIAN_POINT('',(13.1382272111,-37.2742356128,9.37974627375));
#78214=CARTESIAN_POINT('',(12.8689688238,-37.2742356128,9.11726788193));
#78215=CARTESIAN_POINT('Origin',(12.9288170226,-37.2742356128,9.5945656699));
#78216=CARTESIAN_POINT('Origin',(-3.35265884719E-30,-37.2742356128,3.15283103411E-22));
#78217=CARTESIAN_POINT('',(8.60554847393,-37.2742356128,-10.560093974));
#78218=CARTESIAN_POINT('Origin',(8.82036787008,-37.2742356128,-10.7695041625));
#78219=CARTESIAN_POINT('',(8.32633488929,-37.2742356128,-10.8465198356));
#78220=CARTESIAN_POINT('',(8.46594168161,-37.2742356128,-10.7033069048));
#78221=CARTESIAN_POINT('Origin',(8.54115428543,-37.2742356128,-11.0559300241));
#78222=CARTESIAN_POINT('Origin',(10.0788749548,-37.2742356128,-12.5549304914));
#78223=CARTESIAN_POINT('Origin',(-10.0788749548,-37.2742356128,-12.5549304914));
#78224=CARTESIAN_POINT('',(-8.32633488929,-37.2742356128,-10.8465198356));
#78225=CARTESIAN_POINT('Origin',(-8.54115428543,-37.2742356128,-11.0559300241));
#78226=CARTESIAN_POINT('',(-8.60554847393,-37.2742356128,-10.560093974));
#78227=CARTESIAN_POINT('',(-8.46594168161,-37.2742356128,-10.7033069048));
#78228=CARTESIAN_POINT('Origin',(-8.82036787008,-37.2742356128,-10.7695041625));
#78229=CARTESIAN_POINT('',(-10.9154607948,-37.2742356128,-8.19051504615));
#78230=CARTESIAN_POINT('Origin',(-11.1302801909,-37.2742356128,-8.39992523463));
#78231=CARTESIAN_POINT('',(-11.1946743794,-37.2742356128,-7.90408918462));
#78232=CARTESIAN_POINT('',(-11.0550675871,-37.2742356128,-8.04730211538));
#78233=CARTESIAN_POINT('Origin',(-11.4094937756,-37.2742356128,-8.1134993731));
#78234=CARTESIAN_POINT('',(-9.4709461123,-37.2742356128,13.0795270061));
#78235=CARTESIAN_POINT('',(-9.19878759701,-37.2742356128,12.8142215122));
#78236=CARTESIAN_POINT('Origin',(-9.68035630078,-37.2742356128,12.8647076099));
#78237=CARTESIAN_POINT('',(9.86946476635,-37.2742356128,12.7697498875));
#78238=CARTESIAN_POINT('Origin',(10.0788749548,-37.2742356128,12.5549304914));
#78239=CARTESIAN_POINT('',(9.60206866896,-37.2742356128,12.5090868927));
#78240=CARTESIAN_POINT('',(11.1946743794,-37.2742356128,-7.90408918462));
#78241=CARTESIAN_POINT('Origin',(11.4094937756,-37.2742356128,-8.1134993731));
#78242=CARTESIAN_POINT('',(10.9154607948,-37.2742356128,-8.19051504615));
#78243=CARTESIAN_POINT('',(11.0550675871,-37.2742356128,-8.04730211538));
#78244=CARTESIAN_POINT('Origin',(11.1302801909,-37.2742356128,-8.39992523463));
#78245=CARTESIAN_POINT('Origin',(-3.35265884719E-30,-37.2742356128,3.15283103411E-22));
#78246=CARTESIAN_POINT('Origin',(-12.9288170226,-37.2742356128,-9.5945656699));
#78247=CARTESIAN_POINT('Origin',(-3.35265884719E-30,-37.2742356128,3.15283103411E-22));
#78248=CARTESIAN_POINT('',(-13.4331612704,-37.2742356128,8.96899284723));
#78249=CARTESIAN_POINT('Origin',(-13.2237510819,-37.2742356128,9.18381224337));
#78250=CARTESIAN_POINT('',(-13.1590062198,-37.2742356128,8.70174109129));
#78251=CARTESIAN_POINT('Origin',(12.1468815993,-33.7742356128,-8.83231958171));
#78252=CARTESIAN_POINT('',(11.4094937756,-33.4742356128,-8.1134993731));
#78253=CARTESIAN_POINT('Origin',(11.4094937756,-33.7742356128,-8.1134993731));
#78254=CARTESIAN_POINT('',(12.9288170226,-33.4742356128,-9.5945656699));
#78255=CARTESIAN_POINT('Origin',(12.9288170226,-33.7742356128,-9.5945656699));
#78256=CARTESIAN_POINT('',(12.1468815993,-33.4742356128,-8.83231958171));
#78257=CARTESIAN_POINT('Origin',(12.9288170226,-36.1242356128,-9.5945656699));
#78258=CARTESIAN_POINT('Origin',(12.9288170226,-33.7742356128,-9.5945656699));
#78259=CARTESIAN_POINT('Origin',(12.9288170226,-33.7742356128,-9.5945656699));
#78260=CARTESIAN_POINT('Origin',(12.9288170226,-33.7742356128,-9.5945656699));
#78261=CARTESIAN_POINT('Origin',(11.4094937756,-36.1242356128,-8.1134993731));
#78262=CARTESIAN_POINT('',(11.1946743794,-33.7742356128,-7.90408918462));
#78263=CARTESIAN_POINT('Origin',(11.4094937756,-33.7742356128,-8.1134993731));
#78264=CARTESIAN_POINT('',(11.1946743794,-36.1242356128,-7.90408918462));
#78265=CARTESIAN_POINT('Origin',(11.4094937756,-33.7742356128,-8.1134993731));
#78266=CARTESIAN_POINT('Origin',(11.4094937756,-33.7742356128,-8.1134993731));
#78267=CARTESIAN_POINT('Origin',(-1.7763568394E-15,-33.7742356128,3.55271399408E-15));
#78268=CARTESIAN_POINT('',(10.0788749548,-33.4742356128,-12.5549304914));
#78269=CARTESIAN_POINT('Origin',(10.0788749548,-33.7742356128,-12.5549304914));
#78270=CARTESIAN_POINT('Origin',(-1.7763568394E-15,-33.4742356128,3.55271399408E-15));
#78271=CARTESIAN_POINT('Origin',(10.0788749548,-36.1242356128,-12.5549304914));
#78272=CARTESIAN_POINT('Origin',(10.0788749548,-33.7742356128,-12.5549304914));
#78273=CARTESIAN_POINT('Origin',(10.0788749548,-33.7742356128,-12.5549304914));
#78274=CARTESIAN_POINT('Origin',(10.0788749548,-33.7742356128,-12.5549304914));
#78275=CARTESIAN_POINT('Origin',(-3.35265884719E-30,-33.4742356128,3.15283103411E-22));
#78276=CARTESIAN_POINT('',(8.54115428543,-33.4742356128,-11.0559300241));
#78277=CARTESIAN_POINT('',(9.31001462013,-33.4742356128,-11.8054302577));
#78278=CARTESIAN_POINT('',(8.82036787008,-33.4742356128,-10.7695041625));
#78279=CARTESIAN_POINT('',(8.68076107776,-33.4742356128,-10.9127170933));
#78280=CARTESIAN_POINT('',(9.70567660877,-33.4742356128,-11.6325205994));
#78281=CARTESIAN_POINT('',(9.26302223942,-33.4742356128,-11.201012381));
#78282=CARTESIAN_POINT('',(10.5267948792,-33.4742356128,-11.6480294286));
#78283=CARTESIAN_POINT('Origin',(10.1244969857,-33.4742356128,-11.2028818071));
#78284=CARTESIAN_POINT('',(12.0471589199,-33.4742356128,-10.0675698139));
#78285=CARTESIAN_POINT('Origin',(-3.35265884719E-30,-33.4742356128,7.1009945507E-16));
#78286=CARTESIAN_POINT('',(12.005578319,-33.4742356128,-9.25318313064));
#78287=CARTESIAN_POINT('Origin',(11.586757942,-33.4742356128,-9.68282192292));
#78288=CARTESIAN_POINT('',(11.1302801909,-33.4742356128,-8.39992523463));
#78289=CARTESIAN_POINT('',(11.567929255,-33.4742356128,-8.82655418263));
#78290=CARTESIAN_POINT('',(11.2698869833,-33.4742356128,-8.25671230387));
#78291=CARTESIAN_POINT('Origin',(9.96422937677,-33.7742356128,-9.59609593478));
#78292=CARTESIAN_POINT('',(10.9154607948,-33.7742356128,-8.19051504615));
#78293=CARTESIAN_POINT('Origin',(11.1302801909,-33.7742356128,-8.39992523463));
#78294=CARTESIAN_POINT('',(9.74940998063,-33.7742356128,-9.38668574629));
#78295=CARTESIAN_POINT('Origin',(11.1302801909,-33.7742356128,-8.39992523463));
#78296=CARTESIAN_POINT('Origin',(11.1302801909,-33.7742356128,-8.39992523463));
#78297=CARTESIAN_POINT('Origin',(11.1302801909,-33.7742356128,-8.39992523463));
#78298=CARTESIAN_POINT('Origin',(9.33228841993,-33.7742356128,-11.8271431975));
#78299=CARTESIAN_POINT('Origin',(8.54115428543,-33.7742356128,-11.0559300241));
#78300=CARTESIAN_POINT('Origin',(8.54115428543,-33.7742356128,-11.0559300241));
#78301=CARTESIAN_POINT('',(8.32633488929,-33.7742356128,-10.8465198356));
#78302=CARTESIAN_POINT('Origin',(8.54115428543,-33.7742356128,-11.0559300241));
#78303=CARTESIAN_POINT('Origin',(8.54115428543,-33.7742356128,-11.0559300241));
#78304=CARTESIAN_POINT('Origin',(9.96422937677,-33.7742356128,-9.59609593478));
#78305=CARTESIAN_POINT('',(8.60554847393,-33.7742356128,-10.560093974));
#78306=CARTESIAN_POINT('',(9.74940998063,-33.7742356128,-9.38668574629));
#78307=CARTESIAN_POINT('Origin',(8.82036787008,-33.7742356128,-10.7695041625));
#78308=CARTESIAN_POINT('Origin',(8.82036787008,-33.7742356128,-10.7695041625));
#78309=CARTESIAN_POINT('Origin',(8.82036787008,-33.7742356128,-10.7695041625));
#78310=CARTESIAN_POINT('Origin',(8.82036787008,-33.7742356128,-10.7695041625));
#78311=CARTESIAN_POINT('Origin',(9.61880743047,-33.7742356128,-11.5478388094));
#78312=CARTESIAN_POINT('Origin',(9.70567660877,-33.7742356128,-11.6325205994));
#78313=CARTESIAN_POINT('Origin',(10.1244969857,-33.7742356128,-11.2028818071));
#78314=CARTESIAN_POINT('Origin',(10.1244969857,-33.7742356128,-11.2028818071));
#78315=CARTESIAN_POINT('Origin',(10.5267948792,-33.7742356128,-11.6480294286));
#78316=CARTESIAN_POINT('Origin',(1.7763568394E-14,-33.7742356128,-1.42108543999E-14));
#78317=CARTESIAN_POINT('Origin',(12.0471589199,-33.7742356128,-10.0675698139));
#78318=CARTESIAN_POINT('Origin',(11.586757942,-33.7742356128,-9.68282192292));
#78319=CARTESIAN_POINT('Origin',(11.586757942,-33.7742356128,-9.68282192292));
#78320=CARTESIAN_POINT('Origin',(12.005578319,-33.7742356128,-9.25318313064));
#78321=CARTESIAN_POINT('Origin',(11.8603625888,-33.7742356128,-9.11162396985));
#78322=CARTESIAN_POINT('Origin',(11.5436913602,-37.2742356128,-7.54605685771));
#78323=CARTESIAN_POINT('',(10.9154607948,-36.1242356128,-8.19051504615));
#78324=CARTESIAN_POINT('Origin',(11.1302801909,-36.1242356128,-8.39992523463));
#78325=CARTESIAN_POINT('Origin',(8.54115428543,-36.1242356128,-11.0559300241));
#78326=CARTESIAN_POINT('',(8.32633488929,-36.1242356128,-10.8465198356));
#78327=CARTESIAN_POINT('Origin',(11.5436913602,-37.2742356128,-7.54605685771));
#78328=CARTESIAN_POINT('',(8.60554847393,-36.1242356128,-10.560093974));
#78329=CARTESIAN_POINT('Origin',(8.82036787008,-36.1242356128,-10.7695041625));
#78330=CARTESIAN_POINT('Origin',(10.1244969857,-36.1242356128,-11.2028818071));
#78331=CARTESIAN_POINT('Origin',(11.586757942,-36.1242356128,-9.68282192292));
#78332=CARTESIAN_POINT('Origin',(7.97371177005,-37.2742356128,10.9217324394));
#78333=CARTESIAN_POINT('',(9.86946476635,-33.7742356128,12.7697498875));
#78334=CARTESIAN_POINT('',(9.86946476635,-36.1242356128,12.7697498875));
#78335=CARTESIAN_POINT('',(8.33174409695,-33.7742356128,11.2707494202));
#78336=CARTESIAN_POINT('',(9.08759374531,-33.7742356128,12.00756658));
#78337=CARTESIAN_POINT('',(8.33174409695,-36.1242356128,11.2707494202));
#78338=CARTESIAN_POINT('Origin',(9.33228841993,-33.7742356128,11.8271431975));
#78339=CARTESIAN_POINT('',(8.54115428543,-33.4742356128,11.0559300241));
#78340=CARTESIAN_POINT('Origin',(8.54115428543,-33.7742356128,11.0559300241));
#78341=CARTESIAN_POINT('',(10.0788749548,-33.4742356128,12.5549304914));
#78342=CARTESIAN_POINT('Origin',(10.0788749548,-33.7742356128,12.5549304914));
#78343=CARTESIAN_POINT('',(9.33228841993,-33.4742356128,11.8271431975));
#78344=CARTESIAN_POINT('Origin',(10.0788749548,-36.1242356128,12.5549304914));
#78345=CARTESIAN_POINT('Origin',(10.0788749548,-33.7742356128,12.5549304914));
#78346=CARTESIAN_POINT('Origin',(10.0788749548,-33.7742356128,12.5549304914));
#78347=CARTESIAN_POINT('Origin',(10.0788749548,-33.7742356128,12.5549304914));
#78348=CARTESIAN_POINT('Origin',(8.54115428543,-36.1242356128,11.0559300241));
#78349=CARTESIAN_POINT('',(8.32633488929,-33.7742356128,10.8465198356));
#78350=CARTESIAN_POINT('',(8.32633488929,-36.1242356128,10.8465198356));
#78351=CARTESIAN_POINT('Origin',(8.54115428543,-33.7742356128,11.0559300241));
#78352=CARTESIAN_POINT('Origin',(8.54115428543,-33.7742356128,11.0559300241));
#78353=CARTESIAN_POINT('Origin',(8.54115428543,-33.7742356128,11.0559300241));
#78354=CARTESIAN_POINT('Origin',(-3.35265884719E-30,-33.7742356128,3.15283103411E-22));
#78355=CARTESIAN_POINT('',(12.9288170226,-33.4742356128,9.5945656699));
#78356=CARTESIAN_POINT('Origin',(12.9288170226,-33.7742356128,9.5945656699));
#78357=CARTESIAN_POINT('Origin',(-3.35265884719E-30,-33.4742356128,3.15283103411E-22));
#78358=CARTESIAN_POINT('Origin',(12.9288170226,-36.1242356128,9.5945656699));
#78359=CARTESIAN_POINT('',(13.1382272111,-33.7742356128,9.37974627375));
#78360=CARTESIAN_POINT('',(13.1382272111,-36.1242356128,9.37974627375));
#78361=CARTESIAN_POINT('Origin',(12.9288170226,-33.7742356128,9.5945656699));
#78362=CARTESIAN_POINT('Origin',(12.9288170226,-33.7742356128,9.5945656699));
#78363=CARTESIAN_POINT('Origin',(12.9288170226,-33.7742356128,9.5945656699));
#78364=CARTESIAN_POINT('Origin',(-3.35265884719E-30,-33.4742356128,3.15283103411E-22));
#78365=CARTESIAN_POINT('',(11.4094937756,-33.4742356128,8.1134993731));
#78366=CARTESIAN_POINT('',(12.1691553991,-33.4742356128,8.8540325215));
#78367=CARTESIAN_POINT('',(11.1302801909,-33.4742356128,8.39992523463));
#78368=CARTESIAN_POINT('',(11.2698869833,-33.4742356128,8.25671230387));
#78369=CARTESIAN_POINT('',(12.005578319,-33.4742356128,9.25318313064));
#78370=CARTESIAN_POINT('',(11.567929255,-33.4742356128,8.82655418263));
#78371=CARTESIAN_POINT('',(12.0471589199,-33.4742356128,10.0675698139));
#78372=CARTESIAN_POINT('Origin',(11.586757942,-33.4742356128,9.68282192292));
#78373=CARTESIAN_POINT('',(10.5267948792,-33.4742356128,11.6480294286));
#78374=CARTESIAN_POINT('Origin',(-3.35265884719E-30,-33.4742356128,7.1009945507E-16));
#78375=CARTESIAN_POINT('',(9.70567660877,-33.4742356128,11.6325205994));
#78376=CARTESIAN_POINT('Origin',(10.1244969857,-33.4742356128,11.2028818071));
#78377=CARTESIAN_POINT('',(8.82036787008,-33.4742356128,10.7695041625));
#78378=CARTESIAN_POINT('',(9.26302223942,-33.4742356128,11.201012381));
#78379=CARTESIAN_POINT('',(8.68076107776,-33.4742356128,10.9127170933));
#78380=CARTESIAN_POINT('Origin',(9.96422937677,-33.7742356128,9.59609593478));
#78381=CARTESIAN_POINT('',(8.60554847393,-33.7742356128,10.560093974));
#78382=CARTESIAN_POINT('Origin',(8.82036787008,-33.7742356128,10.7695041625));
#78383=CARTESIAN_POINT('',(9.74940998063,-33.7742356128,9.38668574629));
#78384=CARTESIAN_POINT('Origin',(8.82036787008,-33.7742356128,10.7695041625));
#78385=CARTESIAN_POINT('',(9.02977805856,-33.7742356128,10.5546847664));
#78386=CARTESIAN_POINT('Origin',(8.82036787008,-33.7742356128,10.7695041625));
#78387=CARTESIAN_POINT('Origin',(8.82036787008,-33.7742356128,10.7695041625));
#78388=CARTESIAN_POINT('Origin',(12.1468815993,-33.7742356128,8.83231958171));
#78389=CARTESIAN_POINT('',(11.6189039641,-33.7742356128,7.89867997696));
#78390=CARTESIAN_POINT('',(12.3562917878,-33.7742356128,8.61750018557));
#78391=CARTESIAN_POINT('Origin',(11.4094937756,-33.7742356128,8.1134993731));
#78392=CARTESIAN_POINT('Origin',(11.4094937756,-33.7742356128,8.1134993731));
#78393=CARTESIAN_POINT('',(11.1946743794,-33.7742356128,7.90408918462));
#78394=CARTESIAN_POINT('Origin',(11.4094937756,-33.7742356128,8.1134993731));
#78395=CARTESIAN_POINT('Origin',(11.4094937756,-33.7742356128,8.1134993731));
#78396=CARTESIAN_POINT('Origin',(9.96422937677,-33.7742356128,9.59609593478));
#78397=CARTESIAN_POINT('',(10.9154607948,-33.7742356128,8.19051504615));
#78398=CARTESIAN_POINT('',(9.74940998063,-33.7742356128,9.38668574629));
#78399=CARTESIAN_POINT('Origin',(11.1302801909,-33.7742356128,8.39992523463));
#78400=CARTESIAN_POINT('Origin',(11.1302801909,-33.7742356128,8.39992523463));
#78401=CARTESIAN_POINT('',(10.9208700025,-33.7742356128,8.61474463077));
#78402=CARTESIAN_POINT('Origin',(11.1302801909,-33.7742356128,8.39992523463));
#78403=CARTESIAN_POINT('Origin',(11.1302801909,-33.7742356128,8.39992523463));
#78404=CARTESIAN_POINT('Origin',(11.8603625888,-33.7742356128,9.11162396985));
#78405=CARTESIAN_POINT('',(11.7961681305,-33.7742356128,9.46800252678));
#78406=CARTESIAN_POINT('',(11.6509524003,-33.7742356128,9.32644336599));
#78407=CARTESIAN_POINT('Origin',(12.005578319,-33.7742356128,9.25318313064));
#78408=CARTESIAN_POINT('Origin',(11.586757942,-33.7742356128,9.68282192292));
#78409=CARTESIAN_POINT('Origin',(11.586757942,-33.7742356128,9.68282192292));
#78410=CARTESIAN_POINT('Origin',(12.0471589199,-33.7742356128,10.0675698139));
#78411=CARTESIAN_POINT('Origin',(1.24344978758E-14,-33.7742356128,1.59872118699E-14));
#78412=CARTESIAN_POINT('Origin',(10.5267948792,-33.7742356128,11.6480294286));
#78413=CARTESIAN_POINT('Origin',(10.1244969857,-33.7742356128,11.2028818071));
#78414=CARTESIAN_POINT('',(9.91508679725,-33.7742356128,11.4177012033));
#78415=CARTESIAN_POINT('Origin',(10.1244969857,-33.7742356128,11.2028818071));
#78416=CARTESIAN_POINT('Origin',(9.70567660877,-33.7742356128,11.6325205994));
#78417=CARTESIAN_POINT('Origin',(9.61880743047,-33.7742356128,11.5478388094));
#78418=CARTESIAN_POINT('',(9.82821761895,-33.7742356128,11.3330194132));
#78419=CARTESIAN_POINT('Origin',(11.5436913602,-37.2742356128,7.54605685771));
#78420=CARTESIAN_POINT('',(8.60554847393,-36.1242356128,10.560093974));
#78421=CARTESIAN_POINT('Origin',(8.82036787008,-36.1242356128,10.7695041625));
#78422=CARTESIAN_POINT('',(9.02977805856,-36.1242356128,10.5546847664));
#78423=CARTESIAN_POINT('Origin',(11.2608716372,-37.2742356128,7.54966299616));
#78424=CARTESIAN_POINT('',(11.6189039641,-36.1242356128,7.89867997696));
#78425=CARTESIAN_POINT('Origin',(11.4094937756,-36.1242356128,8.1134993731));
#78426=CARTESIAN_POINT('',(11.1946743794,-36.1242356128,7.90408918462));
#78427=CARTESIAN_POINT('Origin',(11.5436913602,-37.2742356128,7.54605685771));
#78428=CARTESIAN_POINT('',(10.9154607948,-36.1242356128,8.19051504615));
#78429=CARTESIAN_POINT('Origin',(11.1302801909,-36.1242356128,8.39992523463));
#78430=CARTESIAN_POINT('',(10.9208700025,-36.1242356128,8.61474463077));
#78431=CARTESIAN_POINT('Origin',(10.5628376756,-37.2742356128,8.26572764997));
#78432=CARTESIAN_POINT('',(11.7961681305,-36.1242356128,9.46800252678));
#78433=CARTESIAN_POINT('Origin',(11.586757942,-36.1242356128,9.68282192292));
#78434=CARTESIAN_POINT('Origin',(10.1244969857,-36.1242356128,11.2028818071));
#78435=CARTESIAN_POINT('',(9.91508679725,-36.1242356128,11.4177012033));
#78436=CARTESIAN_POINT('Origin',(8.67174573165,-37.2742356128,10.2056677856));
#78437=CARTESIAN_POINT('Origin',(-12.1468815993,-33.7742356128,-8.83231958171));
#78438=CARTESIAN_POINT('',(-11.4094937756,-33.4742356128,-8.1134993731));
#78439=CARTESIAN_POINT('Origin',(-11.4094937756,-33.7742356128,-8.1134993731));
#78440=CARTESIAN_POINT('',(-12.9288170226,-33.4742356128,-9.5945656699));
#78441=CARTESIAN_POINT('',(-12.1468815993,-33.4742356128,-8.83231958171));
#78442=CARTESIAN_POINT('Origin',(-12.9288170226,-33.7742356128,-9.5945656699));
#78443=CARTESIAN_POINT('Origin',(-12.9288170226,-36.1242356128,-9.5945656699));
#78444=CARTESIAN_POINT('Origin',(-12.9288170226,-33.7742356128,-9.5945656699));
#78445=CARTESIAN_POINT('Origin',(-12.9288170226,-33.7742356128,-9.5945656699));
#78446=CARTESIAN_POINT('Origin',(-12.9288170226,-33.7742356128,-9.5945656699));
#78447=CARTESIAN_POINT('Origin',(-11.4094937756,-36.1242356128,-8.1134993731));
#78448=CARTESIAN_POINT('',(-11.1946743794,-33.7742356128,-7.90408918462));
#78449=CARTESIAN_POINT('',(-11.1946743794,-36.1242356128,-7.90408918462));
#78450=CARTESIAN_POINT('Origin',(-11.4094937756,-33.7742356128,-8.1134993731));
#78451=CARTESIAN_POINT('Origin',(-11.4094937756,-33.7742356128,-8.1134993731));
#78452=CARTESIAN_POINT('Origin',(-11.4094937756,-33.7742356128,-8.1134993731));
#78453=CARTESIAN_POINT('Origin',(-3.35265884719E-30,-33.7742356128,3.55271399408E-15));
#78454=CARTESIAN_POINT('',(-10.0788749548,-33.4742356128,-12.5549304914));
#78455=CARTESIAN_POINT('Origin',(-3.35265884719E-30,-33.4742356128,3.55271399408E-15));
#78456=CARTESIAN_POINT('Origin',(-10.0788749548,-33.7742356128,-12.5549304914));
#78457=CARTESIAN_POINT('Origin',(-10.0788749548,-36.1242356128,-12.5549304914));
#78458=CARTESIAN_POINT('Origin',(-10.0788749548,-33.7742356128,-12.5549304914));
#78459=CARTESIAN_POINT('Origin',(-10.0788749548,-33.7742356128,-12.5549304914));
#78460=CARTESIAN_POINT('Origin',(-10.0788749548,-33.7742356128,-12.5549304914));
#78461=CARTESIAN_POINT('Origin',(-3.35265884719E-30,-33.4742356128,3.15283103411E-22));
#78462=CARTESIAN_POINT('',(-11.1302801909,-33.4742356128,-8.39992523463));
#78463=CARTESIAN_POINT('',(-11.2698869833,-33.4742356128,-8.25671230387));
#78464=CARTESIAN_POINT('',(-12.005578319,-33.4742356128,-9.25318313064));
#78465=CARTESIAN_POINT('',(-11.567929255,-33.4742356128,-8.82655418263));
#78466=CARTESIAN_POINT('',(-12.0471589199,-33.4742356128,-10.0675698139));
#78467=CARTESIAN_POINT('Origin',(-11.586757942,-33.4742356128,-9.68282192292));
#78468=CARTESIAN_POINT('',(-10.5267948792,-33.4742356128,-11.6480294286));
#78469=CARTESIAN_POINT('Origin',(7.10099139787E-16,-33.4742356128,-1.0651483944E-15));
#78470=CARTESIAN_POINT('',(-9.70567660877,-33.4742356128,-11.6325205994));
#78471=CARTESIAN_POINT('Origin',(-10.1244969857,-33.4742356128,-11.2028818071));
#78472=CARTESIAN_POINT('',(-8.82036787008,-33.4742356128,-10.7695041625));
#78473=CARTESIAN_POINT('',(-9.26302223942,-33.4742356128,-11.201012381));
#78474=CARTESIAN_POINT('',(-8.54115428543,-33.4742356128,-11.0559300241));
#78475=CARTESIAN_POINT('',(-8.68076107776,-33.4742356128,-10.9127170933));
#78476=CARTESIAN_POINT('',(-9.31001462013,-33.4742356128,-11.8054302577));
#78477=CARTESIAN_POINT('Origin',(-9.96422937677,-33.7742356128,-9.59609593478));
#78478=CARTESIAN_POINT('',(-10.9154607948,-33.7742356128,-8.19051504615));
#78479=CARTESIAN_POINT('Origin',(-11.1302801909,-33.7742356128,-8.39992523463));
#78480=CARTESIAN_POINT('',(-9.74940998063,-33.7742356128,-9.38668574629));
#78481=CARTESIAN_POINT('Origin',(-11.1302801909,-33.7742356128,-8.39992523463));
#78482=CARTESIAN_POINT('Origin',(-11.1302801909,-33.7742356128,-8.39992523463));
#78483=CARTESIAN_POINT('Origin',(-11.1302801909,-33.7742356128,-8.39992523463));
#78484=CARTESIAN_POINT('Origin',(-9.33228841993,-33.7742356128,-11.8271431975));
#78485=CARTESIAN_POINT('Origin',(-8.54115428543,-33.7742356128,-11.0559300241));
#78486=CARTESIAN_POINT('Origin',(-8.54115428543,-33.7742356128,-11.0559300241));
#78487=CARTESIAN_POINT('',(-8.32633488929,-33.7742356128,-10.8465198356));
#78488=CARTESIAN_POINT('Origin',(-8.54115428543,-33.7742356128,-11.0559300241));
#78489=CARTESIAN_POINT('Origin',(-8.54115428543,-33.7742356128,-11.0559300241));
#78490=CARTESIAN_POINT('Origin',(-9.96422937677,-33.7742356128,-9.59609593478));
#78491=CARTESIAN_POINT('',(-8.60554847393,-33.7742356128,-10.560093974));
#78492=CARTESIAN_POINT('Origin',(-8.82036787008,-33.7742356128,-10.7695041625));
#78493=CARTESIAN_POINT('',(-9.74940998063,-33.7742356128,-9.38668574629));
#78494=CARTESIAN_POINT('Origin',(-8.82036787008,-33.7742356128,-10.7695041625));
#78495=CARTESIAN_POINT('Origin',(-8.82036787008,-33.7742356128,-10.7695041625));
#78496=CARTESIAN_POINT('Origin',(-8.82036787008,-33.7742356128,-10.7695041625));
#78497=CARTESIAN_POINT('Origin',(-9.61880743047,-33.7742356128,-11.5478388094));
#78498=CARTESIAN_POINT('Origin',(-9.70567660877,-33.7742356128,-11.6325205994));
#78499=CARTESIAN_POINT('Origin',(-10.1244969857,-33.7742356128,-11.2028818071));
#78500=CARTESIAN_POINT('Origin',(-10.5267948792,-33.7742356128,-11.6480294286));
#78501=CARTESIAN_POINT('Origin',(-10.1244969857,-33.7742356128,-11.2028818071));
#78502=CARTESIAN_POINT('Origin',(-1.7763568394E-15,-33.7742356128,-3.55271336352E-15));
#78503=CARTESIAN_POINT('Origin',(-12.0471589199,-33.7742356128,-10.0675698139));
#78504=CARTESIAN_POINT('Origin',(-11.586757942,-33.7742356128,-9.68282192292));
#78505=CARTESIAN_POINT('Origin',(-12.005578319,-33.7742356128,-9.25318313064));
#78506=CARTESIAN_POINT('Origin',(-11.586757942,-33.7742356128,-9.68282192292));
#78507=CARTESIAN_POINT('Origin',(-11.8603625888,-33.7742356128,-9.11162396985));
#78508=CARTESIAN_POINT('Origin',(-11.5436913602,-37.2742356128,-7.54605685771));
#78509=CARTESIAN_POINT('',(-10.9154607948,-36.1242356128,-8.19051504615));
#78510=CARTESIAN_POINT('Origin',(-11.1302801909,-36.1242356128,-8.39992523463));
#78511=CARTESIAN_POINT('Origin',(-8.54115428543,-36.1242356128,-11.0559300241));
#78512=CARTESIAN_POINT('',(-8.32633488929,-36.1242356128,-10.8465198356));
#78513=CARTESIAN_POINT('Origin',(-11.5436913602,-37.2742356128,-7.54605685771));
#78514=CARTESIAN_POINT('',(-8.60554847393,-36.1242356128,-10.560093974));
#78515=CARTESIAN_POINT('Origin',(-8.82036787008,-36.1242356128,-10.7695041625));
#78516=CARTESIAN_POINT('Origin',(-10.1244969857,-36.1242356128,-11.2028818071));
#78517=CARTESIAN_POINT('Origin',(-11.586757942,-36.1242356128,-9.68282192292));
#78518=CARTESIAN_POINT('Origin',(-7.62469478924,-37.2742356128,11.2797647663));
#78519=CARTESIAN_POINT('',(-7.98272711615,-33.7742356128,11.6287817471));
#78520=CARTESIAN_POINT('',(-7.98272711615,-36.1242356128,11.6287817471));
#78521=CARTESIAN_POINT('',(-9.4709461123,-33.7742356128,13.0795270061));
#78522=CARTESIAN_POINT('',(-8.71080409351,-33.7742356128,12.3385255589));
#78523=CARTESIAN_POINT('',(-9.4709461123,-36.1242356128,13.0795270061));
#78524=CARTESIAN_POINT('Origin',(-8.96263144028,-33.7742356128,12.165055246));
#78525=CARTESIAN_POINT('',(-8.19213730463,-33.4742356128,11.413962351));
#78526=CARTESIAN_POINT('Origin',(-8.19213730463,-33.7742356128,11.413962351));
#78527=CARTESIAN_POINT('',(-9.68035630078,-33.4742356128,12.8647076099));
#78528=CARTESIAN_POINT('',(-8.96263144028,-33.4742356128,12.165055246));
#78529=CARTESIAN_POINT('Origin',(-9.68035630078,-33.7742356128,12.8647076099));
#78530=CARTESIAN_POINT('Origin',(-8.19213730463,-36.1242356128,11.413962351));
#78531=CARTESIAN_POINT('',(-7.97731790849,-33.7742356128,11.2045521625));
#78532=CARTESIAN_POINT('',(-7.97731790849,-36.1242356128,11.2045521625));
#78533=CARTESIAN_POINT('Origin',(-8.19213730463,-33.7742356128,11.413962351));
#78534=CARTESIAN_POINT('Origin',(-8.19213730463,-33.7742356128,11.413962351));
#78535=CARTESIAN_POINT('Origin',(-8.19213730463,-33.7742356128,11.413962351));
#78536=CARTESIAN_POINT('Origin',(-9.68035630078,-36.1242356128,12.8647076099));
#78537=CARTESIAN_POINT('Origin',(-9.68035630078,-33.7742356128,12.8647076099));
#78538=CARTESIAN_POINT('Origin',(-9.68035630078,-33.7742356128,12.8647076099));
#78539=CARTESIAN_POINT('Origin',(-9.68035630078,-33.7742356128,12.8647076099));
#78540=CARTESIAN_POINT('Origin',(-3.35265884719E-30,-33.4742356128,3.15283103411E-22));
#78541=CARTESIAN_POINT('',(-8.47135088927,-33.4742356128,11.1275364894));
#78542=CARTESIAN_POINT('',(-8.33174409695,-33.4742356128,11.2707494202));
#78543=CARTESIAN_POINT('',(-9.32799888907,-33.4742356128,11.9626138722));
#78544=CARTESIAN_POINT('',(-8.89967488917,-33.4742356128,11.5450751808));
#78545=CARTESIAN_POINT('',(-10.1341100978,-33.4742356128,11.9912389904));
#78546=CARTESIAN_POINT('Origin',(-9.74681926603,-33.4742356128,11.5329750799));
#78547=CARTESIAN_POINT('',(-12.3752654181,-33.4742356128,9.66140806669));
#78548=CARTESIAN_POINT('Origin',(7.10099139787E-16,-33.4742356128,-1.0651483944E-15));
#78549=CARTESIAN_POINT('',(-12.3211457154,-33.4742356128,8.86254348841));
#78550=CARTESIAN_POINT('Origin',(-11.9023253384,-33.4742356128,9.2921822807));
#78551=CARTESIAN_POINT('',(-11.4792971717,-33.4742356128,8.04189290772));
#78552=CARTESIAN_POINT('',(-11.9002214436,-33.4742356128,8.45221819807));
#78553=CARTESIAN_POINT('',(-11.7585107564,-33.4742356128,7.7554670462));
#78554=CARTESIAN_POINT('',(-11.6189039641,-33.4742356128,7.89867997696));
#78555=CARTESIAN_POINT('',(-13.2237510819,-33.4742356128,9.18381224337));
#78556=CARTESIAN_POINT('',(-12.4911309192,-33.4742356128,8.46963964479));
#78557=CARTESIAN_POINT('Origin',(1.01287953956E-15,-33.4742356128,-6.7525271109E-16));
#78558=CARTESIAN_POINT('Origin',(-9.96493365594,-33.7742356128,9.5953734636));
#78559=CARTESIAN_POINT('',(-8.25653149313,-33.7742356128,10.918126301));
#78560=CARTESIAN_POINT('Origin',(-8.47135088927,-33.7742356128,11.1275364894));
#78561=CARTESIAN_POINT('',(-9.7501142598,-33.7742356128,9.38596327512));
#78562=CARTESIAN_POINT('Origin',(-8.47135088927,-33.7742356128,11.1275364894));
#78563=CARTESIAN_POINT('',(-8.68076107776,-33.7742356128,10.9127170933));
#78564=CARTESIAN_POINT('Origin',(-8.47135088927,-33.7742356128,11.1275364894));
#78565=CARTESIAN_POINT('Origin',(-8.47135088927,-33.7742356128,11.1275364894));
#78566=CARTESIAN_POINT('Origin',(3.5527136788E-15,-33.7742356128,-1.77635652412E-15));
#78567=CARTESIAN_POINT('Origin',(-13.2237510819,-33.7742356128,9.18381224337));
#78568=CARTESIAN_POINT('Origin',(-13.2237510819,-33.7742356128,9.18381224337));
#78569=CARTESIAN_POINT('',(-13.4331612704,-33.7742356128,8.96899284723));
#78570=CARTESIAN_POINT('Origin',(-13.2237510819,-33.7742356128,9.18381224337));
#78571=CARTESIAN_POINT('Origin',(-13.2237510819,-33.7742356128,9.18381224337));
#78572=CARTESIAN_POINT('Origin',(-9.96493365594,-33.7742356128,9.5953734636));
#78573=CARTESIAN_POINT('',(-11.5436913602,-33.7742356128,7.54605685771));
#78574=CARTESIAN_POINT('Origin',(-11.7585107564,-33.7742356128,7.7554670462));
#78575=CARTESIAN_POINT('',(-11.2644777756,-33.7742356128,7.83248271924));
#78576=CARTESIAN_POINT('Origin',(-11.4792971717,-33.7742356128,8.04189290772));
#78577=CARTESIAN_POINT('',(-9.7501142598,-33.7742356128,9.38596327512));
#78578=CARTESIAN_POINT('Origin',(-11.7585107564,-33.7742356128,7.7554670462));
#78579=CARTESIAN_POINT('',(-11.9679209449,-33.7742356128,7.54064765005));
#78580=CARTESIAN_POINT('Origin',(-11.7585107564,-33.7742356128,7.7554670462));
#78581=CARTESIAN_POINT('Origin',(-11.7585107564,-33.7742356128,7.7554670462));
#78582=CARTESIAN_POINT('Origin',(-11.4792971717,-33.7742356128,8.04189290772));
#78583=CARTESIAN_POINT('',(-11.2698869833,-33.7742356128,8.25671230387));
#78584=CARTESIAN_POINT('Origin',(-11.4792971717,-33.7742356128,8.04189290772));
#78585=CARTESIAN_POINT('Origin',(-11.4792971717,-33.7742356128,8.04189290772));
#78586=CARTESIAN_POINT('Origin',(-12.4647462816,-33.7742356128,8.44391937918));
#78587=CARTESIAN_POINT('',(-12.6741564701,-33.7742356128,8.22909998303));
#78588=CARTESIAN_POINT('Origin',(-12.1782272711,-33.7742356128,8.72322376731));
#78589=CARTESIAN_POINT('',(-12.1117355269,-33.7742356128,9.07736288456));
#78590=CARTESIAN_POINT('Origin',(-12.3211457154,-33.7742356128,8.86254348841));
#78591=CARTESIAN_POINT('',(-11.9688170826,-33.7742356128,8.93804316346));
#78592=CARTESIAN_POINT('Origin',(-11.9023253384,-33.7742356128,9.2921822807));
#78593=CARTESIAN_POINT('Origin',(-12.3752654181,-33.7742356128,9.66140806669));
#78594=CARTESIAN_POINT('Origin',(-11.9023253384,-33.7742356128,9.2921822807));
#78595=CARTESIAN_POINT('Origin',(1.7763568394E-15,-33.7742356128,-1.77635652412E-15));
#78596=CARTESIAN_POINT('Origin',(-10.1341100978,-33.7742356128,11.9912389904));
#78597=CARTESIAN_POINT('Origin',(-9.74681926603,-33.7742356128,11.5329750799));
#78598=CARTESIAN_POINT('',(-9.53740907755,-33.7742356128,11.7477944761));
#78599=CARTESIAN_POINT('Origin',(-9.32799888907,-33.7742356128,11.9626138722));
#78600=CARTESIAN_POINT('Origin',(-9.74681926603,-33.7742356128,11.5329750799));
#78601=CARTESIAN_POINT('Origin',(-9.24915045081,-33.7742356128,11.8857508579));
#78602=CARTESIAN_POINT('',(-9.45856063929,-33.7742356128,11.6709314618));
#78603=CARTESIAN_POINT('Origin',(-11.5436913602,-37.2742356128,7.54605685771));
#78604=CARTESIAN_POINT('',(-8.25653149313,-36.1242356128,10.918126301));
#78605=CARTESIAN_POINT('Origin',(-8.47135088927,-36.1242356128,11.1275364894));
#78606=CARTESIAN_POINT('',(-8.68076107776,-36.1242356128,10.9127170933));
#78607=CARTESIAN_POINT('Origin',(-13.2237510819,-36.1242356128,9.18381224337));
#78608=CARTESIAN_POINT('',(-13.4331612704,-36.1242356128,8.96899284723));
#78609=CARTESIAN_POINT('Origin',(-11.5436913602,-37.2742356128,7.54605685771));
#78610=CARTESIAN_POINT('',(-11.2644777756,-36.1242356128,7.83248271924));
#78611=CARTESIAN_POINT('',(-11.5436913602,-36.1242356128,7.54605685771));
#78612=CARTESIAN_POINT('Origin',(-11.7585107564,-36.1242356128,7.7554670462));
#78613=CARTESIAN_POINT('',(-11.9679209449,-36.1242356128,7.54064765005));
#78614=CARTESIAN_POINT('Origin',(-11.4792971717,-36.1242356128,8.04189290772));
#78615=CARTESIAN_POINT('',(-11.2698869833,-36.1242356128,8.25671230387));
#78616=CARTESIAN_POINT('Origin',(-11.609888618,-37.2742356128,7.19163066925));
#78617=CARTESIAN_POINT('Origin',(-10.9118546564,-37.2742356128,7.90769532306));
#78618=CARTESIAN_POINT('',(-12.1117355269,-36.1242356128,9.07736288456));
#78619=CARTESIAN_POINT('Origin',(-11.9023253384,-36.1242356128,9.2921822807));
#78620=CARTESIAN_POINT('Origin',(-9.74681926603,-36.1242356128,11.5329750799));
#78621=CARTESIAN_POINT('',(-9.53740907755,-36.1242356128,11.7477944761));
#78622=CARTESIAN_POINT('Origin',(-8.32272875085,-37.2742356128,10.5637001125));
#98284=UNCERTAINTY_MEASURE_WITH_UNIT(LENGTH_MEASURE(0.01),#98303,
'DISTANCE_ACCURACY_VALUE',
'Maximum model space distance between geometric entities at asserted c
onnectivities');
#98290=UNCERTAINTY_MEASURE_WITH_UNIT(LENGTH_MEASURE(0.01),#98303,
'DISTANCE_ACCURACY_VALUE',
'Maximum model space distance between geometric entities at asserted c
onnectivities');
#98296=(
GEOMETRIC_REPRESENTATION_CONTEXT(3)
GLOBAL_UNCERTAINTY_ASSIGNED_CONTEXT((#98284))
GLOBAL_UNIT_ASSIGNED_CONTEXT((#98303,#98305,#98306))
REPRESENTATION_CONTEXT('','3D')
);
#98302=(
GEOMETRIC_REPRESENTATION_CONTEXT(3)
GLOBAL_UNCERTAINTY_ASSIGNED_CONTEXT((#98290))
GLOBAL_UNIT_ASSIGNED_CONTEXT((#98303,#98305,#98306))
REPRESENTATION_CONTEXT('','3D')
);
#98303=(
LENGTH_UNIT()
NAMED_UNIT(*)
SI_UNIT(.MILLI.,.METRE.)
);
#98305=(
NAMED_UNIT(*)
PLANE_ANGLE_UNIT()
SI_UNIT($,.RADIAN.)
);
#98306=(
NAMED_UNIT(*)
SI_UNIT($,.STERADIAN.)
SOLID_ANGLE_UNIT()
);
#98312=SHAPE_DEFINITION_REPRESENTATION(#98323,#98344);
#98323=PRODUCT_DEFINITION_SHAPE('',$,#98356);
#98344=SHAPE_REPRESENTATION('',(#34962),#98296);
#98350=PRODUCT_DEFINITION_CONTEXT('part definition',#98385,'design');
#98356=PRODUCT_DEFINITION('Bottom Base','Bottom Base',#98367,#98350);
#98367=PRODUCT_DEFINITION_FORMATION('',$,#98392);
#98385=APPLICATION_CONTEXT(
'Core Data for Automotive Mechanical Design Process');
#98386=PRODUCT_CONTEXT('part definition',#98385,'mechanical');
#98392=PRODUCT('Bottom Base','Bottom Base',$,(#98386));
#98399=PRESENTATION_STYLE_ASSIGNMENT((#98401));
#98401=SURFACE_STYLE_USAGE(.BOTH.,#98403);
#98403=SURFACE_SIDE_STYLE('',(#98405));
#98405=SURFACE_STYLE_FILL_AREA(#98407);
#98407=FILL_AREA_STYLE('Opaque(202,209,238)',(#98409));
#98409=FILL_AREA_STYLE_COLOUR('Opaque(202,209,238)',#98411);
#98411=COLOUR_RGB('Opaque(202,209,238)', 0.31764706, 0.68627451, 0.89019608);
ENDSEC;
END-ISO-10303-21;
